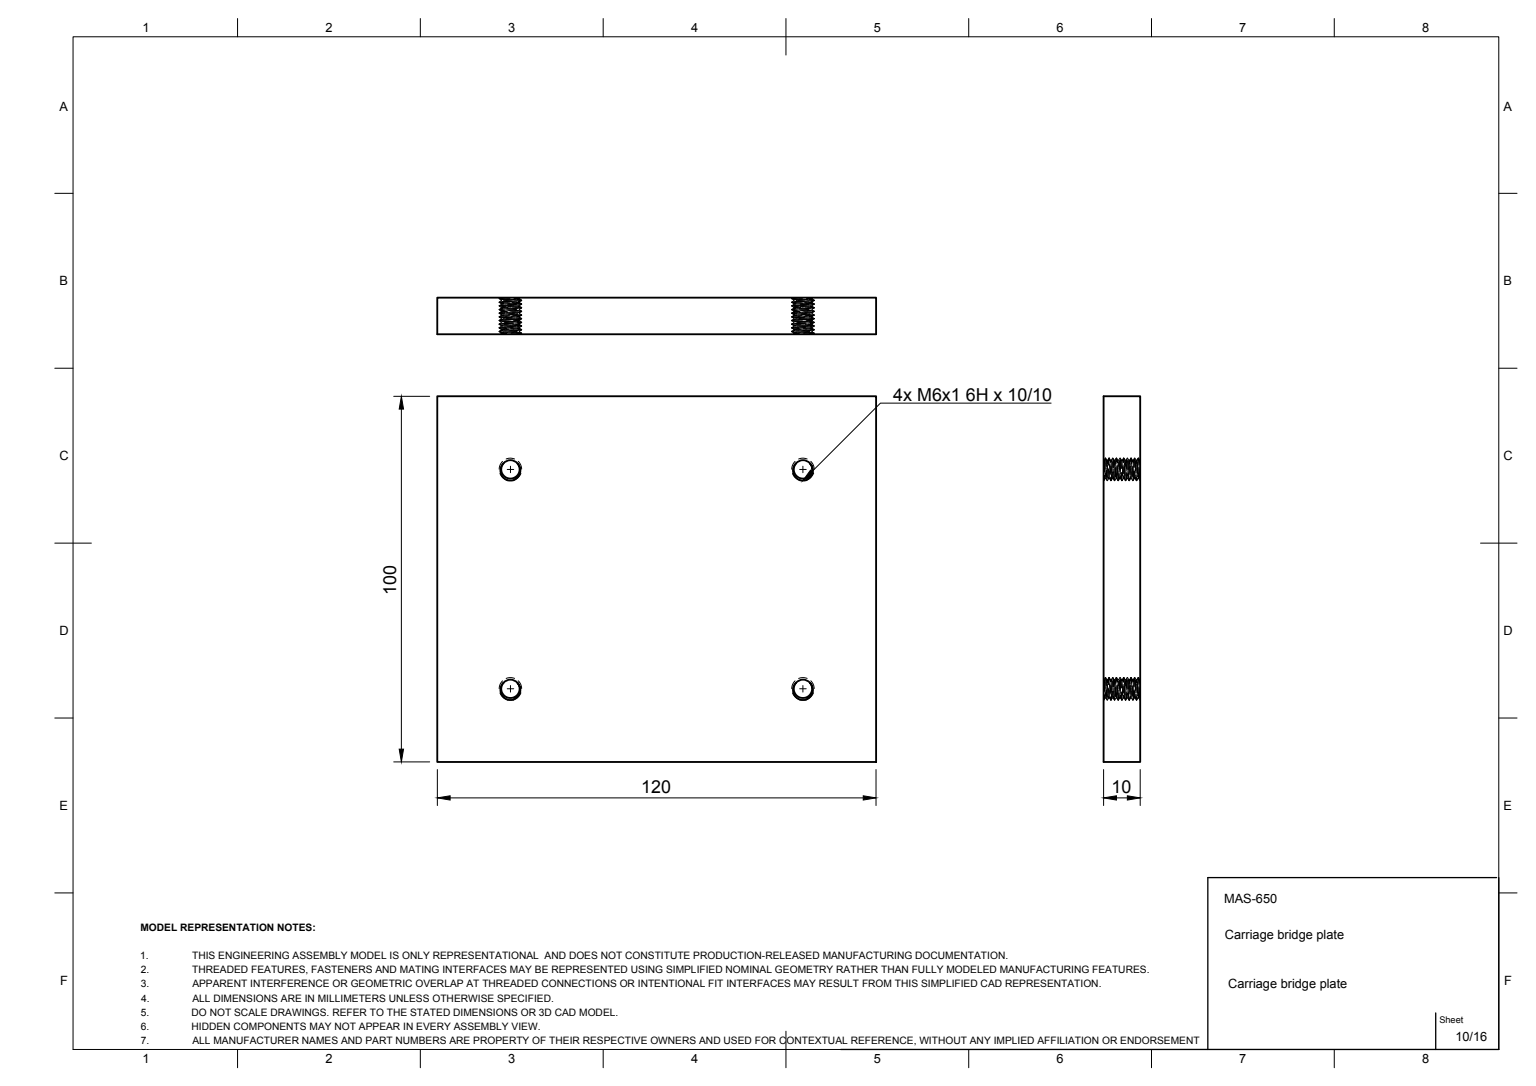
ISO-10303-21;
HEADER;
/* Generated by software containing ST-Developer
 * from STEP Tools, Inc. (www.steptools.com) 
 */

FILE_DESCRIPTION(
/* description */ ('Independent manual traversing gantry with native reusable aluminum pr
ofiles,180mm captured carriage travel, four bronze-bushed rollers, lin
ked ideal rolling motion, bonded acetal lateral guides, positive welde
d end stops and fully retained axle stacks. Editable native profile cu
t lengths220/400mm. Tool attachments viaM6 bridge-plate taps; mounted 
tool outside assembly. Welds, anchors, adhesives, fits, traction, load
/speed/structural/life ratings unassigned.'),
/* implementation_level */ '2;1');

FILE_NAME(
/* name */ 'Carriage bridge plate.step',
/* time_stamp */ '2026-11-09T20:04:38-08:00',
/* author */ (''),
/* organization */ (''),
/* preprocessor_version */ 'ST-DEVELOPER v20.2',
/* originating_system */ 'Autodesk Translation Framework v15.17.0.0',
/* authorisation */ '');

FILE_SCHEMA (('AUTOMOTIVE_DESIGN { 1 0 10303 214 3 1 1 }'));
ENDSEC;

DATA;
#10=MECHANICAL_DESIGN_GEOMETRIC_PRESENTATION_REPRESENTATION('',(#478),#13231);
#239=B_SPLINE_SURFACE_WITH_KNOTS('',3,3,((#8992,#8993,#8994,#8995,#8996,
#8997,#8998,#8999,#9000,#9001,#9002,#9003,#9004,#9005,#9006,#9007,#9008,
#9009,#9010,#9011,#9012,#9013,#9014,#9015,#9016,#9017,#9018,#9019,#9020,
#9021,#9022,#9023,#9024,#9025,#9026,#9027,#9028,#9029,#9030,#9031,#9032,
#9033,#9034,#9035,#9036,#9037,#9038,#9039,#9040,#9041,#9042,#9043,#9044,
#9045,#9046,#9047,#9048,#9049,#9050,#9051,#9052,#9053,#9054,#9055,#9056,
#9057,#9058,#9059),(#9060,#9061,#9062,#9063,#9064,#9065,#9066,#9067,#9068,
#9069,#9070,#9071,#9072,#9073,#9074,#9075,#9076,#9077,#9078,#9079,#9080,
#9081,#9082,#9083,#9084,#9085,#9086,#9087,#9088,#9089,#9090,#9091,#9092,
#9093,#9094,#9095,#9096,#9097,#9098,#9099,#9100,#9101,#9102,#9103,#9104,
#9105,#9106,#9107,#9108,#9109,#9110,#9111,#9112,#9113,#9114,#9115,#9116,
#9117,#9118,#9119,#9120,#9121,#9122,#9123,#9124,#9125,#9126,#9127),(#9128,
#9129,#9130,#9131,#9132,#9133,#9134,#9135,#9136,#9137,#9138,#9139,#9140,
#9141,#9142,#9143,#9144,#9145,#9146,#9147,#9148,#9149,#9150,#9151,#9152,
#9153,#9154,#9155,#9156,#9157,#9158,#9159,#9160,#9161,#9162,#9163,#9164,
#9165,#9166,#9167,#9168,#9169,#9170,#9171,#9172,#9173,#9174,#9175,#9176,
#9177,#9178,#9179,#9180,#9181,#9182,#9183,#9184,#9185,#9186,#9187,#9188,
#9189,#9190,#9191,#9192,#9193,#9194,#9195),(#9196,#9197,#9198,#9199,#9200,
#9201,#9202,#9203,#9204,#9205,#9206,#9207,#9208,#9209,#9210,#9211,#9212,
#9213,#9214,#9215,#9216,#9217,#9218,#9219,#9220,#9221,#9222,#9223,#9224,
#9225,#9226,#9227,#9228,#9229,#9230,#9231,#9232,#9233,#9234,#9235,#9236,
#9237,#9238,#9239,#9240,#9241,#9242,#9243,#9244,#9245,#9246,#9247,#9248,
#9249,#9250,#9251,#9252,#9253,#9254,#9255,#9256,#9257,#9258,#9259,#9260,
#9261,#9262,#9263)),.UNSPECIFIED.,.F.,.F.,.F.,(4,4),(4,1,1,1,1,1,1,1,1,
1,1,1,1,1,1,1,1,1,1,1,1,1,1,1,1,1,1,1,1,1,1,1,1,1,1,1,1,1,1,1,1,1,1,1,1,
1,1,1,1,1,1,1,1,1,1,1,1,1,1,1,1,1,1,1,1,4),(0.,0.0642013499338865),(11.8589888623078,
12.8566626771512,13.8543364919947,14.8520103068381,15.8496841216816,16.8473579365251,
17.8450317513685,18.842705566212,19.8403793810554,20.8380531958989,21.8357270107423,
22.8334008255858,23.8310746404292,24.8287484552727,25.8264222701161,26.8240960849596,
27.821769899803,28.8194437146465,29.8171175294899,30.8147913443334,31.8124651591768,
32.8101389740203,33.8078127888637,34.8054866037072,35.8031604185506,36.8008342333941,
37.7985080482375,38.796181863081,39.7938556779244,40.7915294927679,41.7892033076113,
42.7868771224548,43.7845509372982,44.7822247521417,45.7798985669851,46.7775723818286,
47.775246196672,48.7729200115155,49.7705938263589,50.7682676412024,51.7659414560458,
52.7636152708893,53.7612890857327,54.7589629005762,55.7566367154196,56.7543105302631,
57.7519843451065,58.74965815995,59.7473319747934,60.7450057896369,61.7426796044803,
62.7403534193238,63.7380272341672,64.7357010490107,65.7333748638542,66.7310486786976,
67.728722493541,68.7263963083845,69.7240701232279,70.7217439380714,71.7194177529149,
72.7170915677583,73.7147653826018,74.7124391974452,75.7101130122887,76.7077868271321),
 .UNSPECIFIED.);
#240=B_SPLINE_SURFACE_WITH_KNOTS('',3,3,((#9480,#9481,#9482,#9483,#9484,
#9485,#9486,#9487,#9488,#9489,#9490,#9491,#9492,#9493,#9494,#9495,#9496,
#9497,#9498,#9499,#9500,#9501,#9502,#9503,#9504,#9505,#9506,#9507,#9508,
#9509,#9510,#9511,#9512,#9513,#9514,#9515,#9516,#9517,#9518,#9519,#9520,
#9521,#9522,#9523,#9524,#9525,#9526,#9527,#9528,#9529,#9530,#9531,#9532,
#9533,#9534,#9535,#9536,#9537,#9538,#9539,#9540,#9541,#9542,#9543,#9544,
#9545,#9546,#9547),(#9548,#9549,#9550,#9551,#9552,#9553,#9554,#9555,#9556,
#9557,#9558,#9559,#9560,#9561,#9562,#9563,#9564,#9565,#9566,#9567,#9568,
#9569,#9570,#9571,#9572,#9573,#9574,#9575,#9576,#9577,#9578,#9579,#9580,
#9581,#9582,#9583,#9584,#9585,#9586,#9587,#9588,#9589,#9590,#9591,#9592,
#9593,#9594,#9595,#9596,#9597,#9598,#9599,#9600,#9601,#9602,#9603,#9604,
#9605,#9606,#9607,#9608,#9609,#9610,#9611,#9612,#9613,#9614,#9615),(#9616,
#9617,#9618,#9619,#9620,#9621,#9622,#9623,#9624,#9625,#9626,#9627,#9628,
#9629,#9630,#9631,#9632,#9633,#9634,#9635,#9636,#9637,#9638,#9639,#9640,
#9641,#9642,#9643,#9644,#9645,#9646,#9647,#9648,#9649,#9650,#9651,#9652,
#9653,#9654,#9655,#9656,#9657,#9658,#9659,#9660,#9661,#9662,#9663,#9664,
#9665,#9666,#9667,#9668,#9669,#9670,#9671,#9672,#9673,#9674,#9675,#9676,
#9677,#9678,#9679,#9680,#9681,#9682,#9683),(#9684,#9685,#9686,#9687,#9688,
#9689,#9690,#9691,#9692,#9693,#9694,#9695,#9696,#9697,#9698,#9699,#9700,
#9701,#9702,#9703,#9704,#9705,#9706,#9707,#9708,#9709,#9710,#9711,#9712,
#9713,#9714,#9715,#9716,#9717,#9718,#9719,#9720,#9721,#9722,#9723,#9724,
#9725,#9726,#9727,#9728,#9729,#9730,#9731,#9732,#9733,#9734,#9735,#9736,
#9737,#9738,#9739,#9740,#9741,#9742,#9743,#9744,#9745,#9746,#9747,#9748,
#9749,#9750,#9751)),.UNSPECIFIED.,.F.,.F.,.F.,(4,4),(4,1,1,1,1,1,1,1,1,
1,1,1,1,1,1,1,1,1,1,1,1,1,1,1,1,1,1,1,1,1,1,1,1,1,1,1,1,1,1,1,1,1,1,1,1,
1,1,1,1,1,1,1,1,1,1,1,1,1,1,1,1,1,1,1,1,4),(0.,0.0642013499338865),(14.3984001269718,
15.3960739418153,16.3937477566587,17.3914215715022,18.3890953863456,19.3867692011891,
20.3844430160325,21.382116830876,22.3797906457194,23.3774644605629,24.3751382754063,
25.3728120902498,26.3704859050932,27.3681597199367,28.3658335347801,29.3635073496236,
30.361181164467,31.3588549793105,32.3565287941539,33.3542026089974,34.3518764238408,
35.3495502386843,36.3472240535278,37.3448978683712,38.3425716832147,39.3402454980581,
40.3379193129016,41.335593127745,42.3332669425885,43.3309407574319,44.3286145722754,
45.3262883871188,46.3239622019623,47.3216360168057,48.3193098316492,49.3169836464926,
50.3146574613361,51.3123312761795,52.310005091023,53.3076789058664,54.3053527207099,
55.3030265355533,56.3007003503968,57.2983741652402,58.2960479800837,59.2937217949271,
60.2913956097706,61.289069424614,62.2867432394575,63.2844170543009,64.2820908691444,
65.2797646839878,66.2774384988313,67.2751123136747,68.2727861285182,69.2704599433616,
70.2681337582051,71.2658075730485,72.263481387892,73.2611552027354,74.2588290175789,
75.2565028324223,76.2541766472658,77.2518504621092,78.2495242769527,79.2471980917962),
 .UNSPECIFIED.);
#241=B_SPLINE_SURFACE_WITH_KNOTS('',3,3,((#10569,#10570,#10571,#10572,#10573,
#10574,#10575,#10576,#10577,#10578,#10579,#10580,#10581,#10582,#10583,#10584,
#10585,#10586,#10587,#10588,#10589,#10590,#10591,#10592,#10593,#10594,#10595,
#10596,#10597,#10598,#10599,#10600,#10601,#10602,#10603,#10604,#10605,#10606,
#10607,#10608,#10609,#10610,#10611,#10612,#10613,#10614,#10615,#10616,#10617,
#10618,#10619,#10620,#10621,#10622,#10623,#10624,#10625,#10626,#10627,#10628,
#10629,#10630,#10631,#10632,#10633,#10634,#10635,#10636),(#10637,#10638,
#10639,#10640,#10641,#10642,#10643,#10644,#10645,#10646,#10647,#10648,#10649,
#10650,#10651,#10652,#10653,#10654,#10655,#10656,#10657,#10658,#10659,#10660,
#10661,#10662,#10663,#10664,#10665,#10666,#10667,#10668,#10669,#10670,#10671,
#10672,#10673,#10674,#10675,#10676,#10677,#10678,#10679,#10680,#10681,#10682,
#10683,#10684,#10685,#10686,#10687,#10688,#10689,#10690,#10691,#10692,#10693,
#10694,#10695,#10696,#10697,#10698,#10699,#10700,#10701,#10702,#10703,#10704),
(#10705,#10706,#10707,#10708,#10709,#10710,#10711,#10712,#10713,#10714,
#10715,#10716,#10717,#10718,#10719,#10720,#10721,#10722,#10723,#10724,#10725,
#10726,#10727,#10728,#10729,#10730,#10731,#10732,#10733,#10734,#10735,#10736,
#10737,#10738,#10739,#10740,#10741,#10742,#10743,#10744,#10745,#10746,#10747,
#10748,#10749,#10750,#10751,#10752,#10753,#10754,#10755,#10756,#10757,#10758,
#10759,#10760,#10761,#10762,#10763,#10764,#10765,#10766,#10767,#10768,#10769,
#10770,#10771,#10772),(#10773,#10774,#10775,#10776,#10777,#10778,#10779,
#10780,#10781,#10782,#10783,#10784,#10785,#10786,#10787,#10788,#10789,#10790,
#10791,#10792,#10793,#10794,#10795,#10796,#10797,#10798,#10799,#10800,#10801,
#10802,#10803,#10804,#10805,#10806,#10807,#10808,#10809,#10810,#10811,#10812,
#10813,#10814,#10815,#10816,#10817,#10818,#10819,#10820,#10821,#10822,#10823,
#10824,#10825,#10826,#10827,#10828,#10829,#10830,#10831,#10832,#10833,#10834,
#10835,#10836,#10837,#10838,#10839,#10840)),.UNSPECIFIED.,.F.,.F.,.F.,(4,
4),(4,1,1,1,1,1,1,1,1,1,1,1,1,1,1,1,1,1,1,1,1,1,1,1,1,1,1,1,1,1,1,1,1,1,
1,1,1,1,1,1,1,1,1,1,1,1,1,1,1,1,1,1,1,1,1,1,1,1,1,1,1,1,1,1,1,4),(0.,0.0642013499338865),
(11.8589888623078,12.8566626771512,13.8543364919947,14.8520103068381,15.8496841216816,
16.847357936525,17.8450317513685,18.8427055662119,19.8403793810554,20.8380531958989,
21.8357270107423,22.8334008255858,23.8310746404292,24.8287484552727,25.8264222701161,
26.8240960849596,27.821769899803,28.8194437146465,29.8171175294899,30.8147913443334,
31.8124651591768,32.8101389740203,33.8078127888637,34.8054866037072,35.8031604185506,
36.8008342333941,37.7985080482375,38.796181863081,39.7938556779244,40.7915294927679,
41.7892033076113,42.7868771224548,43.7845509372982,44.7822247521417,45.7798985669851,
46.7775723818286,47.775246196672,48.7729200115155,49.7705938263589,50.7682676412024,
51.7659414560458,52.7636152708893,53.7612890857327,54.7589629005762,55.7566367154196,
56.7543105302631,57.7519843451065,58.74965815995,59.7473319747934,60.7450057896369,
61.7426796044803,62.7403534193238,63.7380272341672,64.7357010490107,65.7333748638542,
66.7310486786976,67.728722493541,68.7263963083845,69.7240701232279,70.7217439380714,
71.7194177529149,72.7170915677583,73.7147653826018,74.7124391974452,75.7101130122887,
76.7077868271321),.UNSPECIFIED.);
#242=B_SPLINE_SURFACE_WITH_KNOTS('',3,3,((#10960,#10961,#10962,#10963,#10964,
#10965,#10966,#10967,#10968,#10969,#10970,#10971,#10972,#10973,#10974,#10975,
#10976,#10977,#10978,#10979,#10980,#10981,#10982,#10983,#10984,#10985,#10986,
#10987,#10988,#10989,#10990,#10991,#10992,#10993,#10994,#10995,#10996,#10997,
#10998,#10999,#11000,#11001,#11002,#11003,#11004,#11005,#11006,#11007,#11008,
#11009,#11010,#11011,#11012,#11013,#11014,#11015,#11016,#11017,#11018,#11019,
#11020,#11021,#11022,#11023,#11024,#11025,#11026,#11027),(#11028,#11029,
#11030,#11031,#11032,#11033,#11034,#11035,#11036,#11037,#11038,#11039,#11040,
#11041,#11042,#11043,#11044,#11045,#11046,#11047,#11048,#11049,#11050,#11051,
#11052,#11053,#11054,#11055,#11056,#11057,#11058,#11059,#11060,#11061,#11062,
#11063,#11064,#11065,#11066,#11067,#11068,#11069,#11070,#11071,#11072,#11073,
#11074,#11075,#11076,#11077,#11078,#11079,#11080,#11081,#11082,#11083,#11084,
#11085,#11086,#11087,#11088,#11089,#11090,#11091,#11092,#11093,#11094,#11095),
(#11096,#11097,#11098,#11099,#11100,#11101,#11102,#11103,#11104,#11105,
#11106,#11107,#11108,#11109,#11110,#11111,#11112,#11113,#11114,#11115,#11116,
#11117,#11118,#11119,#11120,#11121,#11122,#11123,#11124,#11125,#11126,#11127,
#11128,#11129,#11130,#11131,#11132,#11133,#11134,#11135,#11136,#11137,#11138,
#11139,#11140,#11141,#11142,#11143,#11144,#11145,#11146,#11147,#11148,#11149,
#11150,#11151,#11152,#11153,#11154,#11155,#11156,#11157,#11158,#11159,#11160,
#11161,#11162,#11163),(#11164,#11165,#11166,#11167,#11168,#11169,#11170,
#11171,#11172,#11173,#11174,#11175,#11176,#11177,#11178,#11179,#11180,#11181,
#11182,#11183,#11184,#11185,#11186,#11187,#11188,#11189,#11190,#11191,#11192,
#11193,#11194,#11195,#11196,#11197,#11198,#11199,#11200,#11201,#11202,#11203,
#11204,#11205,#11206,#11207,#11208,#11209,#11210,#11211,#11212,#11213,#11214,
#11215,#11216,#11217,#11218,#11219,#11220,#11221,#11222,#11223,#11224,#11225,
#11226,#11227,#11228,#11229,#11230,#11231)),.UNSPECIFIED.,.F.,.F.,.F.,(4,
4),(4,1,1,1,1,1,1,1,1,1,1,1,1,1,1,1,1,1,1,1,1,1,1,1,1,1,1,1,1,1,1,1,1,1,
1,1,1,1,1,1,1,1,1,1,1,1,1,1,1,1,1,1,1,1,1,1,1,1,1,1,1,1,1,1,1,4),(0.,0.0642013499338865),
(14.3984001269718,15.3960739418153,16.3937477566587,17.3914215715022,18.3890953863456,
19.3867692011891,20.3844430160325,21.382116830876,22.3797906457194,23.3774644605629,
24.3751382754063,25.3728120902498,26.3704859050932,27.3681597199367,28.3658335347801,
29.3635073496236,30.361181164467,31.3588549793105,32.3565287941539,33.3542026089974,
34.3518764238408,35.3495502386843,36.3472240535278,37.3448978683712,38.3425716832147,
39.3402454980581,40.3379193129016,41.335593127745,42.3332669425885,43.3309407574319,
44.3286145722754,45.3262883871188,46.3239622019623,47.3216360168057,48.3193098316492,
49.3169836464926,50.3146574613361,51.3123312761795,52.310005091023,53.3076789058664,
54.3053527207099,55.3030265355533,56.3007003503968,57.2983741652402,58.2960479800837,
59.2937217949271,60.2913956097706,61.289069424614,62.2867432394575,63.2844170543009,
64.2820908691444,65.2797646839878,66.2774384988313,67.2751123136747,68.2727861285182,
69.2704599433616,70.2681337582051,71.2658075730485,72.263481387892,73.2611552027354,
74.2588290175789,75.2565028324223,76.2541766472658,77.2518504621092,78.2495242769527,
79.2471980917962),.UNSPECIFIED.);
#243=B_SPLINE_SURFACE_WITH_KNOTS('',3,3,((#11373,#11374,#11375,#11376,#11377,
#11378,#11379,#11380,#11381,#11382,#11383,#11384,#11385,#11386,#11387,#11388,
#11389,#11390,#11391,#11392,#11393,#11394,#11395,#11396,#11397,#11398,#11399,
#11400,#11401,#11402,#11403,#11404,#11405,#11406,#11407,#11408,#11409,#11410,
#11411,#11412,#11413,#11414,#11415,#11416,#11417,#11418,#11419,#11420,#11421,
#11422,#11423,#11424,#11425,#11426,#11427,#11428,#11429,#11430,#11431,#11432,
#11433,#11434,#11435,#11436,#11437,#11438,#11439,#11440),(#11441,#11442,
#11443,#11444,#11445,#11446,#11447,#11448,#11449,#11450,#11451,#11452,#11453,
#11454,#11455,#11456,#11457,#11458,#11459,#11460,#11461,#11462,#11463,#11464,
#11465,#11466,#11467,#11468,#11469,#11470,#11471,#11472,#11473,#11474,#11475,
#11476,#11477,#11478,#11479,#11480,#11481,#11482,#11483,#11484,#11485,#11486,
#11487,#11488,#11489,#11490,#11491,#11492,#11493,#11494,#11495,#11496,#11497,
#11498,#11499,#11500,#11501,#11502,#11503,#11504,#11505,#11506,#11507,#11508),
(#11509,#11510,#11511,#11512,#11513,#11514,#11515,#11516,#11517,#11518,
#11519,#11520,#11521,#11522,#11523,#11524,#11525,#11526,#11527,#11528,#11529,
#11530,#11531,#11532,#11533,#11534,#11535,#11536,#11537,#11538,#11539,#11540,
#11541,#11542,#11543,#11544,#11545,#11546,#11547,#11548,#11549,#11550,#11551,
#11552,#11553,#11554,#11555,#11556,#11557,#11558,#11559,#11560,#11561,#11562,
#11563,#11564,#11565,#11566,#11567,#11568,#11569,#11570,#11571,#11572,#11573,
#11574,#11575,#11576),(#11577,#11578,#11579,#11580,#11581,#11582,#11583,
#11584,#11585,#11586,#11587,#11588,#11589,#11590,#11591,#11592,#11593,#11594,
#11595,#11596,#11597,#11598,#11599,#11600,#11601,#11602,#11603,#11604,#11605,
#11606,#11607,#11608,#11609,#11610,#11611,#11612,#11613,#11614,#11615,#11616,
#11617,#11618,#11619,#11620,#11621,#11622,#11623,#11624,#11625,#11626,#11627,
#11628,#11629,#11630,#11631,#11632,#11633,#11634,#11635,#11636,#11637,#11638,
#11639,#11640,#11641,#11642,#11643,#11644)),.UNSPECIFIED.,.F.,.F.,.F.,(4,
4),(4,1,1,1,1,1,1,1,1,1,1,1,1,1,1,1,1,1,1,1,1,1,1,1,1,1,1,1,1,1,1,1,1,1,
1,1,1,1,1,1,1,1,1,1,1,1,1,1,1,1,1,1,1,1,1,1,1,1,1,1,1,1,1,1,1,4),(0.,0.0642013499338865),
(11.8589888623078,12.8566626771512,13.8543364919947,14.8520103068381,15.8496841216816,
16.847357936525,17.8450317513685,18.8427055662119,19.8403793810554,20.8380531958988,
21.8357270107423,22.8334008255857,23.8310746404292,24.8287484552726,25.8264222701161,
26.8240960849595,27.821769899803,28.8194437146464,29.8171175294899,30.8147913443333,
31.8124651591768,32.8101389740202,33.8078127888637,34.8054866037072,35.8031604185506,
36.8008342333941,37.7985080482375,38.796181863081,39.7938556779244,40.7915294927679,
41.7892033076113,42.7868771224548,43.7845509372982,44.7822247521417,45.7798985669851,
46.7775723818286,47.775246196672,48.7729200115155,49.7705938263589,50.7682676412024,
51.7659414560458,52.7636152708893,53.7612890857327,54.7589629005762,55.7566367154196,
56.7543105302631,57.7519843451065,58.74965815995,59.7473319747934,60.7450057896369,
61.7426796044803,62.7403534193238,63.7380272341672,64.7357010490107,65.7333748638541,
66.7310486786976,67.728722493541,68.7263963083845,69.7240701232279,70.7217439380714,
71.7194177529148,72.7170915677583,73.7147653826017,74.7124391974452,75.7101130122886,
76.7077868271321),.UNSPECIFIED.);
#244=B_SPLINE_SURFACE_WITH_KNOTS('',3,3,((#11764,#11765,#11766,#11767,#11768,
#11769,#11770,#11771,#11772,#11773,#11774,#11775,#11776,#11777,#11778,#11779,
#11780,#11781,#11782,#11783,#11784,#11785,#11786,#11787,#11788,#11789,#11790,
#11791,#11792,#11793,#11794,#11795,#11796,#11797,#11798,#11799,#11800,#11801,
#11802,#11803,#11804,#11805,#11806,#11807,#11808,#11809,#11810,#11811,#11812,
#11813,#11814,#11815,#11816,#11817,#11818,#11819,#11820,#11821,#11822,#11823,
#11824,#11825,#11826,#11827,#11828,#11829,#11830,#11831),(#11832,#11833,
#11834,#11835,#11836,#11837,#11838,#11839,#11840,#11841,#11842,#11843,#11844,
#11845,#11846,#11847,#11848,#11849,#11850,#11851,#11852,#11853,#11854,#11855,
#11856,#11857,#11858,#11859,#11860,#11861,#11862,#11863,#11864,#11865,#11866,
#11867,#11868,#11869,#11870,#11871,#11872,#11873,#11874,#11875,#11876,#11877,
#11878,#11879,#11880,#11881,#11882,#11883,#11884,#11885,#11886,#11887,#11888,
#11889,#11890,#11891,#11892,#11893,#11894,#11895,#11896,#11897,#11898,#11899),
(#11900,#11901,#11902,#11903,#11904,#11905,#11906,#11907,#11908,#11909,
#11910,#11911,#11912,#11913,#11914,#11915,#11916,#11917,#11918,#11919,#11920,
#11921,#11922,#11923,#11924,#11925,#11926,#11927,#11928,#11929,#11930,#11931,
#11932,#11933,#11934,#11935,#11936,#11937,#11938,#11939,#11940,#11941,#11942,
#11943,#11944,#11945,#11946,#11947,#11948,#11949,#11950,#11951,#11952,#11953,
#11954,#11955,#11956,#11957,#11958,#11959,#11960,#11961,#11962,#11963,#11964,
#11965,#11966,#11967),(#11968,#11969,#11970,#11971,#11972,#11973,#11974,
#11975,#11976,#11977,#11978,#11979,#11980,#11981,#11982,#11983,#11984,#11985,
#11986,#11987,#11988,#11989,#11990,#11991,#11992,#11993,#11994,#11995,#11996,
#11997,#11998,#11999,#12000,#12001,#12002,#12003,#12004,#12005,#12006,#12007,
#12008,#12009,#12010,#12011,#12012,#12013,#12014,#12015,#12016,#12017,#12018,
#12019,#12020,#12021,#12022,#12023,#12024,#12025,#12026,#12027,#12028,#12029,
#12030,#12031,#12032,#12033,#12034,#12035)),.UNSPECIFIED.,.F.,.F.,.F.,(4,
4),(4,1,1,1,1,1,1,1,1,1,1,1,1,1,1,1,1,1,1,1,1,1,1,1,1,1,1,1,1,1,1,1,1,1,
1,1,1,1,1,1,1,1,1,1,1,1,1,1,1,1,1,1,1,1,1,1,1,1,1,1,1,1,1,1,1,4),(0.,0.0642013499338865),
(14.3984001269718,15.3960739418153,16.3937477566587,17.3914215715022,18.3890953863456,
19.3867692011891,20.3844430160325,21.382116830876,22.3797906457194,23.3774644605629,
24.3751382754063,25.3728120902498,26.3704859050932,27.3681597199367,28.3658335347801,
29.3635073496236,30.361181164467,31.3588549793105,32.3565287941539,33.3542026089974,
34.3518764238408,35.3495502386843,36.3472240535277,37.3448978683712,38.3425716832146,
39.3402454980581,40.3379193129015,41.335593127745,42.3332669425884,43.3309407574319,
44.3286145722753,45.3262883871188,46.3239622019622,47.3216360168057,48.3193098316492,
49.3169836464926,50.3146574613361,51.3123312761795,52.310005091023,53.3076789058664,
54.3053527207099,55.3030265355533,56.3007003503968,57.2983741652402,58.2960479800837,
59.2937217949271,60.2913956097706,61.289069424614,62.2867432394575,63.2844170543009,
64.2820908691444,65.2797646839878,66.2774384988313,67.2751123136747,68.2727861285182,
69.2704599433616,70.2681337582051,71.2658075730485,72.263481387892,73.2611552027354,
74.2588290175789,75.2565028324223,76.2541766472658,77.2518504621092,78.2495242769527,
79.2471980917961),.UNSPECIFIED.);
#245=B_SPLINE_SURFACE_WITH_KNOTS('',3,3,((#12177,#12178,#12179,#12180,#12181,
#12182,#12183,#12184,#12185,#12186,#12187,#12188,#12189,#12190,#12191,#12192,
#12193,#12194,#12195,#12196,#12197,#12198,#12199,#12200,#12201,#12202,#12203,
#12204,#12205,#12206,#12207,#12208,#12209,#12210,#12211,#12212,#12213,#12214,
#12215,#12216,#12217,#12218,#12219,#12220,#12221,#12222,#12223,#12224,#12225,
#12226,#12227,#12228,#12229,#12230,#12231,#12232,#12233,#12234,#12235,#12236,
#12237,#12238,#12239,#12240,#12241,#12242,#12243,#12244),(#12245,#12246,
#12247,#12248,#12249,#12250,#12251,#12252,#12253,#12254,#12255,#12256,#12257,
#12258,#12259,#12260,#12261,#12262,#12263,#12264,#12265,#12266,#12267,#12268,
#12269,#12270,#12271,#12272,#12273,#12274,#12275,#12276,#12277,#12278,#12279,
#12280,#12281,#12282,#12283,#12284,#12285,#12286,#12287,#12288,#12289,#12290,
#12291,#12292,#12293,#12294,#12295,#12296,#12297,#12298,#12299,#12300,#12301,
#12302,#12303,#12304,#12305,#12306,#12307,#12308,#12309,#12310,#12311,#12312),
(#12313,#12314,#12315,#12316,#12317,#12318,#12319,#12320,#12321,#12322,
#12323,#12324,#12325,#12326,#12327,#12328,#12329,#12330,#12331,#12332,#12333,
#12334,#12335,#12336,#12337,#12338,#12339,#12340,#12341,#12342,#12343,#12344,
#12345,#12346,#12347,#12348,#12349,#12350,#12351,#12352,#12353,#12354,#12355,
#12356,#12357,#12358,#12359,#12360,#12361,#12362,#12363,#12364,#12365,#12366,
#12367,#12368,#12369,#12370,#12371,#12372,#12373,#12374,#12375,#12376,#12377,
#12378,#12379,#12380),(#12381,#12382,#12383,#12384,#12385,#12386,#12387,
#12388,#12389,#12390,#12391,#12392,#12393,#12394,#12395,#12396,#12397,#12398,
#12399,#12400,#12401,#12402,#12403,#12404,#12405,#12406,#12407,#12408,#12409,
#12410,#12411,#12412,#12413,#12414,#12415,#12416,#12417,#12418,#12419,#12420,
#12421,#12422,#12423,#12424,#12425,#12426,#12427,#12428,#12429,#12430,#12431,
#12432,#12433,#12434,#12435,#12436,#12437,#12438,#12439,#12440,#12441,#12442,
#12443,#12444,#12445,#12446,#12447,#12448)),.UNSPECIFIED.,.F.,.F.,.F.,(4,
4),(4,1,1,1,1,1,1,1,1,1,1,1,1,1,1,1,1,1,1,1,1,1,1,1,1,1,1,1,1,1,1,1,1,1,
1,1,1,1,1,1,1,1,1,1,1,1,1,1,1,1,1,1,1,1,1,1,1,1,1,1,1,1,1,1,1,4),(0.,0.0642013499338865),
(11.8589888623078,12.8566626771512,13.8543364919947,14.8520103068381,15.8496841216816,
16.8473579365251,17.8450317513685,18.842705566212,19.8403793810554,20.8380531958989,
21.8357270107423,22.8334008255858,23.8310746404292,24.8287484552727,25.8264222701161,
26.8240960849596,27.821769899803,28.8194437146465,29.8171175294899,30.8147913443334,
31.8124651591768,32.8101389740203,33.8078127888637,34.8054866037072,35.8031604185506,
36.8008342333941,37.7985080482375,38.796181863081,39.7938556779244,40.7915294927679,
41.7892033076113,42.7868771224548,43.7845509372982,44.7822247521417,45.7798985669851,
46.7775723818286,47.775246196672,48.7729200115155,49.7705938263589,50.7682676412024,
51.7659414560458,52.7636152708893,53.7612890857327,54.7589629005762,55.7566367154196,
56.7543105302631,57.7519843451065,58.74965815995,59.7473319747934,60.7450057896369,
61.7426796044803,62.7403534193238,63.7380272341672,64.7357010490107,65.7333748638542,
66.7310486786976,67.728722493541,68.7263963083845,69.7240701232279,70.7217439380714,
71.7194177529149,72.7170915677583,73.7147653826018,74.7124391974452,75.7101130122887,
76.7077868271321),.UNSPECIFIED.);
#246=B_SPLINE_SURFACE_WITH_KNOTS('',3,3,((#12568,#12569,#12570,#12571,#12572,
#12573,#12574,#12575,#12576,#12577,#12578,#12579,#12580,#12581,#12582,#12583,
#12584,#12585,#12586,#12587,#12588,#12589,#12590,#12591,#12592,#12593,#12594,
#12595,#12596,#12597,#12598,#12599,#12600,#12601,#12602,#12603,#12604,#12605,
#12606,#12607,#12608,#12609,#12610,#12611,#12612,#12613,#12614,#12615,#12616,
#12617,#12618,#12619,#12620,#12621,#12622,#12623,#12624,#12625,#12626,#12627,
#12628,#12629,#12630,#12631,#12632,#12633,#12634,#12635),(#12636,#12637,
#12638,#12639,#12640,#12641,#12642,#12643,#12644,#12645,#12646,#12647,#12648,
#12649,#12650,#12651,#12652,#12653,#12654,#12655,#12656,#12657,#12658,#12659,
#12660,#12661,#12662,#12663,#12664,#12665,#12666,#12667,#12668,#12669,#12670,
#12671,#12672,#12673,#12674,#12675,#12676,#12677,#12678,#12679,#12680,#12681,
#12682,#12683,#12684,#12685,#12686,#12687,#12688,#12689,#12690,#12691,#12692,
#12693,#12694,#12695,#12696,#12697,#12698,#12699,#12700,#12701,#12702,#12703),
(#12704,#12705,#12706,#12707,#12708,#12709,#12710,#12711,#12712,#12713,
#12714,#12715,#12716,#12717,#12718,#12719,#12720,#12721,#12722,#12723,#12724,
#12725,#12726,#12727,#12728,#12729,#12730,#12731,#12732,#12733,#12734,#12735,
#12736,#12737,#12738,#12739,#12740,#12741,#12742,#12743,#12744,#12745,#12746,
#12747,#12748,#12749,#12750,#12751,#12752,#12753,#12754,#12755,#12756,#12757,
#12758,#12759,#12760,#12761,#12762,#12763,#12764,#12765,#12766,#12767,#12768,
#12769,#12770,#12771),(#12772,#12773,#12774,#12775,#12776,#12777,#12778,
#12779,#12780,#12781,#12782,#12783,#12784,#12785,#12786,#12787,#12788,#12789,
#12790,#12791,#12792,#12793,#12794,#12795,#12796,#12797,#12798,#12799,#12800,
#12801,#12802,#12803,#12804,#12805,#12806,#12807,#12808,#12809,#12810,#12811,
#12812,#12813,#12814,#12815,#12816,#12817,#12818,#12819,#12820,#12821,#12822,
#12823,#12824,#12825,#12826,#12827,#12828,#12829,#12830,#12831,#12832,#12833,
#12834,#12835,#12836,#12837,#12838,#12839)),.UNSPECIFIED.,.F.,.F.,.F.,(4,
4),(4,1,1,1,1,1,1,1,1,1,1,1,1,1,1,1,1,1,1,1,1,1,1,1,1,1,1,1,1,1,1,1,1,1,
1,1,1,1,1,1,1,1,1,1,1,1,1,1,1,1,1,1,1,1,1,1,1,1,1,1,1,1,1,1,1,4),(0.,0.0642013499338865),
(14.3984001269718,15.3960739418153,16.3937477566587,17.3914215715022,18.3890953863456,
19.3867692011891,20.3844430160325,21.382116830876,22.3797906457194,23.3774644605629,
24.3751382754063,25.3728120902498,26.3704859050932,27.3681597199367,28.3658335347801,
29.3635073496236,30.361181164467,31.3588549793105,32.3565287941539,33.3542026089974,
34.3518764238408,35.3495502386843,36.3472240535278,37.3448978683712,38.3425716832147,
39.3402454980581,40.3379193129016,41.335593127745,42.3332669425885,43.3309407574319,
44.3286145722754,45.3262883871188,46.3239622019623,47.3216360168057,48.3193098316492,
49.3169836464926,50.3146574613361,51.3123312761795,52.310005091023,53.3076789058664,
54.3053527207099,55.3030265355533,56.3007003503968,57.2983741652402,58.2960479800837,
59.2937217949271,60.2913956097706,61.289069424614,62.2867432394575,63.2844170543009,
64.2820908691444,65.2797646839878,66.2774384988313,67.2751123136747,68.2727861285182,
69.2704599433616,70.2681337582051,71.2658075730485,72.263481387892,73.2611552027354,
74.2588290175789,75.2565028324223,76.2541766472658,77.2518504621092,78.2495242769527,
79.2471980917962),.UNSPECIFIED.);
#247=B_SPLINE_CURVE_WITH_KNOTS('',3,(#6191,#6192,#6193,#6194),
 .UNSPECIFIED.,.F.,.F.,(4,4),(64.141416212773,64.8487979648243),
 .UNSPECIFIED.);
#248=B_SPLINE_CURVE_WITH_KNOTS('',3,(#6197,#6198,#6199,#6200,#6201,#6202,
#6203,#6204,#6205,#6206),.UNSPECIFIED.,.F.,.F.,(4,3,3,4),(-62.8318530717959,
-61.855776520294,-60.8581027054505,-60.3976421702574),.UNSPECIFIED.);
#249=B_SPLINE_CURVE_WITH_KNOTS('',3,(#6211,#6212,#6213,#6214,#6215,#6216,
#6217,#6218,#6219,#6220,#6221,#6222,#6223,#6224,#6225,#6226,#6227,#6228,
#6229,#6230,#6231,#6232,#6233,#6234,#6235),.UNSPECIFIED.,.F.,.F.,(4,3,3,
3,3,3,3,3,4),(57.8582309055934,57.8650812609202,58.8627550757636,59.8604288906071,
60.8581027054505,61.855776520294,62.8534503351374,63.8511241499809,64.141416212773),
 .UNSPECIFIED.);
#250=B_SPLINE_CURVE_WITH_KNOTS('',3,(#6236,#6237,#6238,#6239,#6240,#6241,
#6242,#6243,#6244,#6245,#6246,#6247,#6248,#6249,#6250,#6251,#6252,#6253,
#6254,#6255,#6256,#6257),.UNSPECIFIED.,.F.,.F.,(4,3,3,3,3,3,3,4),(-60.3976421702574,
-59.8604288906071,-58.8627550757636,-57.8650812609202,-56.8674074460767,
-55.8697336312333,-54.8720598163898,-54.1144568630778),.UNSPECIFIED.);
#251=B_SPLINE_CURVE_WITH_KNOTS('',3,(#6262,#6263,#6264,#6265,#6266,#6267,
#6268,#6269,#6270,#6271,#6272,#6273,#6274,#6275,#6276,#6277,#6278,#6279,
#6280,#6281,#6282,#6283),.UNSPECIFIED.,.F.,.F.,(4,3,3,3,3,3,3,4),(51.5750455984138,
51.8790383718595,52.8767121867029,53.8743860015464,54.8720598163898,55.8697336312333,
56.8674074460767,57.8582309055934),.UNSPECIFIED.);
#252=B_SPLINE_CURVE_WITH_KNOTS('',3,(#6284,#6285,#6286,#6287,#6288,#6289,
#6290,#6291,#6292,#6293,#6294,#6295,#6296,#6297,#6298,#6299,#6300,#6301,
#6302,#6303,#6304,#6305,#6306,#6307,#6308),.UNSPECIFIED.,.F.,.F.,(4,3,3,
3,3,3,3,3,4),(-54.1144568630778,-53.8743860015464,-52.8767121867029,-51.8790383718595,
-50.881364557016,-49.8836907421726,-48.8860169273291,-47.8883431124856,
-47.8312715558982),.UNSPECIFIED.);
#253=B_SPLINE_CURVE_WITH_KNOTS('',3,(#6313,#6314,#6315,#6316,#6317,#6318,
#6319,#6320,#6321,#6322,#6323,#6324,#6325,#6326,#6327,#6328,#6329,#6330,
#6331,#6332,#6333,#6334),.UNSPECIFIED.,.F.,.F.,(4,3,3,3,3,3,3,4),(45.2918602912342,
45.8929954827987,46.8906692976422,47.8883431124856,48.8860169273291,49.8836907421726,
50.881364557016,51.5750455984138),.UNSPECIFIED.);
#254=B_SPLINE_CURVE_WITH_KNOTS('',3,(#6335,#6336,#6337,#6338,#6339,#6340,
#6341,#6342,#6343,#6344,#6345,#6346,#6347,#6348,#6349,#6350,#6351,#6352,
#6353,#6354,#6355,#6356),.UNSPECIFIED.,.F.,.F.,(4,3,3,3,3,3,3,4),(-47.8312715558982,
-46.8906692976422,-45.8929954827987,-44.8953216679553,-43.8976478531118,
-42.8999740382684,-41.9023002234249,-41.5480862487187),.UNSPECIFIED.);
#255=B_SPLINE_CURVE_WITH_KNOTS('',3,(#6361,#6362,#6363,#6364,#6365,#6366,
#6367,#6368,#6369,#6370,#6371,#6372,#6373,#6374,#6375,#6376,#6377,#6378,
#6379,#6380,#6381,#6382),.UNSPECIFIED.,.F.,.F.,(4,3,3,3,3,3,3,4),(39.0086749840546,
39.906952593738,40.9046264085815,41.9023002234249,42.8999740382684,43.8976478531118,
44.8953216679553,45.2918602912342),.UNSPECIFIED.);
#256=B_SPLINE_CURVE_WITH_KNOTS('',3,(#6383,#6384,#6385,#6386,#6387,#6388,
#6389,#6390,#6391,#6392,#6393,#6394,#6395,#6396,#6397,#6398,#6399,#6400,
#6401,#6402,#6403,#6404),.UNSPECIFIED.,.F.,.F.,(4,3,3,3,3,3,3,4),(-41.5480862487187,
-40.9046264085815,-39.906952593738,-38.9092787788946,-37.9116049640511,
-36.9139311492077,-35.9162573343642,-35.2649009415391),.UNSPECIFIED.);
#257=B_SPLINE_CURVE_WITH_KNOTS('',3,(#6409,#6410,#6411,#6412,#6413,#6414,
#6415,#6416,#6417,#6418,#6419,#6420,#6421,#6422,#6423,#6424,#6425,#6426,
#6427,#6428,#6429,#6430,#6431,#6432,#6433),.UNSPECIFIED.,.F.,.F.,(4,3,3,
3,3,3,3,3,4),(32.725489676875,32.9232358898339,33.9209097046773,34.9185835195208,
35.9162573343642,36.9139311492077,37.9116049640511,38.9092787788946,39.0086749840546),
 .UNSPECIFIED.);
#258=B_SPLINE_CURVE_WITH_KNOTS('',3,(#6434,#6435,#6436,#6437,#6438,#6439,
#6440,#6441,#6442,#6443,#6444,#6445,#6446,#6447,#6448,#6449,#6450,#6451,
#6452,#6453,#6454,#6455),.UNSPECIFIED.,.F.,.F.,(4,3,3,3,3,3,3,4),(-35.2649009415391,
-34.9185835195208,-33.9209097046773,-32.9232358898339,-31.9255620749904,
-30.927888260147,-29.9302144453035,-28.9817156343595),.UNSPECIFIED.);
#259=B_SPLINE_CURVE_WITH_KNOTS('',3,(#6460,#6461,#6462,#6463,#6464,#6465,
#6466,#6467,#6468,#6469,#6470,#6471,#6472,#6473,#6474,#6475,#6476,#6477,
#6478,#6479,#6480,#6481),.UNSPECIFIED.,.F.,.F.,(4,3,3,3,3,3,3,4),(26.4423043696954,
26.9371930007732,27.9348668156166,28.9325406304601,29.9302144453035,30.927888260147,
31.9255620749904,32.725489676875),.UNSPECIFIED.);
#260=B_SPLINE_CURVE_WITH_KNOTS('',3,(#6482,#6483,#6484,#6485,#6486,#6487,
#6488,#6489,#6490,#6491,#6492,#6493,#6494,#6495,#6496,#6497,#6498,#6499,
#6500,#6501,#6502,#6503,#6504,#6505,#6506),.UNSPECIFIED.,.F.,.F.,(4,3,3,
3,3,3,3,3,4),(-28.9817156343595,-28.9325406304601,-27.9348668156166,-26.9371930007732,
-25.9395191859297,-24.9418453710863,-23.9441715562428,-22.9464977413994,
-22.6985303271799),.UNSPECIFIED.);
#261=B_SPLINE_CURVE_WITH_KNOTS('',3,(#6511,#6512,#6513,#6514,#6515,#6516,
#6517,#6518,#6519,#6520,#6521,#6522,#6523,#6524,#6525,#6526,#6527,#6528,
#6529,#6530,#6531,#6532),.UNSPECIFIED.,.F.,.F.,(4,3,3,3,3,3,3,4),(20.1591190625158,
20.9511501117125,21.9488239265559,22.9464977413994,23.9441715562428,24.9418453710863,
25.9395191859297,26.4423043696954),.UNSPECIFIED.);
#262=B_SPLINE_CURVE_WITH_KNOTS('',3,(#6533,#6534,#6535,#6536,#6537,#6538,
#6539,#6540,#6541,#6542,#6543,#6544,#6545,#6546,#6547,#6548,#6549,#6550,
#6551,#6552,#6553,#6554),.UNSPECIFIED.,.F.,.F.,(4,3,3,3,3,3,3,4),(-22.6985303271799,
-21.9488239265559,-20.9511501117125,-19.953476296869,-18.9558024820256,
-17.9581286671821,-16.9604548523387,-16.4153450200003),.UNSPECIFIED.);
#263=B_SPLINE_CURVE_WITH_KNOTS('',3,(#6559,#6560,#6561,#6562,#6563,#6564,
#6565,#6566,#6567,#6568,#6569,#6570,#6571,#6572,#6573,#6574,#6575,#6576,
#6577,#6578,#6579,#6580,#6581,#6582,#6583),.UNSPECIFIED.,.F.,.F.,(4,3,3,
3,3,3,3,3,4),(13.8759337553362,13.9674334078083,14.9651072226518,15.9627810374952,
16.9604548523387,17.9581286671821,18.9558024820256,19.953476296869,20.1591190625158),
 .UNSPECIFIED.);
#264=B_SPLINE_CURVE_WITH_KNOTS('',3,(#6584,#6585,#6586,#6587,#6588,#6589,
#6590,#6591,#6592,#6593,#6594,#6595,#6596,#6597,#6598,#6599,#6600,#6601,
#6602,#6603,#6604,#6605),.UNSPECIFIED.,.F.,.F.,(4,3,3,3,3,3,3,4),(-16.4153450200003,
-15.9627810374952,-14.9651072226518,-13.9674334078083,-12.9697595929649,
-11.9720857781214,-10.974411963278,-10.1321597128207),.UNSPECIFIED.);
#265=B_SPLINE_CURVE_WITH_KNOTS('',3,(#6611,#6612,#6613,#6614,#6615,#6616,
#6617,#6618,#6619,#6620,#6621,#6622,#6623),.UNSPECIFIED.,.F.,.F.,(4,3,3,
3,4),(-3.84897440564113,-2.99302144453035,-1.99534762968691,-0.997673814843449,
0.),.UNSPECIFIED.);
#266=B_SPLINE_CURVE_WITH_KNOTS('',3,(#6626,#6627,#6628,#6629,#6630,#6631,
#6632,#6633,#6634,#6635,#6636,#6637,#6638,#6639,#6640,#6641,#6642,#6643,
#6644),.UNSPECIFIED.,.F.,.F.,(4,3,3,3,3,3,4),(2.01694489302844,2.99302144453035,
3.9906952593738,4.98836907421725,5.9860428890607,6.98371670390416,7.59274844815664),
 .UNSPECIFIED.);
#267=B_SPLINE_CURVE_WITH_KNOTS('',3,(#6650,#6651,#6652,#6653),
 .UNSPECIFIED.,.F.,.F.,(4,4),(64.141416212773,64.8487979648243),
 .UNSPECIFIED.);
#268=B_SPLINE_CURVE_WITH_KNOTS('',3,(#6656,#6657,#6658,#6659,#6660,#6661,
#6662,#6663,#6664,#6665),.UNSPECIFIED.,.F.,.F.,(4,3,3,4),(-62.8318530717958,
-61.855776520294,-60.8581027054505,-60.3976421702575),.UNSPECIFIED.);
#269=B_SPLINE_CURVE_WITH_KNOTS('',3,(#6670,#6671,#6672,#6673,#6674,#6675,
#6676,#6677,#6678,#6679,#6680,#6681,#6682,#6683,#6684,#6685,#6686,#6687,
#6688,#6689,#6690,#6691,#6692,#6693,#6694),.UNSPECIFIED.,.F.,.F.,(4,3,3,
3,3,3,3,3,4),(57.8582309055934,57.8650812609202,58.8627550757636,59.8604288906071,
60.8581027054505,61.855776520294,62.8534503351374,63.8511241499808,64.141416212773),
 .UNSPECIFIED.);
#270=B_SPLINE_CURVE_WITH_KNOTS('',3,(#6695,#6696,#6697,#6698,#6699,#6700,
#6701,#6702,#6703,#6704,#6705,#6706,#6707,#6708,#6709,#6710,#6711,#6712,
#6713,#6714,#6715,#6716),.UNSPECIFIED.,.F.,.F.,(4,3,3,3,3,3,3,4),(-60.3976421702575,
-59.8604288906071,-58.8627550757636,-57.8650812609201,-56.8674074460767,
-55.8697336312333,-54.8720598163898,-54.1144568630779),.UNSPECIFIED.);
#271=B_SPLINE_CURVE_WITH_KNOTS('',3,(#6721,#6722,#6723,#6724,#6725,#6726,
#6727,#6728,#6729,#6730,#6731,#6732,#6733,#6734,#6735,#6736,#6737,#6738,
#6739,#6740,#6741,#6742),.UNSPECIFIED.,.F.,.F.,(4,3,3,3,3,3,3,4),(51.5750455984138,
51.8790383718595,52.8767121867029,53.8743860015464,54.8720598163898,55.8697336312333,
56.8674074460767,57.8582309055934),.UNSPECIFIED.);
#272=B_SPLINE_CURVE_WITH_KNOTS('',3,(#6743,#6744,#6745,#6746,#6747,#6748,
#6749,#6750,#6751,#6752,#6753,#6754,#6755,#6756,#6757,#6758,#6759,#6760,
#6761,#6762,#6763,#6764,#6765,#6766,#6767),.UNSPECIFIED.,.F.,.F.,(4,3,3,
3,3,3,3,3,4),(-54.1144568630779,-53.8743860015464,-52.8767121867029,-51.8790383718595,
-50.881364557016,-49.8836907421726,-48.8860169273291,-47.8883431124857,
-47.8312715558983),.UNSPECIFIED.);
#273=B_SPLINE_CURVE_WITH_KNOTS('',3,(#6772,#6773,#6774,#6775,#6776,#6777,
#6778,#6779,#6780,#6781,#6782,#6783,#6784,#6785,#6786,#6787,#6788,#6789,
#6790,#6791,#6792,#6793),.UNSPECIFIED.,.F.,.F.,(4,3,3,3,3,3,3,4),(45.2918602912342,
45.8929954827987,46.8906692976422,47.8883431124857,48.8860169273291,49.8836907421725,
50.881364557016,51.5750455984138),.UNSPECIFIED.);
#274=B_SPLINE_CURVE_WITH_KNOTS('',3,(#6794,#6795,#6796,#6797,#6798,#6799,
#6800,#6801,#6802,#6803,#6804,#6805,#6806,#6807,#6808,#6809,#6810,#6811,
#6812,#6813,#6814,#6815),.UNSPECIFIED.,.F.,.F.,(4,3,3,3,3,3,3,4),(-47.8312715558983,
-46.8906692976422,-45.8929954827987,-44.8953216679553,-43.8976478531118,
-42.8999740382684,-41.9023002234249,-41.5480862487187),.UNSPECIFIED.);
#275=B_SPLINE_CURVE_WITH_KNOTS('',3,(#6820,#6821,#6822,#6823,#6824,#6825,
#6826,#6827,#6828,#6829,#6830,#6831,#6832,#6833,#6834,#6835,#6836,#6837,
#6838,#6839,#6840,#6841),.UNSPECIFIED.,.F.,.F.,(4,3,3,3,3,3,3,4),(39.0086749840546,
39.906952593738,40.9046264085815,41.9023002234249,42.8999740382684,43.8976478531118,
44.8953216679553,45.2918602912342),.UNSPECIFIED.);
#276=B_SPLINE_CURVE_WITH_KNOTS('',3,(#6842,#6843,#6844,#6845,#6846,#6847,
#6848,#6849,#6850,#6851,#6852,#6853,#6854,#6855,#6856,#6857,#6858,#6859,
#6860,#6861,#6862,#6863),.UNSPECIFIED.,.F.,.F.,(4,3,3,3,3,3,3,4),(-41.5480862487187,
-40.9046264085815,-39.906952593738,-38.9092787788946,-37.9116049640511,
-36.9139311492077,-35.9162573343642,-35.2649009415391),.UNSPECIFIED.);
#277=B_SPLINE_CURVE_WITH_KNOTS('',3,(#6868,#6869,#6870,#6871,#6872,#6873,
#6874,#6875,#6876,#6877,#6878,#6879,#6880,#6881,#6882,#6883,#6884,#6885,
#6886,#6887,#6888,#6889,#6890,#6891,#6892),.UNSPECIFIED.,.F.,.F.,(4,3,3,
3,3,3,3,3,4),(32.725489676875,32.9232358898339,33.9209097046773,34.9185835195208,
35.9162573343642,36.9139311492077,37.9116049640511,38.9092787788946,39.0086749840546),
 .UNSPECIFIED.);
#278=B_SPLINE_CURVE_WITH_KNOTS('',3,(#6893,#6894,#6895,#6896,#6897,#6898,
#6899,#6900,#6901,#6902,#6903,#6904,#6905,#6906,#6907,#6908,#6909,#6910,
#6911,#6912,#6913,#6914),.UNSPECIFIED.,.F.,.F.,(4,3,3,3,3,3,3,4),(-35.2649009415391,
-34.9185835195208,-33.9209097046773,-32.9232358898339,-31.9255620749904,
-30.927888260147,-29.9302144453035,-28.9817156343595),.UNSPECIFIED.);
#279=B_SPLINE_CURVE_WITH_KNOTS('',3,(#6919,#6920,#6921,#6922,#6923,#6924,
#6925,#6926,#6927,#6928,#6929,#6930,#6931,#6932,#6933,#6934,#6935,#6936,
#6937,#6938,#6939,#6940),.UNSPECIFIED.,.F.,.F.,(4,3,3,3,3,3,3,4),(26.4423043696954,
26.9371930007732,27.9348668156166,28.9325406304601,29.9302144453035,30.927888260147,
31.9255620749904,32.725489676875),.UNSPECIFIED.);
#280=B_SPLINE_CURVE_WITH_KNOTS('',3,(#6941,#6942,#6943,#6944,#6945,#6946,
#6947,#6948,#6949,#6950,#6951,#6952,#6953,#6954,#6955,#6956,#6957,#6958,
#6959,#6960,#6961,#6962,#6963,#6964,#6965),.UNSPECIFIED.,.F.,.F.,(4,3,3,
3,3,3,3,3,4),(-28.9817156343595,-28.9325406304601,-27.9348668156166,-26.9371930007732,
-25.9395191859297,-24.9418453710863,-23.9441715562428,-22.9464977413994,
-22.6985303271799),.UNSPECIFIED.);
#281=B_SPLINE_CURVE_WITH_KNOTS('',3,(#6970,#6971,#6972,#6973,#6974,#6975,
#6976,#6977,#6978,#6979,#6980,#6981,#6982,#6983,#6984,#6985,#6986,#6987,
#6988,#6989,#6990,#6991),.UNSPECIFIED.,.F.,.F.,(4,3,3,3,3,3,3,4),(20.1591190625158,
20.9511501117125,21.9488239265559,22.9464977413994,23.9441715562428,24.9418453710863,
25.9395191859297,26.4423043696954),.UNSPECIFIED.);
#282=B_SPLINE_CURVE_WITH_KNOTS('',3,(#6992,#6993,#6994,#6995,#6996,#6997,
#6998,#6999,#7000,#7001,#7002,#7003,#7004,#7005,#7006,#7007,#7008,#7009,
#7010,#7011,#7012,#7013),.UNSPECIFIED.,.F.,.F.,(4,3,3,3,3,3,3,4),(-22.6985303271799,
-21.9488239265559,-20.9511501117125,-19.953476296869,-18.9558024820256,
-17.9581286671821,-16.9604548523387,-16.4153450200003),.UNSPECIFIED.);
#283=B_SPLINE_CURVE_WITH_KNOTS('',3,(#7018,#7019,#7020,#7021,#7022,#7023,
#7024,#7025,#7026,#7027,#7028,#7029,#7030,#7031,#7032,#7033,#7034,#7035,
#7036,#7037,#7038,#7039,#7040,#7041,#7042),.UNSPECIFIED.,.F.,.F.,(4,3,3,
3,3,3,3,3,4),(13.8759337553362,13.9674334078083,14.9651072226518,15.9627810374952,
16.9604548523387,17.9581286671821,18.9558024820256,19.953476296869,20.1591190625158),
 .UNSPECIFIED.);
#284=B_SPLINE_CURVE_WITH_KNOTS('',3,(#7043,#7044,#7045,#7046,#7047,#7048,
#7049,#7050,#7051,#7052,#7053,#7054,#7055,#7056,#7057,#7058,#7059,#7060,
#7061,#7062,#7063,#7064),.UNSPECIFIED.,.F.,.F.,(4,3,3,3,3,3,3,4),(-16.4153450200003,
-15.9627810374952,-14.9651072226518,-13.9674334078083,-12.9697595929649,
-11.9720857781214,-10.974411963278,-10.1321597128207),.UNSPECIFIED.);
#285=B_SPLINE_CURVE_WITH_KNOTS('',3,(#7070,#7071,#7072,#7073,#7074,#7075,
#7076,#7077,#7078,#7079,#7080,#7081,#7082),.UNSPECIFIED.,.F.,.F.,(4,3,3,
3,4),(-3.84897440564115,-2.99302144453035,-1.9953476296869,-0.997673814843451,
0.),.UNSPECIFIED.);
#286=B_SPLINE_CURVE_WITH_KNOTS('',3,(#7085,#7086,#7087,#7088,#7089,#7090,
#7091,#7092,#7093,#7094,#7095,#7096,#7097,#7098,#7099,#7100,#7101,#7102,
#7103),.UNSPECIFIED.,.F.,.F.,(4,3,3,3,3,3,4),(2.0169448930285,2.99302144453035,
3.99069525937381,4.98836907421726,5.98604288906071,6.98371670390416,7.59274844815666),
 .UNSPECIFIED.);
#287=B_SPLINE_CURVE_WITH_KNOTS('',3,(#7109,#7110,#7111,#7112),
 .UNSPECIFIED.,.F.,.F.,(4,4),(64.141416212773,64.8487979648243),
 .UNSPECIFIED.);
#288=B_SPLINE_CURVE_WITH_KNOTS('',3,(#7115,#7116,#7117,#7118,#7119,#7120,
#7121,#7122,#7123,#7124),.UNSPECIFIED.,.F.,.F.,(4,3,3,4),(-62.8318530717958,
-61.855776520294,-60.8581027054505,-60.3976421702574),.UNSPECIFIED.);
#289=B_SPLINE_CURVE_WITH_KNOTS('',3,(#7129,#7130,#7131,#7132,#7133,#7134,
#7135,#7136,#7137,#7138,#7139,#7140,#7141,#7142,#7143,#7144,#7145,#7146,
#7147,#7148,#7149,#7150,#7151,#7152,#7153),.UNSPECIFIED.,.F.,.F.,(4,3,3,
3,3,3,3,3,4),(57.8582309055934,57.8650812609202,58.8627550757636,59.8604288906071,
60.8581027054505,61.855776520294,62.8534503351374,63.8511241499808,64.141416212773),
 .UNSPECIFIED.);
#290=B_SPLINE_CURVE_WITH_KNOTS('',3,(#7154,#7155,#7156,#7157,#7158,#7159,
#7160,#7161,#7162,#7163,#7164,#7165,#7166,#7167,#7168,#7169,#7170,#7171,
#7172,#7173,#7174,#7175),.UNSPECIFIED.,.F.,.F.,(4,3,3,3,3,3,3,4),(-60.3976421702574,
-59.8604288906071,-58.8627550757636,-57.8650812609202,-56.8674074460767,
-55.8697336312333,-54.8720598163898,-54.1144568630778),.UNSPECIFIED.);
#291=B_SPLINE_CURVE_WITH_KNOTS('',3,(#7180,#7181,#7182,#7183,#7184,#7185,
#7186,#7187,#7188,#7189,#7190,#7191,#7192,#7193,#7194,#7195,#7196,#7197,
#7198,#7199,#7200,#7201),.UNSPECIFIED.,.F.,.F.,(4,3,3,3,3,3,3,4),(51.5750455984138,
51.8790383718595,52.8767121867029,53.8743860015464,54.8720598163898,55.8697336312333,
56.8674074460767,57.8582309055934),.UNSPECIFIED.);
#292=B_SPLINE_CURVE_WITH_KNOTS('',3,(#7202,#7203,#7204,#7205,#7206,#7207,
#7208,#7209,#7210,#7211,#7212,#7213,#7214,#7215,#7216,#7217,#7218,#7219,
#7220,#7221,#7222,#7223,#7224,#7225,#7226),.UNSPECIFIED.,.F.,.F.,(4,3,3,
3,3,3,3,3,4),(-54.1144568630778,-53.8743860015464,-52.8767121867029,-51.8790383718595,
-50.881364557016,-49.8836907421726,-48.8860169273291,-47.8883431124856,
-47.8312715558982),.UNSPECIFIED.);
#293=B_SPLINE_CURVE_WITH_KNOTS('',3,(#7231,#7232,#7233,#7234,#7235,#7236,
#7237,#7238,#7239,#7240,#7241,#7242,#7243,#7244,#7245,#7246,#7247,#7248,
#7249,#7250,#7251,#7252),.UNSPECIFIED.,.F.,.F.,(4,3,3,3,3,3,3,4),(45.2918602912342,
45.8929954827987,46.8906692976422,47.8883431124856,48.8860169273291,49.8836907421725,
50.881364557016,51.5750455984138),.UNSPECIFIED.);
#294=B_SPLINE_CURVE_WITH_KNOTS('',3,(#7253,#7254,#7255,#7256,#7257,#7258,
#7259,#7260,#7261,#7262,#7263,#7264,#7265,#7266,#7267,#7268,#7269,#7270,
#7271,#7272,#7273,#7274),.UNSPECIFIED.,.F.,.F.,(4,3,3,3,3,3,3,4),(-47.8312715558982,
-46.8906692976422,-45.8929954827987,-44.8953216679553,-43.8976478531118,
-42.8999740382684,-41.9023002234249,-41.5480862487187),.UNSPECIFIED.);
#295=B_SPLINE_CURVE_WITH_KNOTS('',3,(#7279,#7280,#7281,#7282,#7283,#7284,
#7285,#7286,#7287,#7288,#7289,#7290,#7291,#7292,#7293,#7294,#7295,#7296,
#7297,#7298,#7299,#7300),.UNSPECIFIED.,.F.,.F.,(4,3,3,3,3,3,3,4),(39.0086749840546,
39.906952593738,40.9046264085815,41.9023002234249,42.8999740382684,43.8976478531118,
44.8953216679553,45.2918602912342),.UNSPECIFIED.);
#296=B_SPLINE_CURVE_WITH_KNOTS('',3,(#7301,#7302,#7303,#7304,#7305,#7306,
#7307,#7308,#7309,#7310,#7311,#7312,#7313,#7314,#7315,#7316,#7317,#7318,
#7319,#7320,#7321,#7322),.UNSPECIFIED.,.F.,.F.,(4,3,3,3,3,3,3,4),(-41.5480862487187,
-40.9046264085815,-39.906952593738,-38.9092787788946,-37.9116049640511,
-36.9139311492077,-35.9162573343642,-35.2649009415391),.UNSPECIFIED.);
#297=B_SPLINE_CURVE_WITH_KNOTS('',3,(#7327,#7328,#7329,#7330,#7331,#7332,
#7333,#7334,#7335,#7336,#7337,#7338,#7339,#7340,#7341,#7342,#7343,#7344,
#7345,#7346,#7347,#7348,#7349,#7350,#7351),.UNSPECIFIED.,.F.,.F.,(4,3,3,
3,3,3,3,3,4),(32.725489676875,32.9232358898339,33.9209097046773,34.9185835195208,
35.9162573343642,36.9139311492077,37.9116049640511,38.9092787788946,39.0086749840546),
 .UNSPECIFIED.);
#298=B_SPLINE_CURVE_WITH_KNOTS('',3,(#7352,#7353,#7354,#7355,#7356,#7357,
#7358,#7359,#7360,#7361,#7362,#7363,#7364,#7365,#7366,#7367,#7368,#7369,
#7370,#7371,#7372,#7373),.UNSPECIFIED.,.F.,.F.,(4,3,3,3,3,3,3,4),(-35.2649009415391,
-34.9185835195208,-33.9209097046773,-32.9232358898339,-31.9255620749904,
-30.927888260147,-29.9302144453035,-28.9817156343595),.UNSPECIFIED.);
#299=B_SPLINE_CURVE_WITH_KNOTS('',3,(#7378,#7379,#7380,#7381,#7382,#7383,
#7384,#7385,#7386,#7387,#7388,#7389,#7390,#7391,#7392,#7393,#7394,#7395,
#7396,#7397,#7398,#7399),.UNSPECIFIED.,.F.,.F.,(4,3,3,3,3,3,3,4),(26.4423043696954,
26.9371930007732,27.9348668156166,28.9325406304601,29.9302144453035,30.927888260147,
31.9255620749904,32.725489676875),.UNSPECIFIED.);
#300=B_SPLINE_CURVE_WITH_KNOTS('',3,(#7400,#7401,#7402,#7403,#7404,#7405,
#7406,#7407,#7408,#7409,#7410,#7411,#7412,#7413,#7414,#7415,#7416,#7417,
#7418,#7419,#7420,#7421,#7422,#7423,#7424),.UNSPECIFIED.,.F.,.F.,(4,3,3,
3,3,3,3,3,4),(-28.9817156343595,-28.9325406304601,-27.9348668156166,-26.9371930007732,
-25.9395191859297,-24.9418453710863,-23.9441715562428,-22.9464977413994,
-22.6985303271799),.UNSPECIFIED.);
#301=B_SPLINE_CURVE_WITH_KNOTS('',3,(#7429,#7430,#7431,#7432,#7433,#7434,
#7435,#7436,#7437,#7438,#7439,#7440,#7441,#7442,#7443,#7444,#7445,#7446,
#7447,#7448,#7449,#7450),.UNSPECIFIED.,.F.,.F.,(4,3,3,3,3,3,3,4),(20.1591190625158,
20.9511501117125,21.9488239265559,22.9464977413994,23.9441715562428,24.9418453710863,
25.9395191859297,26.4423043696954),.UNSPECIFIED.);
#302=B_SPLINE_CURVE_WITH_KNOTS('',3,(#7451,#7452,#7453,#7454,#7455,#7456,
#7457,#7458,#7459,#7460,#7461,#7462,#7463,#7464,#7465,#7466,#7467,#7468,
#7469,#7470,#7471,#7472),.UNSPECIFIED.,.F.,.F.,(4,3,3,3,3,3,3,4),(-22.6985303271799,
-21.9488239265559,-20.9511501117125,-19.953476296869,-18.9558024820256,
-17.9581286671821,-16.9604548523387,-16.4153450200003),.UNSPECIFIED.);
#303=B_SPLINE_CURVE_WITH_KNOTS('',3,(#7477,#7478,#7479,#7480,#7481,#7482,
#7483,#7484,#7485,#7486,#7487,#7488,#7489,#7490,#7491,#7492,#7493,#7494,
#7495,#7496,#7497,#7498,#7499,#7500,#7501),.UNSPECIFIED.,.F.,.F.,(4,3,3,
3,3,3,3,3,4),(13.8759337553362,13.9674334078083,14.9651072226518,15.9627810374952,
16.9604548523387,17.9581286671821,18.9558024820256,19.953476296869,20.1591190625158),
 .UNSPECIFIED.);
#304=B_SPLINE_CURVE_WITH_KNOTS('',3,(#7502,#7503,#7504,#7505,#7506,#7507,
#7508,#7509,#7510,#7511,#7512,#7513,#7514,#7515,#7516,#7517,#7518,#7519,
#7520,#7521,#7522,#7523),.UNSPECIFIED.,.F.,.F.,(4,3,3,3,3,3,3,4),(-16.4153450200003,
-15.9627810374952,-14.9651072226518,-13.9674334078083,-12.9697595929649,
-11.9720857781214,-10.974411963278,-10.1321597128207),.UNSPECIFIED.);
#305=B_SPLINE_CURVE_WITH_KNOTS('',3,(#7529,#7530,#7531,#7532,#7533,#7534,
#7535,#7536,#7537,#7538,#7539,#7540,#7541),.UNSPECIFIED.,.F.,.F.,(4,3,3,
3,4),(-3.84897440564114,-2.99302144453035,-1.9953476296869,-0.997673814843452,
0.),.UNSPECIFIED.);
#306=B_SPLINE_CURVE_WITH_KNOTS('',3,(#7544,#7545,#7546,#7547,#7548,#7549,
#7550,#7551,#7552,#7553,#7554,#7555,#7556,#7557,#7558,#7559,#7560,#7561,
#7562),.UNSPECIFIED.,.F.,.F.,(4,3,3,3,3,3,4),(2.0169448930285,2.99302144453035,
3.9906952593738,4.98836907421725,5.9860428890607,6.98371670390415,7.59274844815666),
 .UNSPECIFIED.);
#307=B_SPLINE_CURVE_WITH_KNOTS('',3,(#7568,#7569,#7570,#7571),
 .UNSPECIFIED.,.F.,.F.,(4,4),(64.141416212773,64.8487979648243),
 .UNSPECIFIED.);
#308=B_SPLINE_CURVE_WITH_KNOTS('',3,(#7574,#7575,#7576,#7577,#7578,#7579,
#7580,#7581,#7582,#7583),.UNSPECIFIED.,.F.,.F.,(4,3,3,4),(-62.8318530717959,
-61.855776520294,-60.8581027054505,-60.3976421702574),.UNSPECIFIED.);
#309=B_SPLINE_CURVE_WITH_KNOTS('',3,(#7588,#7589,#7590,#7591,#7592,#7593,
#7594,#7595,#7596,#7597,#7598,#7599,#7600,#7601,#7602,#7603,#7604,#7605,
#7606,#7607,#7608,#7609,#7610,#7611,#7612),.UNSPECIFIED.,.F.,.F.,(4,3,3,
3,3,3,3,3,4),(57.8582309055934,57.8650812609202,58.8627550757636,59.8604288906071,
60.8581027054505,61.855776520294,62.8534503351374,63.8511241499808,64.141416212773),
 .UNSPECIFIED.);
#310=B_SPLINE_CURVE_WITH_KNOTS('',3,(#7613,#7614,#7615,#7616,#7617,#7618,
#7619,#7620,#7621,#7622,#7623,#7624,#7625,#7626,#7627,#7628,#7629,#7630,
#7631,#7632,#7633,#7634),.UNSPECIFIED.,.F.,.F.,(4,3,3,3,3,3,3,4),(-60.3976421702574,
-59.8604288906071,-58.8627550757636,-57.8650812609202,-56.8674074460767,
-55.8697336312333,-54.8720598163898,-54.1144568630778),.UNSPECIFIED.);
#311=B_SPLINE_CURVE_WITH_KNOTS('',3,(#7639,#7640,#7641,#7642,#7643,#7644,
#7645,#7646,#7647,#7648,#7649,#7650,#7651,#7652,#7653,#7654,#7655,#7656,
#7657,#7658,#7659,#7660),.UNSPECIFIED.,.F.,.F.,(4,3,3,3,3,3,3,4),(51.5750455984138,
51.8790383718595,52.8767121867029,53.8743860015464,54.8720598163898,55.8697336312333,
56.8674074460767,57.8582309055934),.UNSPECIFIED.);
#312=B_SPLINE_CURVE_WITH_KNOTS('',3,(#7661,#7662,#7663,#7664,#7665,#7666,
#7667,#7668,#7669,#7670,#7671,#7672,#7673,#7674,#7675,#7676,#7677,#7678,
#7679,#7680,#7681,#7682,#7683,#7684,#7685),.UNSPECIFIED.,.F.,.F.,(4,3,3,
3,3,3,3,3,4),(-54.1144568630778,-53.8743860015464,-52.8767121867029,-51.8790383718595,
-50.881364557016,-49.8836907421725,-48.8860169273291,-47.8883431124856,
-47.8312715558982),.UNSPECIFIED.);
#313=B_SPLINE_CURVE_WITH_KNOTS('',3,(#7690,#7691,#7692,#7693,#7694,#7695,
#7696,#7697,#7698,#7699,#7700,#7701,#7702,#7703,#7704,#7705,#7706,#7707,
#7708,#7709,#7710,#7711),.UNSPECIFIED.,.F.,.F.,(4,3,3,3,3,3,3,4),(45.2918602912342,
45.8929954827987,46.8906692976422,47.8883431124857,48.8860169273291,49.8836907421726,
50.881364557016,51.5750455984138),.UNSPECIFIED.);
#314=B_SPLINE_CURVE_WITH_KNOTS('',3,(#7712,#7713,#7714,#7715,#7716,#7717,
#7718,#7719,#7720,#7721,#7722,#7723,#7724,#7725,#7726,#7727,#7728,#7729,
#7730,#7731,#7732,#7733),.UNSPECIFIED.,.F.,.F.,(4,3,3,3,3,3,3,4),(-47.8312715558982,
-46.8906692976422,-45.8929954827987,-44.8953216679553,-43.8976478531118,
-42.8999740382684,-41.9023002234249,-41.5480862487187),.UNSPECIFIED.);
#315=B_SPLINE_CURVE_WITH_KNOTS('',3,(#7738,#7739,#7740,#7741,#7742,#7743,
#7744,#7745,#7746,#7747,#7748,#7749,#7750,#7751,#7752,#7753,#7754,#7755,
#7756,#7757,#7758,#7759),.UNSPECIFIED.,.F.,.F.,(4,3,3,3,3,3,3,4),(39.0086749840546,
39.906952593738,40.9046264085815,41.9023002234249,42.8999740382684,43.8976478531118,
44.8953216679553,45.2918602912342),.UNSPECIFIED.);
#316=B_SPLINE_CURVE_WITH_KNOTS('',3,(#7760,#7761,#7762,#7763,#7764,#7765,
#7766,#7767,#7768,#7769,#7770,#7771,#7772,#7773,#7774,#7775,#7776,#7777,
#7778,#7779,#7780,#7781),.UNSPECIFIED.,.F.,.F.,(4,3,3,3,3,3,3,4),(-41.5480862487187,
-40.9046264085815,-39.906952593738,-38.9092787788946,-37.9116049640511,
-36.9139311492077,-35.9162573343642,-35.2649009415391),.UNSPECIFIED.);
#317=B_SPLINE_CURVE_WITH_KNOTS('',3,(#7786,#7787,#7788,#7789,#7790,#7791,
#7792,#7793,#7794,#7795,#7796,#7797,#7798,#7799,#7800,#7801,#7802,#7803,
#7804,#7805,#7806,#7807,#7808,#7809,#7810),.UNSPECIFIED.,.F.,.F.,(4,3,3,
3,3,3,3,3,4),(32.725489676875,32.9232358898339,33.9209097046773,34.9185835195208,
35.9162573343642,36.9139311492077,37.9116049640511,38.9092787788946,39.0086749840546),
 .UNSPECIFIED.);
#318=B_SPLINE_CURVE_WITH_KNOTS('',3,(#7811,#7812,#7813,#7814,#7815,#7816,
#7817,#7818,#7819,#7820,#7821,#7822,#7823,#7824,#7825,#7826,#7827,#7828,
#7829,#7830,#7831,#7832),.UNSPECIFIED.,.F.,.F.,(4,3,3,3,3,3,3,4),(-35.2649009415391,
-34.9185835195208,-33.9209097046773,-32.9232358898339,-31.9255620749904,
-30.927888260147,-29.9302144453035,-28.9817156343595),.UNSPECIFIED.);
#319=B_SPLINE_CURVE_WITH_KNOTS('',3,(#7837,#7838,#7839,#7840,#7841,#7842,
#7843,#7844,#7845,#7846,#7847,#7848,#7849,#7850,#7851,#7852,#7853,#7854,
#7855,#7856,#7857,#7858),.UNSPECIFIED.,.F.,.F.,(4,3,3,3,3,3,3,4),(26.4423043696954,
26.9371930007732,27.9348668156166,28.9325406304601,29.9302144453035,30.927888260147,
31.9255620749904,32.725489676875),.UNSPECIFIED.);
#320=B_SPLINE_CURVE_WITH_KNOTS('',3,(#7859,#7860,#7861,#7862,#7863,#7864,
#7865,#7866,#7867,#7868,#7869,#7870,#7871,#7872,#7873,#7874,#7875,#7876,
#7877,#7878,#7879,#7880,#7881,#7882,#7883),.UNSPECIFIED.,.F.,.F.,(4,3,3,
3,3,3,3,3,4),(-28.9817156343595,-28.9325406304601,-27.9348668156166,-26.9371930007732,
-25.9395191859297,-24.9418453710863,-23.9441715562428,-22.9464977413994,
-22.6985303271799),.UNSPECIFIED.);
#321=B_SPLINE_CURVE_WITH_KNOTS('',3,(#7888,#7889,#7890,#7891,#7892,#7893,
#7894,#7895,#7896,#7897,#7898,#7899,#7900,#7901,#7902,#7903,#7904,#7905,
#7906,#7907,#7908,#7909),.UNSPECIFIED.,.F.,.F.,(4,3,3,3,3,3,3,4),(20.1591190625158,
20.9511501117125,21.9488239265559,22.9464977413994,23.9441715562428,24.9418453710863,
25.9395191859297,26.4423043696954),.UNSPECIFIED.);
#322=B_SPLINE_CURVE_WITH_KNOTS('',3,(#7910,#7911,#7912,#7913,#7914,#7915,
#7916,#7917,#7918,#7919,#7920,#7921,#7922,#7923,#7924,#7925,#7926,#7927,
#7928,#7929,#7930,#7931),.UNSPECIFIED.,.F.,.F.,(4,3,3,3,3,3,3,4),(-22.6985303271799,
-21.9488239265559,-20.9511501117125,-19.953476296869,-18.9558024820256,
-17.9581286671821,-16.9604548523387,-16.4153450200003),.UNSPECIFIED.);
#323=B_SPLINE_CURVE_WITH_KNOTS('',3,(#7936,#7937,#7938,#7939,#7940,#7941,
#7942,#7943,#7944,#7945,#7946,#7947,#7948,#7949,#7950,#7951,#7952,#7953,
#7954,#7955,#7956,#7957,#7958,#7959,#7960),.UNSPECIFIED.,.F.,.F.,(4,3,3,
3,3,3,3,3,4),(13.8759337553362,13.9674334078083,14.9651072226518,15.9627810374952,
16.9604548523387,17.9581286671821,18.9558024820256,19.953476296869,20.1591190625158),
 .UNSPECIFIED.);
#324=B_SPLINE_CURVE_WITH_KNOTS('',3,(#7961,#7962,#7963,#7964,#7965,#7966,
#7967,#7968,#7969,#7970,#7971,#7972,#7973,#7974,#7975,#7976,#7977,#7978,
#7979,#7980,#7981,#7982),.UNSPECIFIED.,.F.,.F.,(4,3,3,3,3,3,3,4),(-16.4153450200003,
-15.9627810374952,-14.9651072226518,-13.9674334078083,-12.9697595929649,
-11.9720857781214,-10.974411963278,-10.1321597128207),.UNSPECIFIED.);
#325=B_SPLINE_CURVE_WITH_KNOTS('',3,(#7988,#7989,#7990,#7991,#7992,#7993,
#7994,#7995,#7996,#7997,#7998,#7999,#8000),.UNSPECIFIED.,.F.,.F.,(4,3,3,
3,4),(-3.84897440564114,-2.99302144453035,-1.9953476296869,-0.997673814843451,
0.),.UNSPECIFIED.);
#326=B_SPLINE_CURVE_WITH_KNOTS('',3,(#8003,#8004,#8005,#8006,#8007,#8008,
#8009,#8010,#8011,#8012,#8013,#8014,#8015,#8016,#8017,#8018,#8019,#8020,
#8021),.UNSPECIFIED.,.F.,.F.,(4,3,3,3,3,3,4),(2.01694489302845,2.99302144453035,
3.9906952593738,4.98836907421725,5.98604288906071,6.98371670390416,7.59274844815666),
 .UNSPECIFIED.);
#327=B_SPLINE_CURVE_WITH_KNOTS('',3,(#8027,#8028,#8029,#8030,#8031,#8032,
#8033,#8034),.UNSPECIFIED.,.F.,.F.,(4,1,1,1,1,4),(72.2566310325652,72.7170915677583,
73.7147653826018,74.7124391974452,75.7101130122887,76.7077868271321),
 .UNSPECIFIED.);
#328=B_SPLINE_CURVE_WITH_KNOTS('',3,(#8037,#8038,#8039,#8040,#8041,#8042,
#8043,#8044,#8045),.UNSPECIFIED.,.F.,.F.,(4,1,1,1,1,1,4),(72.2566310325652,
72.263481387892,73.2611552027354,74.2588290175789,75.2565028324223,76.2541766472658,
77.2302531987677),.UNSPECIFIED.);
#329=B_SPLINE_CURVE_WITH_KNOTS('',3,(#8050,#8051,#8052,#8053,#8054,#8055,
#8056,#8057,#8058,#8059),.UNSPECIFIED.,.F.,.F.,(4,1,1,1,1,1,1,4),(65.9734457253856,
66.7310486786976,67.728722493541,68.7263963083845,69.7240701232279,70.7217439380714,
71.7194177529149,72.2566310325652),.UNSPECIFIED.);
#330=B_SPLINE_CURVE_WITH_KNOTS('',3,(#8060,#8061,#8062,#8063,#8064,#8065,
#8066,#8067,#8068,#8069),.UNSPECIFIED.,.F.,.F.,(4,1,1,1,1,1,1,4),(65.9734457253856,
66.2774384988313,67.2751123136747,68.2727861285182,69.2704599433616,70.2681337582051,
71.2658075730485,72.2566310325652),.UNSPECIFIED.);
#331=B_SPLINE_CURVE_WITH_KNOTS('',3,(#8074,#8075,#8076,#8077,#8078,#8079,
#8080,#8081,#8082,#8083,#8084),.UNSPECIFIED.,.F.,.F.,(4,1,1,1,1,1,1,1,4),
(59.6902604182061,59.7473319747934,60.7450057896369,61.7426796044803,62.7403534193238,
63.7380272341672,64.7357010490107,65.7333748638542,65.9734457253856),
 .UNSPECIFIED.);
#332=B_SPLINE_CURVE_WITH_KNOTS('',3,(#8085,#8086,#8087,#8088,#8089,#8090,
#8091,#8092,#8093,#8094),.UNSPECIFIED.,.F.,.F.,(4,1,1,1,1,1,1,4),(59.6902604182061,
60.2913956097706,61.289069424614,62.2867432394575,63.2844170543009,64.2820908691444,
65.2797646839878,65.9734457253856),.UNSPECIFIED.);
#333=B_SPLINE_CURVE_WITH_KNOTS('',3,(#8099,#8100,#8101,#8102,#8103,#8104,
#8105,#8106,#8107,#8108),.UNSPECIFIED.,.F.,.F.,(4,1,1,1,1,1,1,4),(53.4070751110265,
53.7612890857327,54.7589629005762,55.7566367154196,56.7543105302631,57.7519843451065,
58.74965815995,59.6902604182061),.UNSPECIFIED.);
#334=B_SPLINE_CURVE_WITH_KNOTS('',3,(#8109,#8110,#8111,#8112,#8113,#8114,
#8115,#8116,#8117,#8118),.UNSPECIFIED.,.F.,.F.,(4,1,1,1,1,1,1,4),(53.4070751110265,
54.3053527207099,55.3030265355533,56.3007003503968,57.2983741652402,58.2960479800837,
59.2937217949271,59.6902604182061),.UNSPECIFIED.);
#335=B_SPLINE_CURVE_WITH_KNOTS('',3,(#8123,#8124,#8125,#8126,#8127,#8128,
#8129,#8130,#8131,#8132),.UNSPECIFIED.,.F.,.F.,(4,1,1,1,1,1,1,4),(47.1238898038469,
47.775246196672,48.7729200115155,49.7705938263589,50.7682676412024,51.7659414560458,
52.7636152708893,53.4070751110265),.UNSPECIFIED.);
#336=B_SPLINE_CURVE_WITH_KNOTS('',3,(#8133,#8134,#8135,#8136,#8137,#8138,
#8139,#8140,#8141,#8142,#8143),.UNSPECIFIED.,.F.,.F.,(4,1,1,1,1,1,1,1,4),
(47.1238898038469,47.3216360168057,48.3193098316492,49.3169836464926,50.3146574613361,
51.3123312761795,52.310005091023,53.3076789058664,53.4070751110265),
 .UNSPECIFIED.);
#337=B_SPLINE_CURVE_WITH_KNOTS('',3,(#8148,#8149,#8150,#8151,#8152,#8153,
#8154,#8155,#8156,#8157),.UNSPECIFIED.,.F.,.F.,(4,1,1,1,1,1,1,4),(40.8407044966673,
41.7892033076113,42.7868771224548,43.7845509372982,44.7822247521417,45.7798985669851,
46.7775723818286,47.1238898038469),.UNSPECIFIED.);
#338=B_SPLINE_CURVE_WITH_KNOTS('',3,(#8158,#8159,#8160,#8161,#8162,#8163,
#8164,#8165,#8166,#8167),.UNSPECIFIED.,.F.,.F.,(4,1,1,1,1,1,1,4),(40.8407044966673,
41.335593127745,42.3332669425885,43.3309407574319,44.3286145722754,45.3262883871188,
46.3239622019623,47.1238898038469),.UNSPECIFIED.);
#339=B_SPLINE_CURVE_WITH_KNOTS('',3,(#8172,#8173,#8174,#8175,#8176,#8177,
#8178,#8179,#8180,#8181,#8182),.UNSPECIFIED.,.F.,.F.,(4,1,1,1,1,1,1,1,4),
(34.5575191894877,34.8054866037072,35.8031604185506,36.8008342333941,37.7985080482375,
38.796181863081,39.7938556779244,40.7915294927679,40.8407044966673),
 .UNSPECIFIED.);
#340=B_SPLINE_CURVE_WITH_KNOTS('',3,(#8183,#8184,#8185,#8186,#8187,#8188,
#8189,#8190,#8191,#8192),.UNSPECIFIED.,.F.,.F.,(4,1,1,1,1,1,1,4),(34.5575191894877,
35.3495502386843,36.3472240535278,37.3448978683712,38.3425716832147,39.3402454980581,
40.3379193129016,40.8407044966673),.UNSPECIFIED.);
#341=B_SPLINE_CURVE_WITH_KNOTS('',3,(#8197,#8198,#8199,#8200,#8201,#8202,
#8203,#8204,#8205,#8206),.UNSPECIFIED.,.F.,.F.,(4,1,1,1,1,1,1,4),(28.2743338823081,
28.8194437146465,29.8171175294899,30.8147913443334,31.8124651591768,32.8101389740203,
33.8078127888637,34.5575191894877),.UNSPECIFIED.);
#342=B_SPLINE_CURVE_WITH_KNOTS('',3,(#8207,#8208,#8209,#8210,#8211,#8212,
#8213,#8214,#8215,#8216,#8217),.UNSPECIFIED.,.F.,.F.,(4,1,1,1,1,1,1,1,4),
(28.2743338823081,28.3658335347801,29.3635073496236,30.361181164467,31.3588549793105,
32.3565287941539,33.3542026089974,34.3518764238408,34.5575191894877),
 .UNSPECIFIED.);
#343=B_SPLINE_CURVE_WITH_KNOTS('',3,(#8222,#8223,#8224,#8225,#8226,#8227,
#8228,#8229,#8230,#8231),.UNSPECIFIED.,.F.,.F.,(4,1,1,1,1,1,1,4),(21.9911485751285,
22.8334008255858,23.8310746404292,24.8287484552727,25.8264222701161,26.8240960849596,
27.821769899803,28.2743338823081),.UNSPECIFIED.);
#344=B_SPLINE_CURVE_WITH_KNOTS('',3,(#8232,#8233,#8234,#8235,#8236,#8237,
#8238,#8239,#8240,#8241),.UNSPECIFIED.,.F.,.F.,(4,1,1,1,1,1,1,4),(21.9911485751285,
22.3797906457194,23.3774644605629,24.3751382754063,25.3728120902498,26.3704859050932,
27.3681597199367,28.2743338823081),.UNSPECIFIED.);
#345=B_SPLINE_CURVE_WITH_KNOTS('',3,(#8247,#8248,#8249,#8250,#8251),
 .UNSPECIFIED.,.F.,.F.,(4,1,4),(14.3984001269718,15.3960739418153,15.7079632679489),
 .UNSPECIFIED.);
#346=B_SPLINE_CURVE_WITH_KNOTS('',3,(#8254,#8255,#8256,#8257,#8258),
 .UNSPECIFIED.,.F.,.F.,(4,1,4),(13.8759337553362,14.8520103068381,15.7079632679489),
 .UNSPECIFIED.);
#347=B_SPLINE_CURVE_WITH_KNOTS('',3,(#8264,#8265,#8266,#8267,#8268,#8269,
#8270,#8271),.UNSPECIFIED.,.F.,.F.,(4,1,1,1,1,4),(72.2566310325652,72.7170915677583,
73.7147653826017,74.7124391974452,75.7101130122886,76.7077868271321),
 .UNSPECIFIED.);
#348=B_SPLINE_CURVE_WITH_KNOTS('',3,(#8274,#8275,#8276,#8277,#8278,#8279,
#8280,#8281,#8282),.UNSPECIFIED.,.F.,.F.,(4,1,1,1,1,1,4),(72.2566310325652,
72.263481387892,73.2611552027354,74.2588290175789,75.2565028324223,76.2541766472658,
77.2302531987677),.UNSPECIFIED.);
#349=B_SPLINE_CURVE_WITH_KNOTS('',3,(#8287,#8288,#8289,#8290,#8291,#8292,
#8293,#8294,#8295,#8296),.UNSPECIFIED.,.F.,.F.,(4,1,1,1,1,1,1,4),(65.9734457253856,
66.7310486786976,67.728722493541,68.7263963083845,69.7240701232279,70.7217439380714,
71.7194177529148,72.2566310325652),.UNSPECIFIED.);
#350=B_SPLINE_CURVE_WITH_KNOTS('',3,(#8297,#8298,#8299,#8300,#8301,#8302,
#8303,#8304,#8305,#8306),.UNSPECIFIED.,.F.,.F.,(4,1,1,1,1,1,1,4),(65.9734457253856,
66.2774384988313,67.2751123136747,68.2727861285182,69.2704599433616,70.2681337582051,
71.2658075730485,72.2566310325652),.UNSPECIFIED.);
#351=B_SPLINE_CURVE_WITH_KNOTS('',3,(#8311,#8312,#8313,#8314,#8315,#8316,
#8317,#8318,#8319,#8320,#8321),.UNSPECIFIED.,.F.,.F.,(4,1,1,1,1,1,1,1,4),
(59.6902604182061,59.7473319747934,60.7450057896369,61.7426796044803,62.7403534193238,
63.7380272341672,64.7357010490107,65.7333748638541,65.9734457253856),
 .UNSPECIFIED.);
#352=B_SPLINE_CURVE_WITH_KNOTS('',3,(#8322,#8323,#8324,#8325,#8326,#8327,
#8328,#8329,#8330,#8331),.UNSPECIFIED.,.F.,.F.,(4,1,1,1,1,1,1,4),(59.6902604182061,
60.2913956097706,61.289069424614,62.2867432394575,63.2844170543009,64.2820908691444,
65.2797646839878,65.9734457253856),.UNSPECIFIED.);
#353=B_SPLINE_CURVE_WITH_KNOTS('',3,(#8336,#8337,#8338,#8339,#8340,#8341,
#8342,#8343,#8344,#8345),.UNSPECIFIED.,.F.,.F.,(4,1,1,1,1,1,1,4),(53.4070751110265,
53.7612890857327,54.7589629005762,55.7566367154196,56.7543105302631,57.7519843451065,
58.74965815995,59.6902604182061),.UNSPECIFIED.);
#354=B_SPLINE_CURVE_WITH_KNOTS('',3,(#8346,#8347,#8348,#8349,#8350,#8351,
#8352,#8353,#8354,#8355),.UNSPECIFIED.,.F.,.F.,(4,1,1,1,1,1,1,4),(53.4070751110265,
54.3053527207099,55.3030265355533,56.3007003503968,57.2983741652402,58.2960479800837,
59.2937217949271,59.6902604182061),.UNSPECIFIED.);
#355=B_SPLINE_CURVE_WITH_KNOTS('',3,(#8360,#8361,#8362,#8363,#8364,#8365,
#8366,#8367,#8368,#8369),.UNSPECIFIED.,.F.,.F.,(4,1,1,1,1,1,1,4),(47.1238898038469,
47.775246196672,48.7729200115155,49.7705938263589,50.7682676412024,51.7659414560458,
52.7636152708893,53.4070751110265),.UNSPECIFIED.);
#356=B_SPLINE_CURVE_WITH_KNOTS('',3,(#8370,#8371,#8372,#8373,#8374,#8375,
#8376,#8377,#8378,#8379,#8380),.UNSPECIFIED.,.F.,.F.,(4,1,1,1,1,1,1,1,4),
(47.1238898038469,47.3216360168057,48.3193098316492,49.3169836464926,50.3146574613361,
51.3123312761795,52.310005091023,53.3076789058664,53.4070751110265),
 .UNSPECIFIED.);
#357=B_SPLINE_CURVE_WITH_KNOTS('',3,(#8385,#8386,#8387,#8388,#8389,#8390,
#8391,#8392,#8393,#8394),.UNSPECIFIED.,.F.,.F.,(4,1,1,1,1,1,1,4),(40.8407044966673,
41.7892033076113,42.7868771224548,43.7845509372982,44.7822247521417,45.7798985669851,
46.7775723818286,47.1238898038469),.UNSPECIFIED.);
#358=B_SPLINE_CURVE_WITH_KNOTS('',3,(#8395,#8396,#8397,#8398,#8399,#8400,
#8401,#8402,#8403,#8404),.UNSPECIFIED.,.F.,.F.,(4,1,1,1,1,1,1,4),(40.8407044966673,
41.335593127745,42.3332669425884,43.3309407574319,44.3286145722753,45.3262883871188,
46.3239622019622,47.1238898038469),.UNSPECIFIED.);
#359=B_SPLINE_CURVE_WITH_KNOTS('',3,(#8409,#8410,#8411,#8412,#8413,#8414,
#8415,#8416,#8417,#8418,#8419),.UNSPECIFIED.,.F.,.F.,(4,1,1,1,1,1,1,1,4),
(34.5575191894877,34.8054866037072,35.8031604185506,36.8008342333941,37.7985080482375,
38.796181863081,39.7938556779244,40.7915294927679,40.8407044966673),
 .UNSPECIFIED.);
#360=B_SPLINE_CURVE_WITH_KNOTS('',3,(#8420,#8421,#8422,#8423,#8424,#8425,
#8426,#8427,#8428,#8429),.UNSPECIFIED.,.F.,.F.,(4,1,1,1,1,1,1,4),(34.5575191894877,
35.3495502386843,36.3472240535277,37.3448978683712,38.3425716832146,39.3402454980581,
40.3379193129015,40.8407044966673),.UNSPECIFIED.);
#361=B_SPLINE_CURVE_WITH_KNOTS('',3,(#8434,#8435,#8436,#8437,#8438,#8439,
#8440,#8441,#8442,#8443),.UNSPECIFIED.,.F.,.F.,(4,1,1,1,1,1,1,4),(28.2743338823081,
28.8194437146464,29.8171175294899,30.8147913443333,31.8124651591768,32.8101389740202,
33.8078127888637,34.5575191894877),.UNSPECIFIED.);
#362=B_SPLINE_CURVE_WITH_KNOTS('',3,(#8444,#8445,#8446,#8447,#8448,#8449,
#8450,#8451,#8452,#8453,#8454),.UNSPECIFIED.,.F.,.F.,(4,1,1,1,1,1,1,1,4),
(28.2743338823081,28.3658335347801,29.3635073496236,30.361181164467,31.3588549793105,
32.3565287941539,33.3542026089974,34.3518764238408,34.5575191894877),
 .UNSPECIFIED.);
#363=B_SPLINE_CURVE_WITH_KNOTS('',3,(#8459,#8460,#8461,#8462,#8463,#8464,
#8465,#8466,#8467,#8468),.UNSPECIFIED.,.F.,.F.,(4,1,1,1,1,1,1,4),(21.9911485751285,
22.8334008255857,23.8310746404292,24.8287484552726,25.8264222701161,26.8240960849595,
27.821769899803,28.2743338823081),.UNSPECIFIED.);
#364=B_SPLINE_CURVE_WITH_KNOTS('',3,(#8469,#8470,#8471,#8472,#8473,#8474,
#8475,#8476,#8477,#8478),.UNSPECIFIED.,.F.,.F.,(4,1,1,1,1,1,1,4),(21.9911485751285,
22.3797906457194,23.3774644605629,24.3751382754063,25.3728120902498,26.3704859050932,
27.3681597199367,28.2743338823081),.UNSPECIFIED.);
#365=B_SPLINE_CURVE_WITH_KNOTS('',3,(#8484,#8485,#8486,#8487,#8488),
 .UNSPECIFIED.,.F.,.F.,(4,1,4),(14.3984001269718,15.3960739418153,15.7079632679489),
 .UNSPECIFIED.);
#366=B_SPLINE_CURVE_WITH_KNOTS('',3,(#8491,#8492,#8493,#8494,#8495),
 .UNSPECIFIED.,.F.,.F.,(4,1,4),(13.8759337553362,14.8520103068381,15.7079632679489),
 .UNSPECIFIED.);
#367=B_SPLINE_CURVE_WITH_KNOTS('',3,(#8501,#8502,#8503,#8504,#8505,#8506,
#8507,#8508),.UNSPECIFIED.,.F.,.F.,(4,1,1,1,1,4),(72.2566310325652,72.7170915677583,
73.7147653826018,74.7124391974452,75.7101130122887,76.7077868271321),
 .UNSPECIFIED.);
#368=B_SPLINE_CURVE_WITH_KNOTS('',3,(#8511,#8512,#8513,#8514,#8515,#8516,
#8517,#8518,#8519),.UNSPECIFIED.,.F.,.F.,(4,1,1,1,1,1,4),(72.2566310325652,
72.263481387892,73.2611552027354,74.2588290175789,75.2565028324223,76.2541766472658,
77.2302531987677),.UNSPECIFIED.);
#369=B_SPLINE_CURVE_WITH_KNOTS('',3,(#8524,#8525,#8526,#8527,#8528,#8529,
#8530,#8531,#8532,#8533),.UNSPECIFIED.,.F.,.F.,(4,1,1,1,1,1,1,4),(65.9734457253856,
66.7310486786976,67.728722493541,68.7263963083845,69.7240701232279,70.7217439380714,
71.7194177529149,72.2566310325652),.UNSPECIFIED.);
#370=B_SPLINE_CURVE_WITH_KNOTS('',3,(#8534,#8535,#8536,#8537,#8538,#8539,
#8540,#8541,#8542,#8543),.UNSPECIFIED.,.F.,.F.,(4,1,1,1,1,1,1,4),(65.9734457253856,
66.2774384988313,67.2751123136747,68.2727861285182,69.2704599433616,70.2681337582051,
71.2658075730485,72.2566310325652),.UNSPECIFIED.);
#371=B_SPLINE_CURVE_WITH_KNOTS('',3,(#8548,#8549,#8550,#8551,#8552,#8553,
#8554,#8555,#8556,#8557,#8558),.UNSPECIFIED.,.F.,.F.,(4,1,1,1,1,1,1,1,4),
(59.6902604182061,59.7473319747934,60.7450057896369,61.7426796044803,62.7403534193238,
63.7380272341672,64.7357010490107,65.7333748638542,65.9734457253856),
 .UNSPECIFIED.);
#372=B_SPLINE_CURVE_WITH_KNOTS('',3,(#8559,#8560,#8561,#8562,#8563,#8564,
#8565,#8566,#8567,#8568),.UNSPECIFIED.,.F.,.F.,(4,1,1,1,1,1,1,4),(59.6902604182061,
60.2913956097706,61.289069424614,62.2867432394575,63.2844170543009,64.2820908691444,
65.2797646839878,65.9734457253856),.UNSPECIFIED.);
#373=B_SPLINE_CURVE_WITH_KNOTS('',3,(#8573,#8574,#8575,#8576,#8577,#8578,
#8579,#8580,#8581,#8582),.UNSPECIFIED.,.F.,.F.,(4,1,1,1,1,1,1,4),(53.4070751110265,
53.7612890857327,54.7589629005762,55.7566367154196,56.7543105302631,57.7519843451065,
58.74965815995,59.6902604182061),.UNSPECIFIED.);
#374=B_SPLINE_CURVE_WITH_KNOTS('',3,(#8583,#8584,#8585,#8586,#8587,#8588,
#8589,#8590,#8591,#8592),.UNSPECIFIED.,.F.,.F.,(4,1,1,1,1,1,1,4),(53.4070751110265,
54.3053527207099,55.3030265355533,56.3007003503968,57.2983741652402,58.2960479800837,
59.2937217949271,59.6902604182061),.UNSPECIFIED.);
#375=B_SPLINE_CURVE_WITH_KNOTS('',3,(#8597,#8598,#8599,#8600,#8601,#8602,
#8603,#8604,#8605,#8606),.UNSPECIFIED.,.F.,.F.,(4,1,1,1,1,1,1,4),(47.1238898038469,
47.775246196672,48.7729200115155,49.7705938263589,50.7682676412024,51.7659414560458,
52.7636152708893,53.4070751110265),.UNSPECIFIED.);
#376=B_SPLINE_CURVE_WITH_KNOTS('',3,(#8607,#8608,#8609,#8610,#8611,#8612,
#8613,#8614,#8615,#8616,#8617),.UNSPECIFIED.,.F.,.F.,(4,1,1,1,1,1,1,1,4),
(47.1238898038469,47.3216360168057,48.3193098316492,49.3169836464926,50.3146574613361,
51.3123312761795,52.310005091023,53.3076789058664,53.4070751110265),
 .UNSPECIFIED.);
#377=B_SPLINE_CURVE_WITH_KNOTS('',3,(#8622,#8623,#8624,#8625,#8626,#8627,
#8628,#8629,#8630,#8631),.UNSPECIFIED.,.F.,.F.,(4,1,1,1,1,1,1,4),(40.8407044966673,
41.7892033076113,42.7868771224548,43.7845509372982,44.7822247521417,45.7798985669851,
46.7775723818286,47.1238898038469),.UNSPECIFIED.);
#378=B_SPLINE_CURVE_WITH_KNOTS('',3,(#8632,#8633,#8634,#8635,#8636,#8637,
#8638,#8639,#8640,#8641),.UNSPECIFIED.,.F.,.F.,(4,1,1,1,1,1,1,4),(40.8407044966673,
41.335593127745,42.3332669425885,43.3309407574319,44.3286145722754,45.3262883871188,
46.3239622019623,47.1238898038469),.UNSPECIFIED.);
#379=B_SPLINE_CURVE_WITH_KNOTS('',3,(#8646,#8647,#8648,#8649,#8650,#8651,
#8652,#8653,#8654,#8655,#8656),.UNSPECIFIED.,.F.,.F.,(4,1,1,1,1,1,1,1,4),
(34.5575191894877,34.8054866037072,35.8031604185506,36.8008342333941,37.7985080482375,
38.796181863081,39.7938556779244,40.7915294927679,40.8407044966673),
 .UNSPECIFIED.);
#380=B_SPLINE_CURVE_WITH_KNOTS('',3,(#8657,#8658,#8659,#8660,#8661,#8662,
#8663,#8664,#8665,#8666),.UNSPECIFIED.,.F.,.F.,(4,1,1,1,1,1,1,4),(34.5575191894877,
35.3495502386843,36.3472240535278,37.3448978683712,38.3425716832147,39.3402454980581,
40.3379193129016,40.8407044966673),.UNSPECIFIED.);
#381=B_SPLINE_CURVE_WITH_KNOTS('',3,(#8671,#8672,#8673,#8674,#8675,#8676,
#8677,#8678,#8679,#8680),.UNSPECIFIED.,.F.,.F.,(4,1,1,1,1,1,1,4),(28.2743338823081,
28.8194437146465,29.8171175294899,30.8147913443334,31.8124651591768,32.8101389740203,
33.8078127888637,34.5575191894877),.UNSPECIFIED.);
#382=B_SPLINE_CURVE_WITH_KNOTS('',3,(#8681,#8682,#8683,#8684,#8685,#8686,
#8687,#8688,#8689,#8690,#8691),.UNSPECIFIED.,.F.,.F.,(4,1,1,1,1,1,1,1,4),
(28.2743338823081,28.3658335347801,29.3635073496236,30.361181164467,31.3588549793105,
32.3565287941539,33.3542026089974,34.3518764238408,34.5575191894877),
 .UNSPECIFIED.);
#383=B_SPLINE_CURVE_WITH_KNOTS('',3,(#8696,#8697,#8698,#8699,#8700,#8701,
#8702,#8703,#8704,#8705),.UNSPECIFIED.,.F.,.F.,(4,1,1,1,1,1,1,4),(21.9911485751285,
22.8334008255858,23.8310746404292,24.8287484552727,25.8264222701161,26.8240960849596,
27.821769899803,28.2743338823081),.UNSPECIFIED.);
#384=B_SPLINE_CURVE_WITH_KNOTS('',3,(#8706,#8707,#8708,#8709,#8710,#8711,
#8712,#8713,#8714,#8715),.UNSPECIFIED.,.F.,.F.,(4,1,1,1,1,1,1,4),(21.9911485751285,
22.3797906457194,23.3774644605629,24.3751382754063,25.3728120902498,26.3704859050932,
27.3681597199367,28.2743338823081),.UNSPECIFIED.);
#385=B_SPLINE_CURVE_WITH_KNOTS('',3,(#8721,#8722,#8723,#8724,#8725),
 .UNSPECIFIED.,.F.,.F.,(4,1,4),(14.3984001269718,15.3960739418153,15.7079632679489),
 .UNSPECIFIED.);
#386=B_SPLINE_CURVE_WITH_KNOTS('',3,(#8728,#8729,#8730,#8731,#8732),
 .UNSPECIFIED.,.F.,.F.,(4,1,4),(13.8759337553362,14.8520103068381,15.7079632679489),
 .UNSPECIFIED.);
#387=B_SPLINE_CURVE_WITH_KNOTS('',3,(#8738,#8739,#8740,#8741,#8742,#8743,
#8744,#8745),.UNSPECIFIED.,.F.,.F.,(4,1,1,1,1,4),(72.2566310325652,72.7170915677583,
73.7147653826018,74.7124391974452,75.7101130122887,76.7077868271321),
 .UNSPECIFIED.);
#388=B_SPLINE_CURVE_WITH_KNOTS('',3,(#8748,#8749,#8750,#8751,#8752,#8753,
#8754,#8755,#8756),.UNSPECIFIED.,.F.,.F.,(4,1,1,1,1,1,4),(72.2566310325652,
72.263481387892,73.2611552027354,74.2588290175789,75.2565028324223,76.2541766472658,
77.2302531987677),.UNSPECIFIED.);
#389=B_SPLINE_CURVE_WITH_KNOTS('',3,(#8761,#8762,#8763,#8764,#8765,#8766,
#8767,#8768,#8769,#8770),.UNSPECIFIED.,.F.,.F.,(4,1,1,1,1,1,1,4),(65.9734457253856,
66.7310486786976,67.728722493541,68.7263963083845,69.7240701232279,70.7217439380714,
71.7194177529149,72.2566310325652),.UNSPECIFIED.);
#390=B_SPLINE_CURVE_WITH_KNOTS('',3,(#8771,#8772,#8773,#8774,#8775,#8776,
#8777,#8778,#8779,#8780),.UNSPECIFIED.,.F.,.F.,(4,1,1,1,1,1,1,4),(65.9734457253856,
66.2774384988313,67.2751123136747,68.2727861285182,69.2704599433616,70.2681337582051,
71.2658075730485,72.2566310325652),.UNSPECIFIED.);
#391=B_SPLINE_CURVE_WITH_KNOTS('',3,(#8785,#8786,#8787,#8788,#8789,#8790,
#8791,#8792,#8793,#8794,#8795),.UNSPECIFIED.,.F.,.F.,(4,1,1,1,1,1,1,1,4),
(59.6902604182061,59.7473319747934,60.7450057896369,61.7426796044803,62.7403534193238,
63.7380272341672,64.7357010490107,65.7333748638542,65.9734457253856),
 .UNSPECIFIED.);
#392=B_SPLINE_CURVE_WITH_KNOTS('',3,(#8796,#8797,#8798,#8799,#8800,#8801,
#8802,#8803,#8804,#8805),.UNSPECIFIED.,.F.,.F.,(4,1,1,1,1,1,1,4),(59.6902604182061,
60.2913956097706,61.289069424614,62.2867432394575,63.2844170543009,64.2820908691444,
65.2797646839878,65.9734457253856),.UNSPECIFIED.);
#393=B_SPLINE_CURVE_WITH_KNOTS('',3,(#8810,#8811,#8812,#8813,#8814,#8815,
#8816,#8817,#8818,#8819),.UNSPECIFIED.,.F.,.F.,(4,1,1,1,1,1,1,4),(53.4070751110265,
53.7612890857327,54.7589629005762,55.7566367154196,56.7543105302631,57.7519843451065,
58.74965815995,59.6902604182061),.UNSPECIFIED.);
#394=B_SPLINE_CURVE_WITH_KNOTS('',3,(#8820,#8821,#8822,#8823,#8824,#8825,
#8826,#8827,#8828,#8829),.UNSPECIFIED.,.F.,.F.,(4,1,1,1,1,1,1,4),(53.4070751110265,
54.3053527207099,55.3030265355533,56.3007003503968,57.2983741652402,58.2960479800837,
59.2937217949271,59.6902604182061),.UNSPECIFIED.);
#395=B_SPLINE_CURVE_WITH_KNOTS('',3,(#8834,#8835,#8836,#8837,#8838,#8839,
#8840,#8841,#8842,#8843),.UNSPECIFIED.,.F.,.F.,(4,1,1,1,1,1,1,4),(47.1238898038469,
47.775246196672,48.7729200115155,49.7705938263589,50.7682676412024,51.7659414560458,
52.7636152708893,53.4070751110265),.UNSPECIFIED.);
#396=B_SPLINE_CURVE_WITH_KNOTS('',3,(#8844,#8845,#8846,#8847,#8848,#8849,
#8850,#8851,#8852,#8853,#8854),.UNSPECIFIED.,.F.,.F.,(4,1,1,1,1,1,1,1,4),
(47.1238898038469,47.3216360168057,48.3193098316492,49.3169836464926,50.3146574613361,
51.3123312761795,52.310005091023,53.3076789058664,53.4070751110265),
 .UNSPECIFIED.);
#397=B_SPLINE_CURVE_WITH_KNOTS('',3,(#8859,#8860,#8861,#8862,#8863,#8864,
#8865,#8866,#8867,#8868),.UNSPECIFIED.,.F.,.F.,(4,1,1,1,1,1,1,4),(40.8407044966673,
41.7892033076113,42.7868771224548,43.7845509372982,44.7822247521417,45.7798985669851,
46.7775723818286,47.1238898038469),.UNSPECIFIED.);
#398=B_SPLINE_CURVE_WITH_KNOTS('',3,(#8869,#8870,#8871,#8872,#8873,#8874,
#8875,#8876,#8877,#8878),.UNSPECIFIED.,.F.,.F.,(4,1,1,1,1,1,1,4),(40.8407044966673,
41.335593127745,42.3332669425885,43.3309407574319,44.3286145722754,45.3262883871188,
46.3239622019623,47.1238898038469),.UNSPECIFIED.);
#399=B_SPLINE_CURVE_WITH_KNOTS('',3,(#8883,#8884,#8885,#8886,#8887,#8888,
#8889,#8890,#8891,#8892,#8893),.UNSPECIFIED.,.F.,.F.,(4,1,1,1,1,1,1,1,4),
(34.5575191894877,34.8054866037072,35.8031604185506,36.8008342333941,37.7985080482375,
38.796181863081,39.7938556779244,40.7915294927679,40.8407044966673),
 .UNSPECIFIED.);
#400=B_SPLINE_CURVE_WITH_KNOTS('',3,(#8894,#8895,#8896,#8897,#8898,#8899,
#8900,#8901,#8902,#8903),.UNSPECIFIED.,.F.,.F.,(4,1,1,1,1,1,1,4),(34.5575191894877,
35.3495502386843,36.3472240535278,37.3448978683712,38.3425716832147,39.3402454980581,
40.3379193129016,40.8407044966673),.UNSPECIFIED.);
#401=B_SPLINE_CURVE_WITH_KNOTS('',3,(#8908,#8909,#8910,#8911,#8912,#8913,
#8914,#8915,#8916,#8917),.UNSPECIFIED.,.F.,.F.,(4,1,1,1,1,1,1,4),(28.2743338823081,
28.8194437146465,29.8171175294899,30.8147913443334,31.8124651591768,32.8101389740203,
33.8078127888637,34.5575191894877),.UNSPECIFIED.);
#402=B_SPLINE_CURVE_WITH_KNOTS('',3,(#8918,#8919,#8920,#8921,#8922,#8923,
#8924,#8925,#8926,#8927,#8928),.UNSPECIFIED.,.F.,.F.,(4,1,1,1,1,1,1,1,4),
(28.2743338823081,28.3658335347801,29.3635073496236,30.361181164467,31.3588549793105,
32.3565287941539,33.3542026089974,34.3518764238408,34.5575191894877),
 .UNSPECIFIED.);
#403=B_SPLINE_CURVE_WITH_KNOTS('',3,(#8933,#8934,#8935,#8936,#8937,#8938,
#8939,#8940,#8941,#8942),.UNSPECIFIED.,.F.,.F.,(4,1,1,1,1,1,1,4),(21.9911485751285,
22.8334008255858,23.8310746404292,24.8287484552727,25.8264222701161,26.8240960849596,
27.821769899803,28.2743338823081),.UNSPECIFIED.);
#404=B_SPLINE_CURVE_WITH_KNOTS('',3,(#8943,#8944,#8945,#8946,#8947,#8948,
#8949,#8950,#8951,#8952),.UNSPECIFIED.,.F.,.F.,(4,1,1,1,1,1,1,4),(21.9911485751285,
22.3797906457194,23.3774644605629,24.3751382754063,25.3728120902498,26.3704859050932,
27.3681597199367,28.2743338823081),.UNSPECIFIED.);
#405=B_SPLINE_CURVE_WITH_KNOTS('',3,(#8958,#8959,#8960,#8961,#8962),
 .UNSPECIFIED.,.F.,.F.,(4,1,4),(14.3984001269718,15.3960739418153,15.7079632679489),
 .UNSPECIFIED.);
#406=B_SPLINE_CURVE_WITH_KNOTS('',3,(#8965,#8966,#8967,#8968,#8969),
 .UNSPECIFIED.,.F.,.F.,(4,1,4),(13.8759337553362,14.8520103068381,15.7079632679489),
 .UNSPECIFIED.);
#407=B_SPLINE_CURVE_WITH_KNOTS('',3,(#8971,#8972,#8973,#8974,#8975,#8976,
#8977,#8978,#8979,#8980,#8981),.UNSPECIFIED.,.F.,.F.,(4,1,1,1,1,1,1,1,4),
(15.7079632679489,15.8496841216816,16.8473579365251,17.8450317513685,18.842705566212,
19.8403793810554,20.8380531958989,21.8357270107423,21.9911485751285),
 .UNSPECIFIED.);
#408=B_SPLINE_CURVE_WITH_KNOTS('',3,(#8982,#8983,#8984,#8985,#8986,#8987,
#8988,#8989,#8990,#8991),.UNSPECIFIED.,.F.,.F.,(4,1,1,1,1,1,1,4),(15.7079632679489,
16.3937477566587,17.3914215715022,18.3890953863456,19.3867692011891,20.3844430160325,
21.382116830876,21.9911485751285),.UNSPECIFIED.);
#409=B_SPLINE_CURVE_WITH_KNOTS('',3,(#9264,#9265,#9266,#9267,#9268,#9269,
#9270,#9271,#9272,#9273,#9274,#9275,#9276,#9277,#9278,#9279,#9280,#9281,
#9282,#9283,#9284,#9285,#9286,#9287,#9288,#9289,#9290,#9291,#9292,#9293,
#9294,#9295,#9296,#9297,#9298,#9299,#9300,#9301,#9302,#9303,#9304,#9305,
#9306,#9307,#9308,#9309,#9310,#9311,#9312,#9313,#9314,#9315,#9316,#9317,
#9318,#9319,#9320,#9321,#9322,#9323,#9324,#9325,#9326,#9327,#9328,#9329,
#9330,#9331,#9332,#9333,#9334,#9335,#9336,#9337,#9338,#9339,#9340,#9341,
#9342,#9343,#9344,#9345,#9346,#9347,#9348,#9349,#9350,#9351,#9352,#9353,
#9354,#9355,#9356,#9357),.UNSPECIFIED.,.F.,.F.,(4,3,3,3,3,3,3,3,3,3,3,3,
3,3,3,3,3,3,3,3,3,3,3,3,3,3,3,3,3,3,3,4),(0.,0.0297253856296242,0.0601108027378182,
0.0895285923314871,0.115269158225947,0.120663203154239,0.150426123645478,
0.180024242366161,0.208881461646413,0.221328534043225,0.230191839641767,
0.234061656880844,0.262605657052961,0.290518670715962,0.295453119487169,
0.324405064850195,0.334115170721295,0.339546989903195,0.343311812224126,
0.371402280037358,0.399548859805574,0.427297746231078,0.438086546423522,
0.4438564739476,0.448937779695101,0.477641116182565,0.499168618548163,0.50804276641633,
0.513343558540668,0.539242379724507,0.563751125644957,0.569248610399426),
 .UNSPECIFIED.);
#410=B_SPLINE_CURVE_WITH_KNOTS('',3,(#9358,#9359,#9360,#9361,#9362,#9363,
#9364,#9365,#9366,#9367,#9368,#9369,#9370,#9371,#9372,#9373,#9374,#9375,
#9376,#9377,#9378,#9379,#9380,#9381,#9382,#9383,#9384,#9385,#9386,#9387,
#9388,#9389,#9390,#9391,#9392,#9393,#9394,#9395,#9396,#9397,#9398,#9399,
#9400,#9401,#9402,#9403,#9404,#9405,#9406,#9407,#9408,#9409,#9410,#9411,
#9412,#9413,#9414,#9415,#9416,#9417,#9418,#9419,#9420,#9421,#9422,#9423,
#9424,#9425,#9426,#9427,#9428,#9429,#9430,#9431,#9432,#9433,#9434,#9435,
#9436,#9437,#9438,#9439,#9440,#9441,#9442,#9443,#9444,#9445,#9446,#9447,
#9448,#9449,#9450,#9451,#9452,#9453,#9454),.UNSPECIFIED.,.F.,.F.,(4,3,3,
3,3,3,3,3,3,3,3,3,3,3,3,3,3,3,3,3,3,3,3,3,3,3,3,3,3,3,3,3,4),(0.,0.0253648787438216,
0.0514012503296148,0.0783340991562622,0.0901172205179204,0.0965533763871403,
0.102698976537763,0.130004344707653,0.157760279045425,0.185036219519768,
0.195822086385967,0.202205933167581,0.206455228577107,0.235058197592291,
0.263563073600605,0.266864040942794,0.294771372010393,0.305811990557415,
0.311201564685129,0.315692000115899,0.343784542768854,0.372917960011625,
0.402371202344126,0.413838480330537,0.423017273727782,0.428134361040601,
0.458199607388461,0.483702640496826,0.492128633871143,0.498168341087558,
0.529190040454739,0.56021173982192,0.566847306048046),.UNSPECIFIED.);
#411=B_SPLINE_CURVE_WITH_KNOTS('',3,(#9455,#9456,#9457,#9458,#9459,#9460,
#9461,#9462,#9463,#9464,#9465,#9466,#9467,#9468,#9469,#9470,#9471,#9472,
#9473,#9474,#9475,#9476,#9477,#9478,#9479),.UNSPECIFIED.,.F.,.F.,(4,3,3,
3,3,3,3,3,4),(-10.1321597128207,-9.9767381484345,-8.97906433359106,-7.9813905187476,
-6.98371670390416,-5.9860428890607,-4.98836907421726,-3.9906952593738,-3.84897440564114),
 .UNSPECIFIED.);
#412=B_SPLINE_CURVE_WITH_KNOTS('',3,(#9752,#9753,#9754,#9755,#9756,#9757,
#9758,#9759,#9760,#9761,#9762,#9763,#9764,#9765,#9766,#9767,#9768,#9769,
#9770,#9771,#9772,#9773,#9774,#9775,#9776,#9777,#9778,#9779,#9780,#9781,
#9782,#9783,#9784,#9785,#9786,#9787,#9788,#9789,#9790,#9791,#9792,#9793,
#9794,#9795,#9796,#9797,#9798,#9799,#9800,#9801,#9802,#9803,#9804,#9805,
#9806,#9807,#9808,#9809,#9810,#9811,#9812,#9813,#9814,#9815,#9816,#9817,
#9818,#9819,#9820,#9821,#9822,#9823,#9824,#9825,#9826,#9827,#9828,#9829,
#9830,#9831,#9832,#9833,#9834,#9835,#9836,#9837,#9838,#9839,#9840,#9841,
#9842,#9843,#9844,#9845,#9846,#9847,#9848),.UNSPECIFIED.,.F.,.F.,(4,3,3,
3,3,3,3,3,3,3,3,3,3,3,3,3,3,3,3,3,3,3,3,3,3,3,3,3,3,3,3,3,4),(0.,0.0253648724852029,
0.0514012384230764,0.0783340887380444,0.0901172107508429,0.0965533720660576,
0.102698977879582,0.130004341727049,0.157760273968556,0.185036215712122,
0.195822085350035,0.202205931968829,0.206455227843058,0.235058195828899,
0.263563073798338,0.26686404094282,0.294771375027874,0.305811996926419,
0.311201630318074,0.31569201086916,0.343784558171023,0.372917977567861,
0.402371220433395,0.413838515963309,0.423017671022353,0.428134408783598,
0.458199656551482,0.483702677369108,0.492128800036471,0.498168345990172,
0.529190042906079,0.560211739821985,0.56684730604811),.UNSPECIFIED.);
#413=B_SPLINE_CURVE_WITH_KNOTS('',3,(#9849,#9850,#9851,#9852,#9853,#9854,
#9855,#9856,#9857,#9858,#9859,#9860,#9861,#9862,#9863,#9864,#9865,#9866,
#9867,#9868,#9869,#9870),.UNSPECIFIED.,.F.,.F.,(4,3,3,3,3,3,3,4),(7.59274844815666,
7.9813905187476,8.97906433359105,9.97673814843451,10.974411963278,11.9720857781214,
12.9697595929649,13.8759337553362),.UNSPECIFIED.);
#414=B_SPLINE_CURVE_WITH_KNOTS('',3,(#9871,#9872,#9873,#9874,#9875,#9876,
#9877,#9878,#9879,#9880,#9881,#9882,#9883,#9884,#9885,#9886,#9887,#9888,
#9889,#9890,#9891,#9892,#9893,#9894,#9895,#9896,#9897,#9898,#9899,#9900,
#9901,#9902,#9903,#9904,#9905,#9906,#9907,#9908,#9909,#9910,#9911,#9912,
#9913,#9914,#9915,#9916,#9917,#9918,#9919,#9920,#9921,#9922,#9923,#9924,
#9925,#9926,#9927,#9928,#9929,#9930,#9931,#9932,#9933,#9934,#9935,#9936,
#9937,#9938,#9939,#9940,#9941,#9942,#9943,#9944,#9945,#9946,#9947,#9948,
#9949,#9950,#9951,#9952,#9953,#9954,#9955,#9956,#9957,#9958,#9959,#9960,
#9961,#9962,#9963,#9964),.UNSPECIFIED.,.F.,.F.,(4,3,3,3,3,3,3,3,3,3,3,3,
3,3,3,3,3,3,3,3,3,3,3,3,3,3,3,3,3,3,3,4),(0.,0.0297253803932464,0.0601107949195137,
0.0895285854904694,0.115269152240056,0.120663201907019,0.150426122369489,
0.180024242551286,0.208881461785255,0.221328534890279,0.230191850972631,
0.234061673089794,0.262605674713976,0.290518689511932,0.295453119487159,
0.324405064607358,0.334115171284016,0.339546990350236,0.343311812881693,
0.371402280552886,0.399548860319871,0.427297747957366,0.43808655063386,
0.443856478069222,0.448937779896069,0.477641116333293,0.499168618661212,
0.508042768434368,0.513343559316224,0.53924238350147,0.563751125644968,
0.569248610399442),.UNSPECIFIED.);
#415=B_SPLINE_CURVE_WITH_KNOTS('',3,(#9974,#9975,#9976,#9977,#9978,#9979,
#9980,#9981,#9982,#9983,#9984,#9985,#9986,#9987,#9988,#9989,#9990,#9991,
#9992,#9993,#9994,#9995,#9996,#9997,#9998,#9999,#10000,#10001,#10002,#10003,
#10004,#10005,#10006,#10007,#10008,#10009,#10010,#10011,#10012,#10013,#10014,
#10015,#10016,#10017,#10018,#10019,#10020,#10021,#10022,#10023,#10024,#10025,
#10026,#10027,#10028,#10029,#10030,#10031,#10032,#10033,#10034,#10035,#10036,
#10037,#10038,#10039,#10040,#10041,#10042,#10043,#10044,#10045,#10046,#10047,
#10048,#10049,#10050,#10051,#10052,#10053,#10054,#10055,#10056,#10057,#10058,
#10059,#10060,#10061,#10062,#10063,#10064,#10065,#10066,#10067,#10068,#10069,
#10070),.UNSPECIFIED.,.F.,.F.,(4,3,3,3,3,3,3,3,3,3,3,3,3,3,3,3,3,3,3,3,
3,3,3,3,3,3,3,3,3,3,3,3,4),(0.,0.0253648605053273,0.0514012156305792,0.0783340687946069,
0.0901171920538689,0.0965533637916206,0.102698980421147,0.130004335995597,
0.157760264221757,0.185036208402018,0.195822083362881,0.202205929681762,
0.206455226436585,0.235058192455082,0.263563074173201,0.2668640409428,0.294771380802971,
0.305812009113333,0.311201755151532,0.315692031327867,0.343784587536137,
0.372918011054392,0.402371254938888,0.413838583941099,0.4230184291352,0.428134500012189,
0.458199750478009,0.483702747813993,0.492129117528397,0.498168355355325,
0.529190047588635,0.560211739821945,0.566847306048074),.UNSPECIFIED.);
#416=B_SPLINE_CURVE_WITH_KNOTS('',3,(#10071,#10072,#10073,#10074,#10075,
#10076,#10077,#10078,#10079,#10080,#10081,#10082,#10083,#10084,#10085,#10086,
#10087,#10088,#10089,#10090,#10091,#10092,#10093,#10094,#10095,#10096,#10097,
#10098,#10099,#10100,#10101,#10102,#10103,#10104,#10105,#10106,#10107,#10108,
#10109,#10110,#10111,#10112,#10113,#10114,#10115,#10116,#10117,#10118,#10119,
#10120,#10121,#10122,#10123,#10124,#10125,#10126,#10127,#10128,#10129,#10130,
#10131,#10132,#10133,#10134,#10135,#10136,#10137,#10138,#10139,#10140,#10141,
#10142,#10143,#10144,#10145,#10146,#10147,#10148,#10149,#10150,#10151,#10152,
#10153,#10154,#10155,#10156,#10157,#10158,#10159,#10160,#10161,#10162,#10163,
#10164),.UNSPECIFIED.,.F.,.F.,(4,3,3,3,3,3,3,3,3,3,3,3,3,3,3,3,3,3,3,3,
3,3,3,3,3,3,3,3,3,3,3,4),(0.,0.0297254323827744,0.0601108725400646,0.0895286534084515,
0.11526921166829,0.12066321428879,0.150426135046203,0.180024240717284,0.208881460409753,
0.221328526477776,0.230191738437716,0.234061511334529,0.262605498546548,
0.290518502067642,0.29545311948716,0.324405067020953,0.334115165693271,
0.339546985526679,0.343311805029728,0.371402274101902,0.399548853885078,
0.42729772947452,0.438086506007797,0.443856434974185,0.44893777735014,0.477641114423841,
0.499168617229116,0.508042746133096,0.513343551251566,0.539242345608596,
0.563751125644942,0.569248610399418),.UNSPECIFIED.);
#417=B_SPLINE_CURVE_WITH_KNOTS('',3,(#10165,#10166,#10167,#10168,#10169,
#10170,#10171,#10172,#10173,#10174,#10175,#10176,#10177,#10178,#10179,#10180,
#10181,#10182,#10183,#10184,#10185,#10186,#10187,#10188,#10189,#10190,#10191,
#10192,#10193,#10194,#10195,#10196,#10197,#10198,#10199,#10200,#10201,#10202,
#10203,#10204,#10205,#10206,#10207,#10208,#10209,#10210,#10211,#10212,#10213,
#10214,#10215,#10216,#10217,#10218,#10219,#10220,#10221,#10222,#10223,#10224,
#10225,#10226,#10227,#10228,#10229,#10230,#10231,#10232,#10233,#10234,#10235,
#10236,#10237,#10238,#10239,#10240,#10241,#10242,#10243,#10244,#10245,#10246,
#10247,#10248,#10249,#10250,#10251,#10252,#10253,#10254,#10255,#10256,#10257,
#10258,#10259,#10260,#10261),.UNSPECIFIED.,.F.,.F.,(4,3,3,3,3,3,3,3,3,3,
3,3,3,3,3,3,3,3,3,3,3,3,3,3,3,3,3,3,3,3,3,3,4),(0.,0.0253648987606154,0.0514012884108024,
0.0783341324773016,0.0901172517563951,0.0965533902110582,0.102698972275023,
0.130004354267608,0.157760295311984,0.185036231719687,0.195822089703329,
0.202205936992556,0.206455230916444,0.235058203214103,0.263563072953794,
0.266864040942797,0.294771362359164,0.305811970189412,0.311201355676537,
0.315691965877597,0.343784493654311,0.372917904009451,0.402371144638991,
0.413838366652747,0.423016006622453,0.42813420907177,0.458199450904524,
0.483702523133876,0.492128105008987,0.498168325925378,0.529190032873656,
0.560211739821933,0.566847306048061),.UNSPECIFIED.);
#418=B_SPLINE_CURVE_WITH_KNOTS('',3,(#10262,#10263,#10264,#10265,#10266,
#10267,#10268,#10269,#10270,#10271,#10272,#10273,#10274,#10275,#10276,#10277,
#10278,#10279,#10280,#10281,#10282,#10283,#10284,#10285,#10286,#10287,#10288,
#10289,#10290,#10291,#10292,#10293,#10294,#10295,#10296,#10297,#10298,#10299,
#10300,#10301,#10302,#10303,#10304,#10305,#10306,#10307,#10308,#10309,#10310,
#10311,#10312,#10313,#10314,#10315,#10316,#10317,#10318,#10319,#10320,#10321,
#10322,#10323,#10324,#10325,#10326,#10327,#10328,#10329,#10330,#10331,#10332,
#10333,#10334,#10335,#10336,#10337,#10338,#10339,#10340,#10341,#10342,#10343,
#10344,#10345,#10346,#10347,#10348,#10349,#10350,#10351,#10352,#10353,#10354,
#10355),.UNSPECIFIED.,.F.,.F.,(4,3,3,3,3,3,3,3,3,3,3,3,3,3,3,3,3,3,3,3,
3,3,3,3,3,3,3,3,3,3,3,4),(0.,0.0297253962397254,0.0601108185791267,0.0895286061926336,
0.115269170354452,0.12066320568266,0.150426126236148,0.180024241996468,
0.208881461369146,0.221328532330586,0.230191816729447,0.23406162386096,
0.262605621092836,0.290518632453638,0.295453119487182,0.324405065342412,
0.334115169579262,0.339546988882028,0.343311810500951,0.371402278599766,
0.399548858373274,0.427297742341304,0.438086537068835,0.443856464964634,
0.448937779125463,0.477641115755344,0.499168618227755,0.508042761654416,
0.513343556861467,0.539242371960185,0.563751125644987,0.569248610399463),
 .UNSPECIFIED.);
#419=B_SPLINE_CURVE_WITH_KNOTS('',3,(#10356,#10357,#10358,#10359,#10360,
#10361,#10362,#10363,#10364,#10365,#10366,#10367,#10368,#10369,#10370,#10371,
#10372,#10373,#10374,#10375,#10376,#10377,#10378,#10379,#10380,#10381,#10382,
#10383,#10384,#10385,#10386,#10387,#10388,#10389,#10390,#10391,#10392,#10393,
#10394,#10395,#10396,#10397,#10398,#10399,#10400,#10401,#10402,#10403,#10404,
#10405,#10406,#10407,#10408,#10409,#10410,#10411,#10412,#10413,#10414,#10415,
#10416,#10417,#10418,#10419,#10420,#10421,#10422,#10423,#10424,#10425,#10426,
#10427,#10428,#10429,#10430,#10431,#10432,#10433,#10434,#10435,#10436,#10437,
#10438,#10439,#10440,#10441,#10442,#10443,#10444,#10445,#10446,#10447,#10448,
#10449,#10450,#10451,#10452),.UNSPECIFIED.,.F.,.F.,(4,3,3,3,3,3,3,3,3,3,
3,3,3,3,3,3,3,3,3,3,3,3,3,3,3,3,3,3,3,3,3,3,4),(0.,0.025364844042126,0.0514011843088595,
0.0783340413881027,0.0901171663602716,0.0965533524230185,0.102698983918303,
0.130004328122858,0.157760250831759,0.185036198359521,0.195822080632133,
0.20220592653402,0.206455224516067,0.235058187831454,0.263563074702486,
0.266864040942805,0.294771388738814,0.30581202586054,0.311201927094549,
0.315692059513443,0.343784627954795,0.372918057137183,0.402371302422366,
0.413838677482968,0.423019472683294,0.428134625857437,0.458199880044474,
0.483702844988851,0.492129555524298,0.498168368529568,0.529190054175775,
0.560211739821982,0.566847306048111),.UNSPECIFIED.);
#420=B_SPLINE_CURVE_WITH_KNOTS('',3,(#10453,#10454,#10455,#10456,#10457,
#10458,#10459,#10460,#10461,#10462,#10463,#10464,#10465,#10466,#10467,#10468,
#10469,#10470,#10471,#10472,#10473,#10474,#10475,#10476,#10477,#10478,#10479,
#10480,#10481,#10482,#10483,#10484,#10485,#10486,#10487,#10488,#10489,#10490,
#10491,#10492,#10493,#10494,#10495,#10496,#10497,#10498,#10499,#10500,#10501,
#10502,#10503,#10504,#10505,#10506,#10507,#10508,#10509,#10510,#10511,#10512,
#10513,#10514,#10515,#10516,#10517,#10518,#10519,#10520,#10521,#10522,#10523,
#10524,#10525,#10526,#10527,#10528,#10529,#10530,#10531,#10532,#10533,#10534,
#10535,#10536,#10537,#10538,#10539,#10540,#10541,#10542,#10543,#10544,#10545,
#10546),.UNSPECIFIED.,.F.,.F.,(4,3,3,3,3,3,3,3,3,3,3,3,3,3,3,3,3,3,3,3,
3,3,3,3,3,3,3,3,3,3,3,4),(0.,0.0297254135725658,0.0601108444573347,0.0895286288360644,
0.115269190167453,0.120663209818937,0.15042613047052,0.180024241393071,
0.208881460916596,0.221328529533058,0.230191779298948,0.234061570055621,
0.262605562480418,0.290518570080715,0.295453119487172,0.324405066148158,
0.334115167717825,0.339546987280336,0.343311807892538,0.371402276458584,
0.399548856237476,0.42729773618933,0.438086522212006,0.443856450609684,
0.448937778272206,0.477641115115396,0.499168617747789,0.508042754204043,
0.513343554169974,0.539242359324933,0.563751125644967,0.569248610399445),
 .UNSPECIFIED.);
#421=B_SPLINE_CURVE_WITH_KNOTS('',3,(#10548,#10549,#10550,#10551,#10552,
#10553,#10554,#10555,#10556,#10557,#10558),.UNSPECIFIED.,.F.,.F.,(4,1,1,
1,1,1,1,1,4),(15.7079632679489,15.8496841216816,16.847357936525,17.8450317513685,
18.8427055662119,19.8403793810554,20.8380531958989,21.8357270107423,21.9911485751285),
 .UNSPECIFIED.);
#422=B_SPLINE_CURVE_WITH_KNOTS('',3,(#10559,#10560,#10561,#10562,#10563,
#10564,#10565,#10566,#10567,#10568),.UNSPECIFIED.,.F.,.F.,(4,1,1,1,1,1,
1,4),(15.7079632679489,16.3937477566587,17.3914215715022,18.3890953863456,
19.3867692011891,20.3844430160325,21.382116830876,21.9911485751285),
 .UNSPECIFIED.);
#423=B_SPLINE_CURVE_WITH_KNOTS('',3,(#10841,#10842,#10843,#10844,#10845,
#10846,#10847,#10848,#10849,#10850,#10851,#10852,#10853,#10854,#10855,#10856,
#10857,#10858,#10859,#10860,#10861,#10862,#10863,#10864,#10865,#10866,#10867,
#10868,#10869,#10870,#10871,#10872,#10873,#10874,#10875,#10876,#10877,#10878,
#10879,#10880,#10881,#10882,#10883,#10884,#10885,#10886,#10887,#10888,#10889,
#10890,#10891,#10892,#10893,#10894,#10895,#10896,#10897,#10898,#10899,#10900,
#10901,#10902,#10903,#10904,#10905,#10906,#10907,#10908,#10909,#10910,#10911,
#10912,#10913,#10914,#10915,#10916,#10917,#10918,#10919,#10920,#10921,#10922,
#10923,#10924,#10925,#10926,#10927,#10928,#10929,#10930,#10931,#10932,#10933,
#10934),.UNSPECIFIED.,.F.,.F.,(4,3,3,3,3,3,3,3,3,3,3,3,3,3,3,3,3,3,3,3,
3,3,3,3,3,3,3,3,3,3,3,4),(0.,0.0297253703679347,0.0601107799498536,0.0895285723920194,
0.115269140778915,0.120663199497391,0.150426119902105,0.180024242882666,
0.208881462033794,0.221328536492063,0.230191872423422,0.234061703914739,
0.262605708325631,0.290518725301924,0.29545311948718,0.32440506413479,0.334115172344466,
0.339546991246465,0.343311814329514,0.37140228172866,0.399548861491339,
0.427297751445956,0.438086559078568,0.443856486243239,0.448937780382051,
0.477641116697784,0.499168618934584,0.508042772723187,0.513343560868865,
0.539242390799467,0.563751125644983,0.569248610399456),.UNSPECIFIED.);
#424=B_SPLINE_CURVE_WITH_KNOTS('',3,(#10935,#10936,#10937,#10938,#10939,
#10940,#10941,#10942,#10943,#10944,#10945,#10946,#10947,#10948,#10949,#10950,
#10951,#10952,#10953,#10954,#10955,#10956,#10957,#10958,#10959),
 .UNSPECIFIED.,.F.,.F.,(4,3,3,3,3,3,3,3,4),(-10.1321597128207,-9.97673814843451,
-8.97906433359106,-7.98139051874761,-6.98371670390416,-5.98604288906071,
-4.98836907421726,-3.9906952593738,-3.84897440564114),.UNSPECIFIED.);
#425=B_SPLINE_CURVE_WITH_KNOTS('',3,(#11232,#11233,#11234,#11235,#11236,
#11237,#11238,#11239,#11240,#11241,#11242,#11243,#11244,#11245,#11246,#11247,
#11248,#11249,#11250,#11251,#11252,#11253,#11254,#11255,#11256,#11257,#11258,
#11259,#11260,#11261,#11262,#11263,#11264,#11265,#11266,#11267,#11268,#11269,
#11270,#11271,#11272,#11273,#11274,#11275,#11276,#11277,#11278,#11279,#11280,
#11281,#11282,#11283,#11284,#11285,#11286,#11287,#11288,#11289,#11290,#11291,
#11292,#11293,#11294,#11295,#11296,#11297,#11298,#11299,#11300,#11301,#11302,
#11303,#11304,#11305,#11306,#11307,#11308,#11309,#11310,#11311,#11312,#11313,
#11314,#11315,#11316,#11317,#11318,#11319,#11320,#11321,#11322,#11323,#11324,
#11325,#11326,#11327,#11328),.UNSPECIFIED.,.F.,.F.,(4,3,3,3,3,3,3,3,3,3,
3,3,3,3,3,3,3,3,3,3,3,3,3,3,3,3,3,3,3,3,3,3,4),(0.,0.0253649346248504,0.0514013566484054,
0.0783341921852065,0.090117307732557,0.0965534149831339,0.102698964686601,
0.130004371440625,0.157760324498296,0.185036253609426,0.195822095654156,
0.202205943841528,0.2064552351094,0.235058213296301,0.263563071795369,0.266864040942814,
0.294771345060892,0.305811933683324,0.311200980890666,0.315691904514554,
0.343784405626614,0.372917803637586,0.402371041212361,0.413838162909138,
0.423013737084902,0.428133938024777,0.458199171791025,0.483702313798766,
0.492127161867958,0.498168299793874,0.529190019807931,0.560211739821988,
0.566847306048107),.UNSPECIFIED.);
#426=B_SPLINE_CURVE_WITH_KNOTS('',3,(#11329,#11330,#11331,#11332,#11333,
#11334,#11335,#11336,#11337,#11338,#11339,#11340,#11341,#11342,#11343,#11344,
#11345,#11346,#11347,#11348,#11349,#11350),.UNSPECIFIED.,.F.,.F.,(4,3,3,
3,3,3,3,4),(7.59274844815666,7.98139051874761,8.97906433359106,9.97673814843451,
10.974411963278,11.9720857781214,12.9697595929649,13.8759337553362),
 .UNSPECIFIED.);
#427=B_SPLINE_CURVE_WITH_KNOTS('',3,(#11352,#11353,#11354,#11355,#11356,
#11357,#11358,#11359,#11360,#11361,#11362),.UNSPECIFIED.,.F.,.F.,(4,1,1,
1,1,1,1,1,4),(15.7079632679489,15.8496841216816,16.847357936525,17.8450317513685,
18.8427055662119,19.8403793810554,20.8380531958988,21.8357270107423,21.9911485751285),
 .UNSPECIFIED.);
#428=B_SPLINE_CURVE_WITH_KNOTS('',3,(#11363,#11364,#11365,#11366,#11367,
#11368,#11369,#11370,#11371,#11372),.UNSPECIFIED.,.F.,.F.,(4,1,1,1,1,1,
1,4),(15.7079632679489,16.3937477566587,17.3914215715022,18.3890953863456,
19.3867692011891,20.3844430160325,21.382116830876,21.9911485751285),
 .UNSPECIFIED.);
#429=B_SPLINE_CURVE_WITH_KNOTS('',3,(#11645,#11646,#11647,#11648,#11649,
#11650,#11651,#11652,#11653,#11654,#11655,#11656,#11657,#11658,#11659,#11660,
#11661,#11662,#11663,#11664,#11665,#11666,#11667,#11668,#11669,#11670,#11671,
#11672,#11673,#11674,#11675,#11676,#11677,#11678,#11679,#11680,#11681,#11682,
#11683,#11684,#11685,#11686,#11687,#11688,#11689,#11690,#11691,#11692,#11693,
#11694,#11695,#11696,#11697,#11698,#11699,#11700,#11701,#11702,#11703,#11704,
#11705,#11706,#11707,#11708,#11709,#11710,#11711,#11712,#11713,#11714,#11715,
#11716,#11717,#11718,#11719,#11720,#11721,#11722,#11723,#11724,#11725,#11726,
#11727,#11728,#11729,#11730,#11731,#11732,#11733,#11734,#11735,#11736,#11737,
#11738),.UNSPECIFIED.,.F.,.F.,(4,3,3,3,3,3,3,3,3,3,3,3,3,3,3,3,3,3,3,3,
3,3,3,3,3,3,3,3,3,3,3,4),(0.,0.0297254023740782,0.0601108277330677,0.0895286142023326,
0.115269177362939,0.120663207133914,0.15042612772287,0.180024241772488,
0.208881461201163,0.221328531331202,0.230191803363959,0.234061604650791,
0.262605600181984,0.290518610215652,0.295453119487186,0.324405065627094,
0.334115168920554,0.339546988327522,0.343311809571304,0.371402277835618,
0.399548857610104,0.427297740159933,0.438086531802328,0.443856459882809,
0.448937778846684,0.477641115546252,0.499168618070928,0.508042759111529,
0.513343555924621,0.539242367504077,0.563751125644955,0.569248610399431),
 .UNSPECIFIED.);
#430=B_SPLINE_CURVE_WITH_KNOTS('',3,(#11739,#11740,#11741,#11742,#11743,
#11744,#11745,#11746,#11747,#11748,#11749,#11750,#11751,#11752,#11753,#11754,
#11755,#11756,#11757,#11758,#11759,#11760,#11761,#11762,#11763),
 .UNSPECIFIED.,.F.,.F.,(4,3,3,3,3,3,3,3,4),(-10.1321597128207,-9.97673814843451,
-8.97906433359106,-7.9813905187476,-6.98371670390416,-5.98604288906071,
-4.98836907421726,-3.99069525937381,-3.84897440564115),.UNSPECIFIED.);
#431=B_SPLINE_CURVE_WITH_KNOTS('',3,(#12036,#12037,#12038,#12039,#12040,
#12041,#12042,#12043,#12044,#12045,#12046,#12047,#12048,#12049,#12050,#12051,
#12052,#12053,#12054,#12055,#12056,#12057,#12058,#12059,#12060,#12061,#12062,
#12063,#12064,#12065,#12066,#12067,#12068,#12069,#12070,#12071,#12072,#12073,
#12074,#12075,#12076,#12077,#12078,#12079,#12080,#12081,#12082,#12083,#12084,
#12085,#12086,#12087,#12088,#12089,#12090,#12091,#12092,#12093,#12094,#12095,
#12096,#12097,#12098,#12099,#12100,#12101,#12102,#12103,#12104,#12105,#12106,
#12107,#12108,#12109,#12110,#12111,#12112,#12113,#12114,#12115,#12116,#12117,
#12118,#12119,#12120,#12121,#12122,#12123,#12124,#12125,#12126,#12127,#12128,
#12129,#12130,#12131,#12132),.UNSPECIFIED.,.F.,.F.,(4,3,3,3,3,3,3,3,3,3,
3,3,3,3,3,3,3,3,3,3,3,3,3,3,3,3,3,3,3,3,3,3,4),(0.,0.0253648914275516,0.0514012744616646,
0.078334120271809,0.0901172403137471,0.0965533851472873,0.102698973861186,
0.130004350789599,0.157760289377991,0.185036227269198,0.195822088492465,
0.202205935589398,0.206455229962407,0.235058201053358,0.263563073088682,
0.26686404094282,0.294771365897737,0.305811977656062,0.311201432434786,
0.315691978449507,0.343784511677691,0.37291792455713,0.402371165813427,
0.413838408362615,0.423016471455126,0.42813426476668,0.458199508244744,
0.483702566139053,0.492128298799099,0.49816833135269,0.529190035587335,
0.560211739821979,0.566847306048113),.UNSPECIFIED.);
#432=B_SPLINE_CURVE_WITH_KNOTS('',3,(#12133,#12134,#12135,#12136,#12137,
#12138,#12139,#12140,#12141,#12142,#12143,#12144,#12145,#12146,#12147,#12148,
#12149,#12150,#12151,#12152,#12153,#12154),.UNSPECIFIED.,.F.,.F.,(4,3,3,
3,3,3,3,4),(7.59274844815666,7.98139051874761,8.97906433359107,9.97673814843452,
10.974411963278,11.9720857781214,12.9697595929649,13.8759337553362),
 .UNSPECIFIED.);
#433=B_SPLINE_CURVE_WITH_KNOTS('',3,(#12156,#12157,#12158,#12159,#12160,
#12161,#12162,#12163,#12164,#12165,#12166),.UNSPECIFIED.,.F.,.F.,(4,1,1,
1,1,1,1,1,4),(15.7079632679489,15.8496841216816,16.8473579365251,17.8450317513685,
18.842705566212,19.8403793810554,20.8380531958989,21.8357270107423,21.9911485751285),
 .UNSPECIFIED.);
#434=B_SPLINE_CURVE_WITH_KNOTS('',3,(#12167,#12168,#12169,#12170,#12171,
#12172,#12173,#12174,#12175,#12176),.UNSPECIFIED.,.F.,.F.,(4,1,1,1,1,1,
1,4),(15.7079632679489,16.3937477566587,17.3914215715022,18.3890953863456,
19.3867692011891,20.3844430160325,21.382116830876,21.9911485751285),
 .UNSPECIFIED.);
#435=B_SPLINE_CURVE_WITH_KNOTS('',3,(#12449,#12450,#12451,#12452,#12453,
#12454,#12455,#12456,#12457,#12458,#12459,#12460,#12461,#12462,#12463,#12464,
#12465,#12466,#12467,#12468,#12469,#12470,#12471,#12472,#12473,#12474,#12475,
#12476,#12477,#12478,#12479,#12480,#12481,#12482,#12483,#12484,#12485,#12486,
#12487,#12488,#12489,#12490,#12491,#12492,#12493,#12494,#12495,#12496,#12497,
#12498,#12499,#12500,#12501,#12502,#12503,#12504,#12505,#12506,#12507,#12508,
#12509,#12510,#12511,#12512,#12513,#12514,#12515,#12516,#12517,#12518,#12519,
#12520,#12521,#12522,#12523,#12524,#12525,#12526,#12527,#12528,#12529,#12530,
#12531,#12532,#12533,#12534,#12535,#12536,#12537,#12538,#12539,#12540,#12541,
#12542),.UNSPECIFIED.,.F.,.F.,(4,3,3,3,3,3,3,3,3,3,3,3,3,3,3,3,3,3,3,3,
3,3,3,3,3,3,3,3,3,3,3,4),(0.,0.029725356595138,0.0601107593868406,0.0895285543993829,
0.115269125035357,0.12066319618678,0.150426116509258,0.180024243330567,
0.20888146236972,0.221328538686106,0.230191901801689,0.234061746102067,
0.262605754332067,0.290518774304223,0.295453119487179,0.324405063500147,
0.334115173835696,0.339546992466191,0.343311816416088,0.37140228344413,
0.399548863199563,0.427297756337497,0.438086570890066,0.443856497633085,
0.448937781098459,0.477641117235086,0.499168619337557,0.508042778795357,
0.513343563033152,0.539242400853845,0.563751125644967,0.569248610399444),
 .UNSPECIFIED.);
#436=B_SPLINE_CURVE_WITH_KNOTS('',3,(#12543,#12544,#12545,#12546,#12547,
#12548,#12549,#12550,#12551,#12552,#12553,#12554,#12555,#12556,#12557,#12558,
#12559,#12560,#12561,#12562,#12563,#12564,#12565,#12566,#12567),
 .UNSPECIFIED.,.F.,.F.,(4,3,3,3,3,3,3,3,4),(-10.1321597128207,-9.97673814843451,
-8.97906433359106,-7.98139051874761,-6.98371670390416,-5.98604288906071,
-4.98836907421726,-3.99069525937381,-3.84897440564113),.UNSPECIFIED.);
#437=B_SPLINE_CURVE_WITH_KNOTS('',3,(#12840,#12841,#12842,#12843,#12844,
#12845,#12846,#12847,#12848,#12849,#12850,#12851,#12852,#12853,#12854,#12855,
#12856,#12857,#12858,#12859,#12860,#12861,#12862,#12863,#12864,#12865,#12866,
#12867,#12868,#12869,#12870,#12871,#12872,#12873,#12874,#12875,#12876,#12877,
#12878,#12879,#12880,#12881,#12882,#12883,#12884,#12885,#12886,#12887,#12888,
#12889,#12890,#12891,#12892,#12893,#12894,#12895,#12896,#12897,#12898,#12899,
#12900,#12901,#12902,#12903,#12904,#12905,#12906,#12907,#12908,#12909,#12910,
#12911,#12912,#12913,#12914,#12915,#12916,#12917,#12918,#12919,#12920,#12921,
#12922,#12923,#12924,#12925,#12926,#12927,#12928,#12929,#12930,#12931,#12932,
#12933,#12934,#12935,#12936),.UNSPECIFIED.,.F.,.F.,(4,3,3,3,3,3,3,3,3,3,
3,3,3,3,3,3,3,3,3,3,3,3,3,3,3,3,3,3,3,3,3,3,4),(0.,0.0253649121453671,0.0514013138739685,
0.0783341547575759,0.0901172726441542,0.0965533994556431,0.102698969500997,
0.130004360735148,0.157760306262492,0.185036239932576,0.195822091936498,
0.202205939549384,0.206455232492389,0.235058206978254,0.263563072530515,
0.266864040942828,0.294771355900332,0.305811956558916,0.311201215703461,
0.315691942956057,0.343784460775633,0.372917866524038,0.40237110601464,
0.413838290565183,0.423015158860743,0.42813410765337,0.458199346461555,
0.48370244480167,0.492127752073996,0.498168316004108,0.529190027913061,
0.560211739822014,0.566847306048133),.UNSPECIFIED.);
#438=B_SPLINE_CURVE_WITH_KNOTS('',3,(#12937,#12938,#12939,#12940,#12941,
#12942,#12943,#12944,#12945,#12946,#12947,#12948,#12949,#12950,#12951,#12952,
#12953,#12954,#12955,#12956,#12957,#12958),.UNSPECIFIED.,.F.,.F.,(4,3,3,
3,3,3,3,4),(7.59274844815664,7.98139051874761,8.97906433359106,9.97673814843451,
10.974411963278,11.9720857781214,12.9697595929649,13.8759337553362),
 .UNSPECIFIED.);
#446=SHAPE_REPRESENTATION_RELATIONSHIP('SRR','None',#13335,#462);
#462=ADVANCED_BREP_SHAPE_REPRESENTATION('',(#494),#13222);
#478=STYLED_ITEM('',(#13417),#494);
#494=MANIFOLD_SOLID_BREP('Body1',#4158);
#531=FACE_BOUND('',#1044,.T.);
#532=FACE_BOUND('',#1045,.T.);
#533=FACE_BOUND('',#1046,.T.);
#534=FACE_BOUND('',#1047,.T.);
#535=FACE_BOUND('',#1066,.T.);
#536=FACE_BOUND('',#1067,.T.);
#537=FACE_BOUND('',#1068,.T.);
#538=FACE_BOUND('',#1069,.T.);
#602=PLANE('',#4584);
#603=PLANE('',#4592);
#604=PLANE('',#4593);
#605=PLANE('',#4594);
#606=PLANE('',#4595);
#607=PLANE('',#4596);
#711=FACE_OUTER_BOUND('',#960,.T.);
#712=FACE_OUTER_BOUND('',#961,.T.);
#713=FACE_OUTER_BOUND('',#962,.T.);
#714=FACE_OUTER_BOUND('',#963,.T.);
#715=FACE_OUTER_BOUND('',#964,.T.);
#716=FACE_OUTER_BOUND('',#965,.T.);
#717=FACE_OUTER_BOUND('',#966,.T.);
#718=FACE_OUTER_BOUND('',#967,.T.);
#719=FACE_OUTER_BOUND('',#968,.T.);
#720=FACE_OUTER_BOUND('',#969,.T.);
#721=FACE_OUTER_BOUND('',#970,.T.);
#722=FACE_OUTER_BOUND('',#971,.T.);
#723=FACE_OUTER_BOUND('',#972,.T.);
#724=FACE_OUTER_BOUND('',#973,.T.);
#725=FACE_OUTER_BOUND('',#974,.T.);
#726=FACE_OUTER_BOUND('',#975,.T.);
#727=FACE_OUTER_BOUND('',#976,.T.);
#728=FACE_OUTER_BOUND('',#977,.T.);
#729=FACE_OUTER_BOUND('',#978,.T.);
#730=FACE_OUTER_BOUND('',#979,.T.);
#731=FACE_OUTER_BOUND('',#980,.T.);
#732=FACE_OUTER_BOUND('',#981,.T.);
#733=FACE_OUTER_BOUND('',#982,.T.);
#734=FACE_OUTER_BOUND('',#983,.T.);
#735=FACE_OUTER_BOUND('',#984,.T.);
#736=FACE_OUTER_BOUND('',#985,.T.);
#737=FACE_OUTER_BOUND('',#986,.T.);
#738=FACE_OUTER_BOUND('',#987,.T.);
#739=FACE_OUTER_BOUND('',#988,.T.);
#740=FACE_OUTER_BOUND('',#989,.T.);
#741=FACE_OUTER_BOUND('',#990,.T.);
#742=FACE_OUTER_BOUND('',#991,.T.);
#743=FACE_OUTER_BOUND('',#992,.T.);
#744=FACE_OUTER_BOUND('',#993,.T.);
#745=FACE_OUTER_BOUND('',#994,.T.);
#746=FACE_OUTER_BOUND('',#995,.T.);
#747=FACE_OUTER_BOUND('',#996,.T.);
#748=FACE_OUTER_BOUND('',#997,.T.);
#749=FACE_OUTER_BOUND('',#998,.T.);
#750=FACE_OUTER_BOUND('',#999,.T.);
#751=FACE_OUTER_BOUND('',#1000,.T.);
#752=FACE_OUTER_BOUND('',#1001,.T.);
#753=FACE_OUTER_BOUND('',#1002,.T.);
#754=FACE_OUTER_BOUND('',#1003,.T.);
#755=FACE_OUTER_BOUND('',#1004,.T.);
#756=FACE_OUTER_BOUND('',#1005,.T.);
#757=FACE_OUTER_BOUND('',#1006,.T.);
#758=FACE_OUTER_BOUND('',#1007,.T.);
#759=FACE_OUTER_BOUND('',#1008,.T.);
#760=FACE_OUTER_BOUND('',#1009,.T.);
#761=FACE_OUTER_BOUND('',#1010,.T.);
#762=FACE_OUTER_BOUND('',#1011,.T.);
#763=FACE_OUTER_BOUND('',#1012,.T.);
#764=FACE_OUTER_BOUND('',#1013,.T.);
#765=FACE_OUTER_BOUND('',#1014,.T.);
#766=FACE_OUTER_BOUND('',#1015,.T.);
#767=FACE_OUTER_BOUND('',#1016,.T.);
#768=FACE_OUTER_BOUND('',#1017,.T.);
#769=FACE_OUTER_BOUND('',#1018,.T.);
#770=FACE_OUTER_BOUND('',#1019,.T.);
#771=FACE_OUTER_BOUND('',#1020,.T.);
#772=FACE_OUTER_BOUND('',#1021,.T.);
#773=FACE_OUTER_BOUND('',#1022,.T.);
#774=FACE_OUTER_BOUND('',#1023,.T.);
#775=FACE_OUTER_BOUND('',#1024,.T.);
#776=FACE_OUTER_BOUND('',#1025,.T.);
#777=FACE_OUTER_BOUND('',#1026,.T.);
#778=FACE_OUTER_BOUND('',#1027,.T.);
#779=FACE_OUTER_BOUND('',#1028,.T.);
#780=FACE_OUTER_BOUND('',#1029,.T.);
#781=FACE_OUTER_BOUND('',#1030,.T.);
#782=FACE_OUTER_BOUND('',#1031,.T.);
#783=FACE_OUTER_BOUND('',#1032,.T.);
#784=FACE_OUTER_BOUND('',#1033,.T.);
#785=FACE_OUTER_BOUND('',#1034,.T.);
#786=FACE_OUTER_BOUND('',#1035,.T.);
#787=FACE_OUTER_BOUND('',#1036,.T.);
#788=FACE_OUTER_BOUND('',#1037,.T.);
#789=FACE_OUTER_BOUND('',#1038,.T.);
#790=FACE_OUTER_BOUND('',#1039,.T.);
#791=FACE_OUTER_BOUND('',#1040,.T.);
#792=FACE_OUTER_BOUND('',#1041,.T.);
#793=FACE_OUTER_BOUND('',#1042,.T.);
#794=FACE_OUTER_BOUND('',#1043,.T.);
#795=FACE_OUTER_BOUND('',#1048,.T.);
#796=FACE_OUTER_BOUND('',#1049,.T.);
#797=FACE_OUTER_BOUND('',#1050,.T.);
#798=FACE_OUTER_BOUND('',#1051,.T.);
#799=FACE_OUTER_BOUND('',#1052,.T.);
#800=FACE_OUTER_BOUND('',#1053,.T.);
#801=FACE_OUTER_BOUND('',#1054,.T.);
#802=FACE_OUTER_BOUND('',#1055,.T.);
#803=FACE_OUTER_BOUND('',#1056,.T.);
#804=FACE_OUTER_BOUND('',#1057,.T.);
#805=FACE_OUTER_BOUND('',#1058,.T.);
#806=FACE_OUTER_BOUND('',#1059,.T.);
#807=FACE_OUTER_BOUND('',#1060,.T.);
#808=FACE_OUTER_BOUND('',#1061,.T.);
#809=FACE_OUTER_BOUND('',#1062,.T.);
#810=FACE_OUTER_BOUND('',#1063,.T.);
#811=FACE_OUTER_BOUND('',#1064,.T.);
#812=FACE_OUTER_BOUND('',#1065,.T.);
#960=EDGE_LOOP('',(#3066,#3067,#3068,#3069));
#961=EDGE_LOOP('',(#3070,#3071,#3072,#3073));
#962=EDGE_LOOP('',(#3074,#3075,#3076,#3077));
#963=EDGE_LOOP('',(#3078,#3079,#3080,#3081));
#964=EDGE_LOOP('',(#3082,#3083,#3084,#3085));
#965=EDGE_LOOP('',(#3086,#3087,#3088,#3089));
#966=EDGE_LOOP('',(#3090,#3091,#3092,#3093));
#967=EDGE_LOOP('',(#3094,#3095,#3096,#3097));
#968=EDGE_LOOP('',(#3098,#3099,#3100,#3101));
#969=EDGE_LOOP('',(#3102,#3103,#3104,#3105));
#970=EDGE_LOOP('',(#3106,#3107,#3108,#3109));
#971=EDGE_LOOP('',(#3110,#3111,#3112,#3113));
#972=EDGE_LOOP('',(#3114,#3115,#3116,#3117));
#973=EDGE_LOOP('',(#3118,#3119,#3120,#3121));
#974=EDGE_LOOP('',(#3122,#3123,#3124,#3125));
#975=EDGE_LOOP('',(#3126,#3127,#3128,#3129));
#976=EDGE_LOOP('',(#3130,#3131,#3132,#3133));
#977=EDGE_LOOP('',(#3134,#3135,#3136,#3137));
#978=EDGE_LOOP('',(#3138,#3139,#3140,#3141));
#979=EDGE_LOOP('',(#3142,#3143,#3144,#3145));
#980=EDGE_LOOP('',(#3146,#3147,#3148,#3149));
#981=EDGE_LOOP('',(#3150,#3151,#3152,#3153));
#982=EDGE_LOOP('',(#3154,#3155,#3156,#3157));
#983=EDGE_LOOP('',(#3158,#3159,#3160,#3161));
#984=EDGE_LOOP('',(#3162,#3163,#3164,#3165));
#985=EDGE_LOOP('',(#3166,#3167,#3168,#3169));
#986=EDGE_LOOP('',(#3170,#3171,#3172,#3173));
#987=EDGE_LOOP('',(#3174,#3175,#3176,#3177));
#988=EDGE_LOOP('',(#3178,#3179,#3180,#3181));
#989=EDGE_LOOP('',(#3182,#3183,#3184,#3185));
#990=EDGE_LOOP('',(#3186,#3187,#3188,#3189));
#991=EDGE_LOOP('',(#3190,#3191,#3192,#3193));
#992=EDGE_LOOP('',(#3194,#3195,#3196,#3197));
#993=EDGE_LOOP('',(#3198,#3199,#3200,#3201));
#994=EDGE_LOOP('',(#3202,#3203,#3204,#3205));
#995=EDGE_LOOP('',(#3206,#3207,#3208,#3209));
#996=EDGE_LOOP('',(#3210,#3211,#3212,#3213));
#997=EDGE_LOOP('',(#3214,#3215,#3216,#3217));
#998=EDGE_LOOP('',(#3218,#3219,#3220,#3221));
#999=EDGE_LOOP('',(#3222,#3223,#3224,#3225));
#1000=EDGE_LOOP('',(#3226,#3227,#3228,#3229));
#1001=EDGE_LOOP('',(#3230,#3231,#3232,#3233));
#1002=EDGE_LOOP('',(#3234,#3235,#3236,#3237));
#1003=EDGE_LOOP('',(#3238,#3239,#3240,#3241));
#1004=EDGE_LOOP('',(#3242,#3243,#3244,#3245));
#1005=EDGE_LOOP('',(#3246,#3247,#3248,#3249));
#1006=EDGE_LOOP('',(#3250,#3251,#3252,#3253));
#1007=EDGE_LOOP('',(#3254,#3255,#3256,#3257));
#1008=EDGE_LOOP('',(#3258,#3259,#3260,#3261));
#1009=EDGE_LOOP('',(#3262,#3263,#3264,#3265));
#1010=EDGE_LOOP('',(#3266,#3267,#3268,#3269));
#1011=EDGE_LOOP('',(#3270,#3271,#3272,#3273));
#1012=EDGE_LOOP('',(#3274,#3275,#3276,#3277));
#1013=EDGE_LOOP('',(#3278,#3279,#3280,#3281));
#1014=EDGE_LOOP('',(#3282,#3283,#3284,#3285));
#1015=EDGE_LOOP('',(#3286,#3287,#3288,#3289));
#1016=EDGE_LOOP('',(#3290,#3291,#3292,#3293));
#1017=EDGE_LOOP('',(#3294,#3295,#3296,#3297));
#1018=EDGE_LOOP('',(#3298,#3299,#3300,#3301));
#1019=EDGE_LOOP('',(#3302,#3303,#3304,#3305));
#1020=EDGE_LOOP('',(#3306,#3307,#3308,#3309));
#1021=EDGE_LOOP('',(#3310,#3311,#3312,#3313));
#1022=EDGE_LOOP('',(#3314,#3315,#3316,#3317));
#1023=EDGE_LOOP('',(#3318,#3319,#3320,#3321));
#1024=EDGE_LOOP('',(#3322,#3323,#3324,#3325));
#1025=EDGE_LOOP('',(#3326,#3327,#3328,#3329));
#1026=EDGE_LOOP('',(#3330,#3331,#3332,#3333));
#1027=EDGE_LOOP('',(#3334,#3335,#3336,#3337));
#1028=EDGE_LOOP('',(#3338,#3339,#3340,#3341));
#1029=EDGE_LOOP('',(#3342,#3343,#3344,#3345));
#1030=EDGE_LOOP('',(#3346,#3347,#3348,#3349));
#1031=EDGE_LOOP('',(#3350,#3351,#3352,#3353));
#1032=EDGE_LOOP('',(#3354,#3355,#3356,#3357));
#1033=EDGE_LOOP('',(#3358,#3359,#3360,#3361));
#1034=EDGE_LOOP('',(#3362,#3363,#3364,#3365));
#1035=EDGE_LOOP('',(#3366,#3367,#3368,#3369));
#1036=EDGE_LOOP('',(#3370,#3371,#3372,#3373));
#1037=EDGE_LOOP('',(#3374,#3375,#3376,#3377));
#1038=EDGE_LOOP('',(#3378,#3379,#3380,#3381));
#1039=EDGE_LOOP('',(#3382,#3383,#3384,#3385));
#1040=EDGE_LOOP('',(#3386,#3387,#3388,#3389));
#1041=EDGE_LOOP('',(#3390,#3391,#3392,#3393,#3394,#3395,#3396,#3397,#3398,
#3399,#3400,#3401,#3402,#3403,#3404,#3405,#3406,#3407,#3408,#3409,#3410,
#3411,#3412,#3413));
#1042=EDGE_LOOP('',(#3414,#3415,#3416,#3417,#3418,#3419,#3420,#3421,#3422,
#3423,#3424,#3425,#3426,#3427,#3428,#3429,#3430,#3431,#3432,#3433,#3434,
#3435,#3436,#3437));
#1043=EDGE_LOOP('',(#3438,#3439,#3440,#3441));
#1044=EDGE_LOOP('',(#3442,#3443,#3444,#3445));
#1045=EDGE_LOOP('',(#3446,#3447,#3448,#3449));
#1046=EDGE_LOOP('',(#3450,#3451,#3452,#3453));
#1047=EDGE_LOOP('',(#3454,#3455,#3456,#3457));
#1048=EDGE_LOOP('',(#3458,#3459,#3460,#3461));
#1049=EDGE_LOOP('',(#3462,#3463,#3464,#3465,#3466,#3467,#3468,#3469,#3470,
#3471,#3472,#3473,#3474,#3475,#3476,#3477,#3478,#3479,#3480,#3481,#3482,
#3483,#3484,#3485));
#1050=EDGE_LOOP('',(#3486,#3487,#3488,#3489,#3490,#3491,#3492,#3493,#3494,
#3495,#3496,#3497,#3498,#3499,#3500,#3501,#3502,#3503,#3504,#3505,#3506,
#3507,#3508,#3509));
#1051=EDGE_LOOP('',(#3510,#3511,#3512,#3513));
#1052=EDGE_LOOP('',(#3514,#3515,#3516,#3517,#3518,#3519,#3520,#3521,#3522,
#3523,#3524,#3525,#3526,#3527,#3528,#3529,#3530,#3531,#3532,#3533,#3534,
#3535,#3536,#3537));
#1053=EDGE_LOOP('',(#3538,#3539,#3540,#3541,#3542,#3543,#3544,#3545,#3546,
#3547,#3548,#3549,#3550,#3551,#3552,#3553,#3554,#3555,#3556,#3557,#3558,
#3559,#3560,#3561));
#1054=EDGE_LOOP('',(#3562,#3563,#3564,#3565));
#1055=EDGE_LOOP('',(#3566,#3567,#3568,#3569,#3570,#3571,#3572,#3573,#3574,
#3575,#3576,#3577,#3578,#3579,#3580,#3581,#3582,#3583,#3584,#3585,#3586,
#3587,#3588,#3589));
#1056=EDGE_LOOP('',(#3590,#3591,#3592,#3593,#3594,#3595,#3596,#3597,#3598,
#3599,#3600,#3601,#3602,#3603,#3604,#3605,#3606,#3607,#3608,#3609,#3610,
#3611,#3612,#3613));
#1057=EDGE_LOOP('',(#3614,#3615,#3616,#3617));
#1058=EDGE_LOOP('',(#3618,#3619,#3620,#3621));
#1059=EDGE_LOOP('',(#3622,#3623,#3624,#3625));
#1060=EDGE_LOOP('',(#3626,#3627,#3628,#3629));
#1061=EDGE_LOOP('',(#3630,#3631,#3632,#3633));
#1062=EDGE_LOOP('',(#3634,#3635,#3636,#3637));
#1063=EDGE_LOOP('',(#3638,#3639,#3640,#3641));
#1064=EDGE_LOOP('',(#3642,#3643,#3644,#3645));
#1065=EDGE_LOOP('',(#3646,#3647,#3648,#3649));
#1066=EDGE_LOOP('',(#3650,#3651,#3652,#3653));
#1067=EDGE_LOOP('',(#3654,#3655,#3656,#3657));
#1068=EDGE_LOOP('',(#3658,#3659,#3660,#3661));
#1069=EDGE_LOOP('',(#3662,#3663,#3664,#3665));
#1260=LINE('',#6189,#1522);
#1261=LINE('',#6210,#1523);
#1262=LINE('',#6261,#1524);
#1263=LINE('',#6312,#1525);
#1264=LINE('',#6360,#1526);
#1265=LINE('',#6408,#1527);
#1266=LINE('',#6459,#1528);
#1267=LINE('',#6510,#1529);
#1268=LINE('',#6558,#1530);
#1269=LINE('',#6609,#1531);
#1270=LINE('',#6648,#1532);
#1271=LINE('',#6669,#1533);
#1272=LINE('',#6720,#1534);
#1273=LINE('',#6771,#1535);
#1274=LINE('',#6819,#1536);
#1275=LINE('',#6867,#1537);
#1276=LINE('',#6918,#1538);
#1277=LINE('',#6969,#1539);
#1278=LINE('',#7017,#1540);
#1279=LINE('',#7068,#1541);
#1280=LINE('',#7107,#1542);
#1281=LINE('',#7128,#1543);
#1282=LINE('',#7179,#1544);
#1283=LINE('',#7230,#1545);
#1284=LINE('',#7278,#1546);
#1285=LINE('',#7326,#1547);
#1286=LINE('',#7377,#1548);
#1287=LINE('',#7428,#1549);
#1288=LINE('',#7476,#1550);
#1289=LINE('',#7527,#1551);
#1290=LINE('',#7566,#1552);
#1291=LINE('',#7587,#1553);
#1292=LINE('',#7638,#1554);
#1293=LINE('',#7689,#1555);
#1294=LINE('',#7737,#1556);
#1295=LINE('',#7785,#1557);
#1296=LINE('',#7836,#1558);
#1297=LINE('',#7887,#1559);
#1298=LINE('',#7935,#1560);
#1299=LINE('',#7986,#1561);
#1300=LINE('',#8025,#1562);
#1301=LINE('',#8049,#1563);
#1302=LINE('',#8073,#1564);
#1303=LINE('',#8098,#1565);
#1304=LINE('',#8122,#1566);
#1305=LINE('',#8147,#1567);
#1306=LINE('',#8171,#1568);
#1307=LINE('',#8196,#1569);
#1308=LINE('',#8221,#1570);
#1309=LINE('',#8245,#1571);
#1310=LINE('',#8262,#1572);
#1311=LINE('',#8286,#1573);
#1312=LINE('',#8310,#1574);
#1313=LINE('',#8335,#1575);
#1314=LINE('',#8359,#1576);
#1315=LINE('',#8384,#1577);
#1316=LINE('',#8408,#1578);
#1317=LINE('',#8433,#1579);
#1318=LINE('',#8458,#1580);
#1319=LINE('',#8482,#1581);
#1320=LINE('',#8499,#1582);
#1321=LINE('',#8523,#1583);
#1322=LINE('',#8547,#1584);
#1323=LINE('',#8572,#1585);
#1324=LINE('',#8596,#1586);
#1325=LINE('',#8621,#1587);
#1326=LINE('',#8645,#1588);
#1327=LINE('',#8670,#1589);
#1328=LINE('',#8695,#1590);
#1329=LINE('',#8719,#1591);
#1330=LINE('',#8736,#1592);
#1331=LINE('',#8760,#1593);
#1332=LINE('',#8784,#1594);
#1333=LINE('',#8809,#1595);
#1334=LINE('',#8833,#1596);
#1335=LINE('',#8858,#1597);
#1336=LINE('',#8882,#1598);
#1337=LINE('',#8907,#1599);
#1338=LINE('',#8932,#1600);
#1339=LINE('',#8956,#1601);
#1340=LINE('',#9968,#1602);
#1341=LINE('',#9970,#1603);
#1342=LINE('',#9972,#1604);
#1343=LINE('',#9973,#1605);
#1344=LINE('',#12966,#1606);
#1345=LINE('',#12967,#1607);
#1346=LINE('',#12968,#1608);
#1347=LINE('',#12971,#1609);
#1348=LINE('',#12972,#1610);
#1349=LINE('',#12975,#1611);
#1350=LINE('',#12976,#1612);
#1351=LINE('',#12978,#1613);
#1522=VECTOR('',#5159,3.);
#1523=VECTOR('',#5164,3.);
#1524=VECTOR('',#5167,3.);
#1525=VECTOR('',#5170,3.);
#1526=VECTOR('',#5173,3.);
#1527=VECTOR('',#5176,3.);
#1528=VECTOR('',#5179,3.);
#1529=VECTOR('',#5182,3.);
#1530=VECTOR('',#5185,3.);
#1531=VECTOR('',#5188,3.);
#1532=VECTOR('',#5193,3.);
#1533=VECTOR('',#5198,3.);
#1534=VECTOR('',#5201,3.);
#1535=VECTOR('',#5204,3.);
#1536=VECTOR('',#5207,3.);
#1537=VECTOR('',#5210,3.);
#1538=VECTOR('',#5213,3.);
#1539=VECTOR('',#5216,3.);
#1540=VECTOR('',#5219,3.);
#1541=VECTOR('',#5222,3.);
#1542=VECTOR('',#5227,3.);
#1543=VECTOR('',#5232,3.);
#1544=VECTOR('',#5235,3.);
#1545=VECTOR('',#5238,3.);
#1546=VECTOR('',#5241,3.);
#1547=VECTOR('',#5244,3.);
#1548=VECTOR('',#5247,3.);
#1549=VECTOR('',#5250,3.);
#1550=VECTOR('',#5253,3.);
#1551=VECTOR('',#5256,3.);
#1552=VECTOR('',#5261,3.);
#1553=VECTOR('',#5266,3.);
#1554=VECTOR('',#5269,3.);
#1555=VECTOR('',#5272,3.);
#1556=VECTOR('',#5275,3.);
#1557=VECTOR('',#5278,3.);
#1558=VECTOR('',#5281,3.);
#1559=VECTOR('',#5284,3.);
#1560=VECTOR('',#5287,3.);
#1561=VECTOR('',#5290,3.);
#1562=VECTOR('',#5295,3.0735);
#1563=VECTOR('',#5300,3.0735);
#1564=VECTOR('',#5303,3.0735);
#1565=VECTOR('',#5306,3.0735);
#1566=VECTOR('',#5309,3.0735);
#1567=VECTOR('',#5312,3.0735);
#1568=VECTOR('',#5315,3.0735);
#1569=VECTOR('',#5318,3.0735);
#1570=VECTOR('',#5321,3.0735);
#1571=VECTOR('',#5324,3.0735);
#1572=VECTOR('',#5329,3.07350000000001);
#1573=VECTOR('',#5334,3.07350000000001);
#1574=VECTOR('',#5337,3.07350000000001);
#1575=VECTOR('',#5340,3.07350000000001);
#1576=VECTOR('',#5343,3.07350000000001);
#1577=VECTOR('',#5346,3.07350000000001);
#1578=VECTOR('',#5349,3.07350000000001);
#1579=VECTOR('',#5352,3.07350000000001);
#1580=VECTOR('',#5355,3.07350000000001);
#1581=VECTOR('',#5358,3.07350000000001);
#1582=VECTOR('',#5363,3.07350000000001);
#1583=VECTOR('',#5368,3.0735);
#1584=VECTOR('',#5371,3.0735);
#1585=VECTOR('',#5374,3.0735);
#1586=VECTOR('',#5377,3.07350000000001);
#1587=VECTOR('',#5380,3.07350000000001);
#1588=VECTOR('',#5383,3.0735);
#1589=VECTOR('',#5386,3.0735);
#1590=VECTOR('',#5389,3.0735);
#1591=VECTOR('',#5392,3.0735);
#1592=VECTOR('',#5397,3.07350000000001);
#1593=VECTOR('',#5402,3.07350000000001);
#1594=VECTOR('',#5405,3.07350000000001);
#1595=VECTOR('',#5408,3.07350000000001);
#1596=VECTOR('',#5411,3.07350000000001);
#1597=VECTOR('',#5414,3.07350000000001);
#1598=VECTOR('',#5417,3.07350000000001);
#1599=VECTOR('',#5420,3.07350000000001);
#1600=VECTOR('',#5423,3.07350000000001);
#1601=VECTOR('',#5426,3.07350000000001);
#1602=VECTOR('',#5433,10.);
#1603=VECTOR('',#5434,10.);
#1604=VECTOR('',#5435,10.);
#1605=VECTOR('',#5436,10.);
#1606=VECTOR('',#5453,10.);
#1607=VECTOR('',#5454,10.);
#1608=VECTOR('',#5455,10.);
#1609=VECTOR('',#5458,10.);
#1610=VECTOR('',#5459,10.);
#1611=VECTOR('',#5462,10.);
#1612=VECTOR('',#5463,10.);
#1613=VECTOR('',#5466,10.);
#1704=CIRCLE('',#4488,2.5175);
#1705=CIRCLE('',#4498,2.5175);
#1706=CIRCLE('',#4500,2.5175);
#1707=CIRCLE('',#4510,2.5175);
#1708=CIRCLE('',#4512,2.5175);
#1709=CIRCLE('',#4522,2.5175);
#1710=CIRCLE('',#4524,2.5175);
#1711=CIRCLE('',#4534,2.5175);
#1712=CIRCLE('',#4536,3.07349999999999);
#1713=CIRCLE('',#4546,3.0735);
#1714=CIRCLE('',#4548,3.07350000000001);
#1715=CIRCLE('',#4558,3.07350000000001);
#1716=CIRCLE('',#4560,3.0735);
#1717=CIRCLE('',#4570,3.0735);
#1718=CIRCLE('',#4572,3.07350000000001);
#1719=CIRCLE('',#4582,3.07350000000001);
#1880=VERTEX_POINT('',#6187);
#1881=VERTEX_POINT('',#6188);
#1882=VERTEX_POINT('',#6190);
#1883=VERTEX_POINT('',#6195);
#1884=VERTEX_POINT('',#6208);
#1885=VERTEX_POINT('',#6209);
#1886=VERTEX_POINT('',#6259);
#1887=VERTEX_POINT('',#6260);
#1888=VERTEX_POINT('',#6310);
#1889=VERTEX_POINT('',#6311);
#1890=VERTEX_POINT('',#6358);
#1891=VERTEX_POINT('',#6359);
#1892=VERTEX_POINT('',#6406);
#1893=VERTEX_POINT('',#6407);
#1894=VERTEX_POINT('',#6457);
#1895=VERTEX_POINT('',#6458);
#1896=VERTEX_POINT('',#6508);
#1897=VERTEX_POINT('',#6509);
#1898=VERTEX_POINT('',#6556);
#1899=VERTEX_POINT('',#6557);
#1900=VERTEX_POINT('',#6607);
#1901=VERTEX_POINT('',#6608);
#1902=VERTEX_POINT('',#6610);
#1903=VERTEX_POINT('',#6624);
#1904=VERTEX_POINT('',#6646);
#1905=VERTEX_POINT('',#6647);
#1906=VERTEX_POINT('',#6649);
#1907=VERTEX_POINT('',#6654);
#1908=VERTEX_POINT('',#6667);
#1909=VERTEX_POINT('',#6668);
#1910=VERTEX_POINT('',#6718);
#1911=VERTEX_POINT('',#6719);
#1912=VERTEX_POINT('',#6769);
#1913=VERTEX_POINT('',#6770);
#1914=VERTEX_POINT('',#6817);
#1915=VERTEX_POINT('',#6818);
#1916=VERTEX_POINT('',#6865);
#1917=VERTEX_POINT('',#6866);
#1918=VERTEX_POINT('',#6916);
#1919=VERTEX_POINT('',#6917);
#1920=VERTEX_POINT('',#6967);
#1921=VERTEX_POINT('',#6968);
#1922=VERTEX_POINT('',#7015);
#1923=VERTEX_POINT('',#7016);
#1924=VERTEX_POINT('',#7066);
#1925=VERTEX_POINT('',#7067);
#1926=VERTEX_POINT('',#7069);
#1927=VERTEX_POINT('',#7083);
#1928=VERTEX_POINT('',#7105);
#1929=VERTEX_POINT('',#7106);
#1930=VERTEX_POINT('',#7108);
#1931=VERTEX_POINT('',#7113);
#1932=VERTEX_POINT('',#7126);
#1933=VERTEX_POINT('',#7127);
#1934=VERTEX_POINT('',#7177);
#1935=VERTEX_POINT('',#7178);
#1936=VERTEX_POINT('',#7228);
#1937=VERTEX_POINT('',#7229);
#1938=VERTEX_POINT('',#7276);
#1939=VERTEX_POINT('',#7277);
#1940=VERTEX_POINT('',#7324);
#1941=VERTEX_POINT('',#7325);
#1942=VERTEX_POINT('',#7375);
#1943=VERTEX_POINT('',#7376);
#1944=VERTEX_POINT('',#7426);
#1945=VERTEX_POINT('',#7427);
#1946=VERTEX_POINT('',#7474);
#1947=VERTEX_POINT('',#7475);
#1948=VERTEX_POINT('',#7525);
#1949=VERTEX_POINT('',#7526);
#1950=VERTEX_POINT('',#7528);
#1951=VERTEX_POINT('',#7542);
#1952=VERTEX_POINT('',#7564);
#1953=VERTEX_POINT('',#7565);
#1954=VERTEX_POINT('',#7567);
#1955=VERTEX_POINT('',#7572);
#1956=VERTEX_POINT('',#7585);
#1957=VERTEX_POINT('',#7586);
#1958=VERTEX_POINT('',#7636);
#1959=VERTEX_POINT('',#7637);
#1960=VERTEX_POINT('',#7687);
#1961=VERTEX_POINT('',#7688);
#1962=VERTEX_POINT('',#7735);
#1963=VERTEX_POINT('',#7736);
#1964=VERTEX_POINT('',#7783);
#1965=VERTEX_POINT('',#7784);
#1966=VERTEX_POINT('',#7834);
#1967=VERTEX_POINT('',#7835);
#1968=VERTEX_POINT('',#7885);
#1969=VERTEX_POINT('',#7886);
#1970=VERTEX_POINT('',#7933);
#1971=VERTEX_POINT('',#7934);
#1972=VERTEX_POINT('',#7984);
#1973=VERTEX_POINT('',#7985);
#1974=VERTEX_POINT('',#7987);
#1975=VERTEX_POINT('',#8001);
#1976=VERTEX_POINT('',#8023);
#1977=VERTEX_POINT('',#8024);
#1978=VERTEX_POINT('',#8026);
#1979=VERTEX_POINT('',#8035);
#1980=VERTEX_POINT('',#8047);
#1981=VERTEX_POINT('',#8048);
#1982=VERTEX_POINT('',#8071);
#1983=VERTEX_POINT('',#8072);
#1984=VERTEX_POINT('',#8096);
#1985=VERTEX_POINT('',#8097);
#1986=VERTEX_POINT('',#8120);
#1987=VERTEX_POINT('',#8121);
#1988=VERTEX_POINT('',#8145);
#1989=VERTEX_POINT('',#8146);
#1990=VERTEX_POINT('',#8169);
#1991=VERTEX_POINT('',#8170);
#1992=VERTEX_POINT('',#8194);
#1993=VERTEX_POINT('',#8195);
#1994=VERTEX_POINT('',#8219);
#1995=VERTEX_POINT('',#8220);
#1996=VERTEX_POINT('',#8243);
#1997=VERTEX_POINT('',#8244);
#1998=VERTEX_POINT('',#8246);
#1999=VERTEX_POINT('',#8252);
#2000=VERTEX_POINT('',#8260);
#2001=VERTEX_POINT('',#8261);
#2002=VERTEX_POINT('',#8263);
#2003=VERTEX_POINT('',#8272);
#2004=VERTEX_POINT('',#8284);
#2005=VERTEX_POINT('',#8285);
#2006=VERTEX_POINT('',#8308);
#2007=VERTEX_POINT('',#8309);
#2008=VERTEX_POINT('',#8333);
#2009=VERTEX_POINT('',#8334);
#2010=VERTEX_POINT('',#8357);
#2011=VERTEX_POINT('',#8358);
#2012=VERTEX_POINT('',#8382);
#2013=VERTEX_POINT('',#8383);
#2014=VERTEX_POINT('',#8406);
#2015=VERTEX_POINT('',#8407);
#2016=VERTEX_POINT('',#8431);
#2017=VERTEX_POINT('',#8432);
#2018=VERTEX_POINT('',#8456);
#2019=VERTEX_POINT('',#8457);
#2020=VERTEX_POINT('',#8480);
#2021=VERTEX_POINT('',#8481);
#2022=VERTEX_POINT('',#8483);
#2023=VERTEX_POINT('',#8489);
#2024=VERTEX_POINT('',#8497);
#2025=VERTEX_POINT('',#8498);
#2026=VERTEX_POINT('',#8500);
#2027=VERTEX_POINT('',#8509);
#2028=VERTEX_POINT('',#8521);
#2029=VERTEX_POINT('',#8522);
#2030=VERTEX_POINT('',#8545);
#2031=VERTEX_POINT('',#8546);
#2032=VERTEX_POINT('',#8570);
#2033=VERTEX_POINT('',#8571);
#2034=VERTEX_POINT('',#8594);
#2035=VERTEX_POINT('',#8595);
#2036=VERTEX_POINT('',#8619);
#2037=VERTEX_POINT('',#8620);
#2038=VERTEX_POINT('',#8643);
#2039=VERTEX_POINT('',#8644);
#2040=VERTEX_POINT('',#8668);
#2041=VERTEX_POINT('',#8669);
#2042=VERTEX_POINT('',#8693);
#2043=VERTEX_POINT('',#8694);
#2044=VERTEX_POINT('',#8717);
#2045=VERTEX_POINT('',#8718);
#2046=VERTEX_POINT('',#8720);
#2047=VERTEX_POINT('',#8726);
#2048=VERTEX_POINT('',#8734);
#2049=VERTEX_POINT('',#8735);
#2050=VERTEX_POINT('',#8737);
#2051=VERTEX_POINT('',#8746);
#2052=VERTEX_POINT('',#8758);
#2053=VERTEX_POINT('',#8759);
#2054=VERTEX_POINT('',#8782);
#2055=VERTEX_POINT('',#8783);
#2056=VERTEX_POINT('',#8807);
#2057=VERTEX_POINT('',#8808);
#2058=VERTEX_POINT('',#8831);
#2059=VERTEX_POINT('',#8832);
#2060=VERTEX_POINT('',#8856);
#2061=VERTEX_POINT('',#8857);
#2062=VERTEX_POINT('',#8880);
#2063=VERTEX_POINT('',#8881);
#2064=VERTEX_POINT('',#8905);
#2065=VERTEX_POINT('',#8906);
#2066=VERTEX_POINT('',#8930);
#2067=VERTEX_POINT('',#8931);
#2068=VERTEX_POINT('',#8954);
#2069=VERTEX_POINT('',#8955);
#2070=VERTEX_POINT('',#8957);
#2071=VERTEX_POINT('',#8963);
#2072=VERTEX_POINT('',#9966);
#2073=VERTEX_POINT('',#9967);
#2074=VERTEX_POINT('',#9969);
#2075=VERTEX_POINT('',#9971);
#2076=VERTEX_POINT('',#12964);
#2077=VERTEX_POINT('',#12965);
#2078=VERTEX_POINT('',#12970);
#2079=VERTEX_POINT('',#12974);
#2316=EDGE_CURVE('',#1880,#1881,#1260,.T.);
#2317=EDGE_CURVE('',#1881,#1882,#247,.T.);
#2318=EDGE_CURVE('',#1883,#1882,#1704,.F.);
#2319=EDGE_CURVE('',#1883,#1880,#248,.T.);
#2320=EDGE_CURVE('',#1884,#1885,#1261,.T.);
#2321=EDGE_CURVE('',#1885,#1881,#249,.T.);
#2322=EDGE_CURVE('',#1880,#1884,#250,.T.);
#2323=EDGE_CURVE('',#1886,#1887,#1262,.T.);
#2324=EDGE_CURVE('',#1887,#1885,#251,.T.);
#2325=EDGE_CURVE('',#1884,#1886,#252,.T.);
#2326=EDGE_CURVE('',#1888,#1889,#1263,.T.);
#2327=EDGE_CURVE('',#1889,#1887,#253,.T.);
#2328=EDGE_CURVE('',#1886,#1888,#254,.T.);
#2329=EDGE_CURVE('',#1890,#1891,#1264,.T.);
#2330=EDGE_CURVE('',#1891,#1889,#255,.T.);
#2331=EDGE_CURVE('',#1888,#1890,#256,.T.);
#2332=EDGE_CURVE('',#1892,#1893,#1265,.T.);
#2333=EDGE_CURVE('',#1893,#1891,#257,.T.);
#2334=EDGE_CURVE('',#1890,#1892,#258,.T.);
#2335=EDGE_CURVE('',#1894,#1895,#1266,.T.);
#2336=EDGE_CURVE('',#1895,#1893,#259,.T.);
#2337=EDGE_CURVE('',#1892,#1894,#260,.T.);
#2338=EDGE_CURVE('',#1896,#1897,#1267,.T.);
#2339=EDGE_CURVE('',#1897,#1895,#261,.T.);
#2340=EDGE_CURVE('',#1894,#1896,#262,.T.);
#2341=EDGE_CURVE('',#1898,#1899,#1268,.T.);
#2342=EDGE_CURVE('',#1899,#1897,#263,.T.);
#2343=EDGE_CURVE('',#1896,#1898,#264,.T.);
#2344=EDGE_CURVE('',#1900,#1901,#1269,.T.);
#2345=EDGE_CURVE('',#1900,#1902,#265,.T.);
#2346=EDGE_CURVE('',#1903,#1902,#1705,.T.);
#2347=EDGE_CURVE('',#1903,#1901,#266,.T.);
#2348=EDGE_CURVE('',#1904,#1905,#1270,.T.);
#2349=EDGE_CURVE('',#1905,#1906,#267,.T.);
#2350=EDGE_CURVE('',#1907,#1906,#1706,.F.);
#2351=EDGE_CURVE('',#1907,#1904,#268,.T.);
#2352=EDGE_CURVE('',#1908,#1909,#1271,.T.);
#2353=EDGE_CURVE('',#1909,#1905,#269,.T.);
#2354=EDGE_CURVE('',#1904,#1908,#270,.T.);
#2355=EDGE_CURVE('',#1910,#1911,#1272,.T.);
#2356=EDGE_CURVE('',#1911,#1909,#271,.T.);
#2357=EDGE_CURVE('',#1908,#1910,#272,.T.);
#2358=EDGE_CURVE('',#1912,#1913,#1273,.T.);
#2359=EDGE_CURVE('',#1913,#1911,#273,.T.);
#2360=EDGE_CURVE('',#1910,#1912,#274,.T.);
#2361=EDGE_CURVE('',#1914,#1915,#1274,.T.);
#2362=EDGE_CURVE('',#1915,#1913,#275,.T.);
#2363=EDGE_CURVE('',#1912,#1914,#276,.T.);
#2364=EDGE_CURVE('',#1916,#1917,#1275,.T.);
#2365=EDGE_CURVE('',#1917,#1915,#277,.T.);
#2366=EDGE_CURVE('',#1914,#1916,#278,.T.);
#2367=EDGE_CURVE('',#1918,#1919,#1276,.T.);
#2368=EDGE_CURVE('',#1919,#1917,#279,.T.);
#2369=EDGE_CURVE('',#1916,#1918,#280,.T.);
#2370=EDGE_CURVE('',#1920,#1921,#1277,.T.);
#2371=EDGE_CURVE('',#1921,#1919,#281,.T.);
#2372=EDGE_CURVE('',#1918,#1920,#282,.T.);
#2373=EDGE_CURVE('',#1922,#1923,#1278,.T.);
#2374=EDGE_CURVE('',#1923,#1921,#283,.T.);
#2375=EDGE_CURVE('',#1920,#1922,#284,.T.);
#2376=EDGE_CURVE('',#1924,#1925,#1279,.T.);
#2377=EDGE_CURVE('',#1924,#1926,#285,.T.);
#2378=EDGE_CURVE('',#1927,#1926,#1707,.T.);
#2379=EDGE_CURVE('',#1927,#1925,#286,.T.);
#2380=EDGE_CURVE('',#1928,#1929,#1280,.T.);
#2381=EDGE_CURVE('',#1929,#1930,#287,.T.);
#2382=EDGE_CURVE('',#1931,#1930,#1708,.F.);
#2383=EDGE_CURVE('',#1931,#1928,#288,.T.);
#2384=EDGE_CURVE('',#1932,#1933,#1281,.T.);
#2385=EDGE_CURVE('',#1933,#1929,#289,.T.);
#2386=EDGE_CURVE('',#1928,#1932,#290,.T.);
#2387=EDGE_CURVE('',#1934,#1935,#1282,.T.);
#2388=EDGE_CURVE('',#1935,#1933,#291,.T.);
#2389=EDGE_CURVE('',#1932,#1934,#292,.T.);
#2390=EDGE_CURVE('',#1936,#1937,#1283,.T.);
#2391=EDGE_CURVE('',#1937,#1935,#293,.T.);
#2392=EDGE_CURVE('',#1934,#1936,#294,.T.);
#2393=EDGE_CURVE('',#1938,#1939,#1284,.T.);
#2394=EDGE_CURVE('',#1939,#1937,#295,.T.);
#2395=EDGE_CURVE('',#1936,#1938,#296,.T.);
#2396=EDGE_CURVE('',#1940,#1941,#1285,.T.);
#2397=EDGE_CURVE('',#1941,#1939,#297,.T.);
#2398=EDGE_CURVE('',#1938,#1940,#298,.T.);
#2399=EDGE_CURVE('',#1942,#1943,#1286,.T.);
#2400=EDGE_CURVE('',#1943,#1941,#299,.T.);
#2401=EDGE_CURVE('',#1940,#1942,#300,.T.);
#2402=EDGE_CURVE('',#1944,#1945,#1287,.T.);
#2403=EDGE_CURVE('',#1945,#1943,#301,.T.);
#2404=EDGE_CURVE('',#1942,#1944,#302,.T.);
#2405=EDGE_CURVE('',#1946,#1947,#1288,.T.);
#2406=EDGE_CURVE('',#1947,#1945,#303,.T.);
#2407=EDGE_CURVE('',#1944,#1946,#304,.T.);
#2408=EDGE_CURVE('',#1948,#1949,#1289,.T.);
#2409=EDGE_CURVE('',#1948,#1950,#305,.T.);
#2410=EDGE_CURVE('',#1951,#1950,#1709,.T.);
#2411=EDGE_CURVE('',#1951,#1949,#306,.T.);
#2412=EDGE_CURVE('',#1952,#1953,#1290,.T.);
#2413=EDGE_CURVE('',#1953,#1954,#307,.T.);
#2414=EDGE_CURVE('',#1955,#1954,#1710,.F.);
#2415=EDGE_CURVE('',#1955,#1952,#308,.T.);
#2416=EDGE_CURVE('',#1956,#1957,#1291,.T.);
#2417=EDGE_CURVE('',#1957,#1953,#309,.T.);
#2418=EDGE_CURVE('',#1952,#1956,#310,.T.);
#2419=EDGE_CURVE('',#1958,#1959,#1292,.T.);
#2420=EDGE_CURVE('',#1959,#1957,#311,.T.);
#2421=EDGE_CURVE('',#1956,#1958,#312,.T.);
#2422=EDGE_CURVE('',#1960,#1961,#1293,.T.);
#2423=EDGE_CURVE('',#1961,#1959,#313,.T.);
#2424=EDGE_CURVE('',#1958,#1960,#314,.T.);
#2425=EDGE_CURVE('',#1962,#1963,#1294,.T.);
#2426=EDGE_CURVE('',#1963,#1961,#315,.T.);
#2427=EDGE_CURVE('',#1960,#1962,#316,.T.);
#2428=EDGE_CURVE('',#1964,#1965,#1295,.T.);
#2429=EDGE_CURVE('',#1965,#1963,#317,.T.);
#2430=EDGE_CURVE('',#1962,#1964,#318,.T.);
#2431=EDGE_CURVE('',#1966,#1967,#1296,.T.);
#2432=EDGE_CURVE('',#1967,#1965,#319,.T.);
#2433=EDGE_CURVE('',#1964,#1966,#320,.T.);
#2434=EDGE_CURVE('',#1968,#1969,#1297,.T.);
#2435=EDGE_CURVE('',#1969,#1967,#321,.T.);
#2436=EDGE_CURVE('',#1966,#1968,#322,.T.);
#2437=EDGE_CURVE('',#1970,#1971,#1298,.T.);
#2438=EDGE_CURVE('',#1971,#1969,#323,.T.);
#2439=EDGE_CURVE('',#1968,#1970,#324,.T.);
#2440=EDGE_CURVE('',#1972,#1973,#1299,.T.);
#2441=EDGE_CURVE('',#1972,#1974,#325,.T.);
#2442=EDGE_CURVE('',#1975,#1974,#1711,.T.);
#2443=EDGE_CURVE('',#1975,#1973,#326,.T.);
#2444=EDGE_CURVE('',#1976,#1977,#1300,.T.);
#2445=EDGE_CURVE('',#1977,#1978,#327,.T.);
#2446=EDGE_CURVE('',#1979,#1978,#1712,.T.);
#2447=EDGE_CURVE('',#1976,#1979,#328,.T.);
#2448=EDGE_CURVE('',#1980,#1981,#1301,.T.);
#2449=EDGE_CURVE('',#1981,#1977,#329,.T.);
#2450=EDGE_CURVE('',#1980,#1976,#330,.T.);
#2451=EDGE_CURVE('',#1982,#1983,#1302,.T.);
#2452=EDGE_CURVE('',#1983,#1981,#331,.T.);
#2453=EDGE_CURVE('',#1982,#1980,#332,.T.);
#2454=EDGE_CURVE('',#1984,#1985,#1303,.T.);
#2455=EDGE_CURVE('',#1985,#1983,#333,.T.);
#2456=EDGE_CURVE('',#1984,#1982,#334,.T.);
#2457=EDGE_CURVE('',#1986,#1987,#1304,.T.);
#2458=EDGE_CURVE('',#1987,#1985,#335,.T.);
#2459=EDGE_CURVE('',#1986,#1984,#336,.T.);
#2460=EDGE_CURVE('',#1988,#1989,#1305,.T.);
#2461=EDGE_CURVE('',#1989,#1987,#337,.T.);
#2462=EDGE_CURVE('',#1988,#1986,#338,.T.);
#2463=EDGE_CURVE('',#1990,#1991,#1306,.T.);
#2464=EDGE_CURVE('',#1991,#1989,#339,.T.);
#2465=EDGE_CURVE('',#1990,#1988,#340,.T.);
#2466=EDGE_CURVE('',#1992,#1993,#1307,.T.);
#2467=EDGE_CURVE('',#1993,#1991,#341,.T.);
#2468=EDGE_CURVE('',#1992,#1990,#342,.T.);
#2469=EDGE_CURVE('',#1994,#1995,#1308,.T.);
#2470=EDGE_CURVE('',#1995,#1993,#343,.T.);
#2471=EDGE_CURVE('',#1994,#1992,#344,.T.);
#2472=EDGE_CURVE('',#1996,#1997,#1309,.T.);
#2473=EDGE_CURVE('',#1998,#1996,#345,.T.);
#2474=EDGE_CURVE('',#1999,#1998,#1713,.T.);
#2475=EDGE_CURVE('',#1999,#1997,#346,.T.);
#2476=EDGE_CURVE('',#2000,#2001,#1310,.T.);
#2477=EDGE_CURVE('',#2001,#2002,#347,.T.);
#2478=EDGE_CURVE('',#2003,#2002,#1714,.T.);
#2479=EDGE_CURVE('',#2000,#2003,#348,.T.);
#2480=EDGE_CURVE('',#2004,#2005,#1311,.T.);
#2481=EDGE_CURVE('',#2005,#2001,#349,.T.);
#2482=EDGE_CURVE('',#2004,#2000,#350,.T.);
#2483=EDGE_CURVE('',#2006,#2007,#1312,.T.);
#2484=EDGE_CURVE('',#2007,#2005,#351,.T.);
#2485=EDGE_CURVE('',#2006,#2004,#352,.T.);
#2486=EDGE_CURVE('',#2008,#2009,#1313,.T.);
#2487=EDGE_CURVE('',#2009,#2007,#353,.T.);
#2488=EDGE_CURVE('',#2008,#2006,#354,.T.);
#2489=EDGE_CURVE('',#2010,#2011,#1314,.T.);
#2490=EDGE_CURVE('',#2011,#2009,#355,.T.);
#2491=EDGE_CURVE('',#2010,#2008,#356,.T.);
#2492=EDGE_CURVE('',#2012,#2013,#1315,.T.);
#2493=EDGE_CURVE('',#2013,#2011,#357,.T.);
#2494=EDGE_CURVE('',#2012,#2010,#358,.T.);
#2495=EDGE_CURVE('',#2014,#2015,#1316,.T.);
#2496=EDGE_CURVE('',#2015,#2013,#359,.T.);
#2497=EDGE_CURVE('',#2014,#2012,#360,.T.);
#2498=EDGE_CURVE('',#2016,#2017,#1317,.T.);
#2499=EDGE_CURVE('',#2017,#2015,#361,.T.);
#2500=EDGE_CURVE('',#2016,#2014,#362,.T.);
#2501=EDGE_CURVE('',#2018,#2019,#1318,.T.);
#2502=EDGE_CURVE('',#2019,#2017,#363,.T.);
#2503=EDGE_CURVE('',#2018,#2016,#364,.T.);
#2504=EDGE_CURVE('',#2020,#2021,#1319,.T.);
#2505=EDGE_CURVE('',#2022,#2020,#365,.T.);
#2506=EDGE_CURVE('',#2023,#2022,#1715,.T.);
#2507=EDGE_CURVE('',#2023,#2021,#366,.T.);
#2508=EDGE_CURVE('',#2024,#2025,#1320,.T.);
#2509=EDGE_CURVE('',#2025,#2026,#367,.T.);
#2510=EDGE_CURVE('',#2027,#2026,#1716,.T.);
#2511=EDGE_CURVE('',#2024,#2027,#368,.T.);
#2512=EDGE_CURVE('',#2028,#2029,#1321,.T.);
#2513=EDGE_CURVE('',#2029,#2025,#369,.T.);
#2514=EDGE_CURVE('',#2028,#2024,#370,.T.);
#2515=EDGE_CURVE('',#2030,#2031,#1322,.T.);
#2516=EDGE_CURVE('',#2031,#2029,#371,.T.);
#2517=EDGE_CURVE('',#2030,#2028,#372,.T.);
#2518=EDGE_CURVE('',#2032,#2033,#1323,.T.);
#2519=EDGE_CURVE('',#2033,#2031,#373,.T.);
#2520=EDGE_CURVE('',#2032,#2030,#374,.T.);
#2521=EDGE_CURVE('',#2034,#2035,#1324,.T.);
#2522=EDGE_CURVE('',#2035,#2033,#375,.T.);
#2523=EDGE_CURVE('',#2034,#2032,#376,.T.);
#2524=EDGE_CURVE('',#2036,#2037,#1325,.T.);
#2525=EDGE_CURVE('',#2037,#2035,#377,.T.);
#2526=EDGE_CURVE('',#2036,#2034,#378,.T.);
#2527=EDGE_CURVE('',#2038,#2039,#1326,.T.);
#2528=EDGE_CURVE('',#2039,#2037,#379,.T.);
#2529=EDGE_CURVE('',#2038,#2036,#380,.T.);
#2530=EDGE_CURVE('',#2040,#2041,#1327,.T.);
#2531=EDGE_CURVE('',#2041,#2039,#381,.T.);
#2532=EDGE_CURVE('',#2040,#2038,#382,.T.);
#2533=EDGE_CURVE('',#2042,#2043,#1328,.T.);
#2534=EDGE_CURVE('',#2043,#2041,#383,.T.);
#2535=EDGE_CURVE('',#2042,#2040,#384,.T.);
#2536=EDGE_CURVE('',#2044,#2045,#1329,.T.);
#2537=EDGE_CURVE('',#2046,#2044,#385,.T.);
#2538=EDGE_CURVE('',#2047,#2046,#1717,.T.);
#2539=EDGE_CURVE('',#2047,#2045,#386,.T.);
#2540=EDGE_CURVE('',#2048,#2049,#1330,.T.);
#2541=EDGE_CURVE('',#2049,#2050,#387,.T.);
#2542=EDGE_CURVE('',#2051,#2050,#1718,.T.);
#2543=EDGE_CURVE('',#2048,#2051,#388,.T.);
#2544=EDGE_CURVE('',#2052,#2053,#1331,.T.);
#2545=EDGE_CURVE('',#2053,#2049,#389,.T.);
#2546=EDGE_CURVE('',#2052,#2048,#390,.T.);
#2547=EDGE_CURVE('',#2054,#2055,#1332,.T.);
#2548=EDGE_CURVE('',#2055,#2053,#391,.T.);
#2549=EDGE_CURVE('',#2054,#2052,#392,.T.);
#2550=EDGE_CURVE('',#2056,#2057,#1333,.T.);
#2551=EDGE_CURVE('',#2057,#2055,#393,.T.);
#2552=EDGE_CURVE('',#2056,#2054,#394,.T.);
#2553=EDGE_CURVE('',#2058,#2059,#1334,.T.);
#2554=EDGE_CURVE('',#2059,#2057,#395,.T.);
#2555=EDGE_CURVE('',#2058,#2056,#396,.T.);
#2556=EDGE_CURVE('',#2060,#2061,#1335,.T.);
#2557=EDGE_CURVE('',#2061,#2059,#397,.T.);
#2558=EDGE_CURVE('',#2060,#2058,#398,.T.);
#2559=EDGE_CURVE('',#2062,#2063,#1336,.T.);
#2560=EDGE_CURVE('',#2063,#2061,#399,.T.);
#2561=EDGE_CURVE('',#2062,#2060,#400,.T.);
#2562=EDGE_CURVE('',#2064,#2065,#1337,.T.);
#2563=EDGE_CURVE('',#2065,#2063,#401,.T.);
#2564=EDGE_CURVE('',#2064,#2062,#402,.T.);
#2565=EDGE_CURVE('',#2066,#2067,#1338,.T.);
#2566=EDGE_CURVE('',#2067,#2065,#403,.T.);
#2567=EDGE_CURVE('',#2066,#2064,#404,.T.);
#2568=EDGE_CURVE('',#2068,#2069,#1339,.T.);
#2569=EDGE_CURVE('',#2070,#2068,#405,.T.);
#2570=EDGE_CURVE('',#2071,#2070,#1719,.T.);
#2571=EDGE_CURVE('',#2071,#2069,#406,.T.);
#2572=EDGE_CURVE('',#2069,#2067,#407,.T.);
#2573=EDGE_CURVE('',#2068,#2066,#408,.T.);
#2574=EDGE_CURVE('',#2050,#1931,#409,.T.);
#2575=EDGE_CURVE('',#1950,#2071,#410,.T.);
#2576=EDGE_CURVE('',#1946,#1948,#411,.T.);
#2577=EDGE_CURVE('',#1930,#2051,#412,.T.);
#2578=EDGE_CURVE('',#1949,#1947,#413,.T.);
#2579=EDGE_CURVE('',#2070,#1951,#414,.T.);
#2580=EDGE_CURVE('',#2072,#2073,#1340,.T.);
#2581=EDGE_CURVE('',#2073,#2074,#1341,.T.);
#2582=EDGE_CURVE('',#2074,#2075,#1342,.T.);
#2583=EDGE_CURVE('',#2075,#2072,#1343,.T.);
#2584=EDGE_CURVE('',#1974,#2047,#415,.T.);
#2585=EDGE_CURVE('',#2046,#1975,#416,.T.);
#2586=EDGE_CURVE('',#1926,#2023,#417,.T.);
#2587=EDGE_CURVE('',#2022,#1927,#418,.T.);
#2588=EDGE_CURVE('',#1902,#1999,#419,.T.);
#2589=EDGE_CURVE('',#1998,#1903,#420,.T.);
#2590=EDGE_CURVE('',#2045,#2043,#421,.T.);
#2591=EDGE_CURVE('',#2044,#2042,#422,.T.);
#2592=EDGE_CURVE('',#2026,#1955,#423,.T.);
#2593=EDGE_CURVE('',#1970,#1972,#424,.T.);
#2594=EDGE_CURVE('',#1954,#2027,#425,.T.);
#2595=EDGE_CURVE('',#1973,#1971,#426,.T.);
#2596=EDGE_CURVE('',#2021,#2019,#427,.T.);
#2597=EDGE_CURVE('',#2020,#2018,#428,.T.);
#2598=EDGE_CURVE('',#2002,#1907,#429,.T.);
#2599=EDGE_CURVE('',#1922,#1924,#430,.T.);
#2600=EDGE_CURVE('',#1906,#2003,#431,.T.);
#2601=EDGE_CURVE('',#1925,#1923,#432,.T.);
#2602=EDGE_CURVE('',#1997,#1995,#433,.T.);
#2603=EDGE_CURVE('',#1996,#1994,#434,.T.);
#2604=EDGE_CURVE('',#1978,#1883,#435,.T.);
#2605=EDGE_CURVE('',#1898,#1900,#436,.T.);
#2606=EDGE_CURVE('',#1882,#1979,#437,.T.);
#2607=EDGE_CURVE('',#1901,#1899,#438,.T.);
#2608=EDGE_CURVE('',#2076,#2077,#1344,.T.);
#2609=EDGE_CURVE('',#2077,#2072,#1345,.T.);
#2610=EDGE_CURVE('',#2076,#2075,#1346,.T.);
#2611=EDGE_CURVE('',#2078,#2076,#1347,.T.);
#2612=EDGE_CURVE('',#2078,#2074,#1348,.T.);
#2613=EDGE_CURVE('',#2079,#2078,#1349,.T.);
#2614=EDGE_CURVE('',#2079,#2073,#1350,.T.);
#2615=EDGE_CURVE('',#2077,#2079,#1351,.T.);
#3066=ORIENTED_EDGE('',*,*,#2316,.T.);
#3067=ORIENTED_EDGE('',*,*,#2317,.T.);
#3068=ORIENTED_EDGE('',*,*,#2318,.F.);
#3069=ORIENTED_EDGE('',*,*,#2319,.T.);
#3070=ORIENTED_EDGE('',*,*,#2320,.T.);
#3071=ORIENTED_EDGE('',*,*,#2321,.T.);
#3072=ORIENTED_EDGE('',*,*,#2316,.F.);
#3073=ORIENTED_EDGE('',*,*,#2322,.T.);
#3074=ORIENTED_EDGE('',*,*,#2323,.T.);
#3075=ORIENTED_EDGE('',*,*,#2324,.T.);
#3076=ORIENTED_EDGE('',*,*,#2320,.F.);
#3077=ORIENTED_EDGE('',*,*,#2325,.T.);
#3078=ORIENTED_EDGE('',*,*,#2326,.T.);
#3079=ORIENTED_EDGE('',*,*,#2327,.T.);
#3080=ORIENTED_EDGE('',*,*,#2323,.F.);
#3081=ORIENTED_EDGE('',*,*,#2328,.T.);
#3082=ORIENTED_EDGE('',*,*,#2329,.T.);
#3083=ORIENTED_EDGE('',*,*,#2330,.T.);
#3084=ORIENTED_EDGE('',*,*,#2326,.F.);
#3085=ORIENTED_EDGE('',*,*,#2331,.T.);
#3086=ORIENTED_EDGE('',*,*,#2332,.T.);
#3087=ORIENTED_EDGE('',*,*,#2333,.T.);
#3088=ORIENTED_EDGE('',*,*,#2329,.F.);
#3089=ORIENTED_EDGE('',*,*,#2334,.T.);
#3090=ORIENTED_EDGE('',*,*,#2335,.T.);
#3091=ORIENTED_EDGE('',*,*,#2336,.T.);
#3092=ORIENTED_EDGE('',*,*,#2332,.F.);
#3093=ORIENTED_EDGE('',*,*,#2337,.T.);
#3094=ORIENTED_EDGE('',*,*,#2338,.T.);
#3095=ORIENTED_EDGE('',*,*,#2339,.T.);
#3096=ORIENTED_EDGE('',*,*,#2335,.F.);
#3097=ORIENTED_EDGE('',*,*,#2340,.T.);
#3098=ORIENTED_EDGE('',*,*,#2341,.T.);
#3099=ORIENTED_EDGE('',*,*,#2342,.T.);
#3100=ORIENTED_EDGE('',*,*,#2338,.F.);
#3101=ORIENTED_EDGE('',*,*,#2343,.T.);
#3102=ORIENTED_EDGE('',*,*,#2344,.F.);
#3103=ORIENTED_EDGE('',*,*,#2345,.T.);
#3104=ORIENTED_EDGE('',*,*,#2346,.F.);
#3105=ORIENTED_EDGE('',*,*,#2347,.T.);
#3106=ORIENTED_EDGE('',*,*,#2348,.T.);
#3107=ORIENTED_EDGE('',*,*,#2349,.T.);
#3108=ORIENTED_EDGE('',*,*,#2350,.F.);
#3109=ORIENTED_EDGE('',*,*,#2351,.T.);
#3110=ORIENTED_EDGE('',*,*,#2352,.T.);
#3111=ORIENTED_EDGE('',*,*,#2353,.T.);
#3112=ORIENTED_EDGE('',*,*,#2348,.F.);
#3113=ORIENTED_EDGE('',*,*,#2354,.T.);
#3114=ORIENTED_EDGE('',*,*,#2355,.T.);
#3115=ORIENTED_EDGE('',*,*,#2356,.T.);
#3116=ORIENTED_EDGE('',*,*,#2352,.F.);
#3117=ORIENTED_EDGE('',*,*,#2357,.T.);
#3118=ORIENTED_EDGE('',*,*,#2358,.T.);
#3119=ORIENTED_EDGE('',*,*,#2359,.T.);
#3120=ORIENTED_EDGE('',*,*,#2355,.F.);
#3121=ORIENTED_EDGE('',*,*,#2360,.T.);
#3122=ORIENTED_EDGE('',*,*,#2361,.T.);
#3123=ORIENTED_EDGE('',*,*,#2362,.T.);
#3124=ORIENTED_EDGE('',*,*,#2358,.F.);
#3125=ORIENTED_EDGE('',*,*,#2363,.T.);
#3126=ORIENTED_EDGE('',*,*,#2364,.T.);
#3127=ORIENTED_EDGE('',*,*,#2365,.T.);
#3128=ORIENTED_EDGE('',*,*,#2361,.F.);
#3129=ORIENTED_EDGE('',*,*,#2366,.T.);
#3130=ORIENTED_EDGE('',*,*,#2367,.T.);
#3131=ORIENTED_EDGE('',*,*,#2368,.T.);
#3132=ORIENTED_EDGE('',*,*,#2364,.F.);
#3133=ORIENTED_EDGE('',*,*,#2369,.T.);
#3134=ORIENTED_EDGE('',*,*,#2370,.T.);
#3135=ORIENTED_EDGE('',*,*,#2371,.T.);
#3136=ORIENTED_EDGE('',*,*,#2367,.F.);
#3137=ORIENTED_EDGE('',*,*,#2372,.T.);
#3138=ORIENTED_EDGE('',*,*,#2373,.T.);
#3139=ORIENTED_EDGE('',*,*,#2374,.T.);
#3140=ORIENTED_EDGE('',*,*,#2370,.F.);
#3141=ORIENTED_EDGE('',*,*,#2375,.T.);
#3142=ORIENTED_EDGE('',*,*,#2376,.F.);
#3143=ORIENTED_EDGE('',*,*,#2377,.T.);
#3144=ORIENTED_EDGE('',*,*,#2378,.F.);
#3145=ORIENTED_EDGE('',*,*,#2379,.T.);
#3146=ORIENTED_EDGE('',*,*,#2380,.T.);
#3147=ORIENTED_EDGE('',*,*,#2381,.T.);
#3148=ORIENTED_EDGE('',*,*,#2382,.F.);
#3149=ORIENTED_EDGE('',*,*,#2383,.T.);
#3150=ORIENTED_EDGE('',*,*,#2384,.T.);
#3151=ORIENTED_EDGE('',*,*,#2385,.T.);
#3152=ORIENTED_EDGE('',*,*,#2380,.F.);
#3153=ORIENTED_EDGE('',*,*,#2386,.T.);
#3154=ORIENTED_EDGE('',*,*,#2387,.T.);
#3155=ORIENTED_EDGE('',*,*,#2388,.T.);
#3156=ORIENTED_EDGE('',*,*,#2384,.F.);
#3157=ORIENTED_EDGE('',*,*,#2389,.T.);
#3158=ORIENTED_EDGE('',*,*,#2390,.T.);
#3159=ORIENTED_EDGE('',*,*,#2391,.T.);
#3160=ORIENTED_EDGE('',*,*,#2387,.F.);
#3161=ORIENTED_EDGE('',*,*,#2392,.T.);
#3162=ORIENTED_EDGE('',*,*,#2393,.T.);
#3163=ORIENTED_EDGE('',*,*,#2394,.T.);
#3164=ORIENTED_EDGE('',*,*,#2390,.F.);
#3165=ORIENTED_EDGE('',*,*,#2395,.T.);
#3166=ORIENTED_EDGE('',*,*,#2396,.T.);
#3167=ORIENTED_EDGE('',*,*,#2397,.T.);
#3168=ORIENTED_EDGE('',*,*,#2393,.F.);
#3169=ORIENTED_EDGE('',*,*,#2398,.T.);
#3170=ORIENTED_EDGE('',*,*,#2399,.T.);
#3171=ORIENTED_EDGE('',*,*,#2400,.T.);
#3172=ORIENTED_EDGE('',*,*,#2396,.F.);
#3173=ORIENTED_EDGE('',*,*,#2401,.T.);
#3174=ORIENTED_EDGE('',*,*,#2402,.T.);
#3175=ORIENTED_EDGE('',*,*,#2403,.T.);
#3176=ORIENTED_EDGE('',*,*,#2399,.F.);
#3177=ORIENTED_EDGE('',*,*,#2404,.T.);
#3178=ORIENTED_EDGE('',*,*,#2405,.T.);
#3179=ORIENTED_EDGE('',*,*,#2406,.T.);
#3180=ORIENTED_EDGE('',*,*,#2402,.F.);
#3181=ORIENTED_EDGE('',*,*,#2407,.T.);
#3182=ORIENTED_EDGE('',*,*,#2408,.F.);
#3183=ORIENTED_EDGE('',*,*,#2409,.T.);
#3184=ORIENTED_EDGE('',*,*,#2410,.F.);
#3185=ORIENTED_EDGE('',*,*,#2411,.T.);
#3186=ORIENTED_EDGE('',*,*,#2412,.T.);
#3187=ORIENTED_EDGE('',*,*,#2413,.T.);
#3188=ORIENTED_EDGE('',*,*,#2414,.F.);
#3189=ORIENTED_EDGE('',*,*,#2415,.T.);
#3190=ORIENTED_EDGE('',*,*,#2416,.T.);
#3191=ORIENTED_EDGE('',*,*,#2417,.T.);
#3192=ORIENTED_EDGE('',*,*,#2412,.F.);
#3193=ORIENTED_EDGE('',*,*,#2418,.T.);
#3194=ORIENTED_EDGE('',*,*,#2419,.T.);
#3195=ORIENTED_EDGE('',*,*,#2420,.T.);
#3196=ORIENTED_EDGE('',*,*,#2416,.F.);
#3197=ORIENTED_EDGE('',*,*,#2421,.T.);
#3198=ORIENTED_EDGE('',*,*,#2422,.T.);
#3199=ORIENTED_EDGE('',*,*,#2423,.T.);
#3200=ORIENTED_EDGE('',*,*,#2419,.F.);
#3201=ORIENTED_EDGE('',*,*,#2424,.T.);
#3202=ORIENTED_EDGE('',*,*,#2425,.T.);
#3203=ORIENTED_EDGE('',*,*,#2426,.T.);
#3204=ORIENTED_EDGE('',*,*,#2422,.F.);
#3205=ORIENTED_EDGE('',*,*,#2427,.T.);
#3206=ORIENTED_EDGE('',*,*,#2428,.T.);
#3207=ORIENTED_EDGE('',*,*,#2429,.T.);
#3208=ORIENTED_EDGE('',*,*,#2425,.F.);
#3209=ORIENTED_EDGE('',*,*,#2430,.T.);
#3210=ORIENTED_EDGE('',*,*,#2431,.T.);
#3211=ORIENTED_EDGE('',*,*,#2432,.T.);
#3212=ORIENTED_EDGE('',*,*,#2428,.F.);
#3213=ORIENTED_EDGE('',*,*,#2433,.T.);
#3214=ORIENTED_EDGE('',*,*,#2434,.T.);
#3215=ORIENTED_EDGE('',*,*,#2435,.T.);
#3216=ORIENTED_EDGE('',*,*,#2431,.F.);
#3217=ORIENTED_EDGE('',*,*,#2436,.T.);
#3218=ORIENTED_EDGE('',*,*,#2437,.T.);
#3219=ORIENTED_EDGE('',*,*,#2438,.T.);
#3220=ORIENTED_EDGE('',*,*,#2434,.F.);
#3221=ORIENTED_EDGE('',*,*,#2439,.T.);
#3222=ORIENTED_EDGE('',*,*,#2440,.F.);
#3223=ORIENTED_EDGE('',*,*,#2441,.T.);
#3224=ORIENTED_EDGE('',*,*,#2442,.F.);
#3225=ORIENTED_EDGE('',*,*,#2443,.T.);
#3226=ORIENTED_EDGE('',*,*,#2444,.T.);
#3227=ORIENTED_EDGE('',*,*,#2445,.T.);
#3228=ORIENTED_EDGE('',*,*,#2446,.F.);
#3229=ORIENTED_EDGE('',*,*,#2447,.F.);
#3230=ORIENTED_EDGE('',*,*,#2448,.T.);
#3231=ORIENTED_EDGE('',*,*,#2449,.T.);
#3232=ORIENTED_EDGE('',*,*,#2444,.F.);
#3233=ORIENTED_EDGE('',*,*,#2450,.F.);
#3234=ORIENTED_EDGE('',*,*,#2451,.T.);
#3235=ORIENTED_EDGE('',*,*,#2452,.T.);
#3236=ORIENTED_EDGE('',*,*,#2448,.F.);
#3237=ORIENTED_EDGE('',*,*,#2453,.F.);
#3238=ORIENTED_EDGE('',*,*,#2454,.T.);
#3239=ORIENTED_EDGE('',*,*,#2455,.T.);
#3240=ORIENTED_EDGE('',*,*,#2451,.F.);
#3241=ORIENTED_EDGE('',*,*,#2456,.F.);
#3242=ORIENTED_EDGE('',*,*,#2457,.T.);
#3243=ORIENTED_EDGE('',*,*,#2458,.T.);
#3244=ORIENTED_EDGE('',*,*,#2454,.F.);
#3245=ORIENTED_EDGE('',*,*,#2459,.F.);
#3246=ORIENTED_EDGE('',*,*,#2460,.T.);
#3247=ORIENTED_EDGE('',*,*,#2461,.T.);
#3248=ORIENTED_EDGE('',*,*,#2457,.F.);
#3249=ORIENTED_EDGE('',*,*,#2462,.F.);
#3250=ORIENTED_EDGE('',*,*,#2463,.T.);
#3251=ORIENTED_EDGE('',*,*,#2464,.T.);
#3252=ORIENTED_EDGE('',*,*,#2460,.F.);
#3253=ORIENTED_EDGE('',*,*,#2465,.F.);
#3254=ORIENTED_EDGE('',*,*,#2466,.T.);
#3255=ORIENTED_EDGE('',*,*,#2467,.T.);
#3256=ORIENTED_EDGE('',*,*,#2463,.F.);
#3257=ORIENTED_EDGE('',*,*,#2468,.F.);
#3258=ORIENTED_EDGE('',*,*,#2469,.T.);
#3259=ORIENTED_EDGE('',*,*,#2470,.T.);
#3260=ORIENTED_EDGE('',*,*,#2466,.F.);
#3261=ORIENTED_EDGE('',*,*,#2471,.F.);
#3262=ORIENTED_EDGE('',*,*,#2472,.F.);
#3263=ORIENTED_EDGE('',*,*,#2473,.F.);
#3264=ORIENTED_EDGE('',*,*,#2474,.F.);
#3265=ORIENTED_EDGE('',*,*,#2475,.T.);
#3266=ORIENTED_EDGE('',*,*,#2476,.T.);
#3267=ORIENTED_EDGE('',*,*,#2477,.T.);
#3268=ORIENTED_EDGE('',*,*,#2478,.F.);
#3269=ORIENTED_EDGE('',*,*,#2479,.F.);
#3270=ORIENTED_EDGE('',*,*,#2480,.T.);
#3271=ORIENTED_EDGE('',*,*,#2481,.T.);
#3272=ORIENTED_EDGE('',*,*,#2476,.F.);
#3273=ORIENTED_EDGE('',*,*,#2482,.F.);
#3274=ORIENTED_EDGE('',*,*,#2483,.T.);
#3275=ORIENTED_EDGE('',*,*,#2484,.T.);
#3276=ORIENTED_EDGE('',*,*,#2480,.F.);
#3277=ORIENTED_EDGE('',*,*,#2485,.F.);
#3278=ORIENTED_EDGE('',*,*,#2486,.T.);
#3279=ORIENTED_EDGE('',*,*,#2487,.T.);
#3280=ORIENTED_EDGE('',*,*,#2483,.F.);
#3281=ORIENTED_EDGE('',*,*,#2488,.F.);
#3282=ORIENTED_EDGE('',*,*,#2489,.T.);
#3283=ORIENTED_EDGE('',*,*,#2490,.T.);
#3284=ORIENTED_EDGE('',*,*,#2486,.F.);
#3285=ORIENTED_EDGE('',*,*,#2491,.F.);
#3286=ORIENTED_EDGE('',*,*,#2492,.T.);
#3287=ORIENTED_EDGE('',*,*,#2493,.T.);
#3288=ORIENTED_EDGE('',*,*,#2489,.F.);
#3289=ORIENTED_EDGE('',*,*,#2494,.F.);
#3290=ORIENTED_EDGE('',*,*,#2495,.T.);
#3291=ORIENTED_EDGE('',*,*,#2496,.T.);
#3292=ORIENTED_EDGE('',*,*,#2492,.F.);
#3293=ORIENTED_EDGE('',*,*,#2497,.F.);
#3294=ORIENTED_EDGE('',*,*,#2498,.T.);
#3295=ORIENTED_EDGE('',*,*,#2499,.T.);
#3296=ORIENTED_EDGE('',*,*,#2495,.F.);
#3297=ORIENTED_EDGE('',*,*,#2500,.F.);
#3298=ORIENTED_EDGE('',*,*,#2501,.T.);
#3299=ORIENTED_EDGE('',*,*,#2502,.T.);
#3300=ORIENTED_EDGE('',*,*,#2498,.F.);
#3301=ORIENTED_EDGE('',*,*,#2503,.F.);
#3302=ORIENTED_EDGE('',*,*,#2504,.F.);
#3303=ORIENTED_EDGE('',*,*,#2505,.F.);
#3304=ORIENTED_EDGE('',*,*,#2506,.F.);
#3305=ORIENTED_EDGE('',*,*,#2507,.T.);
#3306=ORIENTED_EDGE('',*,*,#2508,.T.);
#3307=ORIENTED_EDGE('',*,*,#2509,.T.);
#3308=ORIENTED_EDGE('',*,*,#2510,.F.);
#3309=ORIENTED_EDGE('',*,*,#2511,.F.);
#3310=ORIENTED_EDGE('',*,*,#2512,.T.);
#3311=ORIENTED_EDGE('',*,*,#2513,.T.);
#3312=ORIENTED_EDGE('',*,*,#2508,.F.);
#3313=ORIENTED_EDGE('',*,*,#2514,.F.);
#3314=ORIENTED_EDGE('',*,*,#2515,.T.);
#3315=ORIENTED_EDGE('',*,*,#2516,.T.);
#3316=ORIENTED_EDGE('',*,*,#2512,.F.);
#3317=ORIENTED_EDGE('',*,*,#2517,.F.);
#3318=ORIENTED_EDGE('',*,*,#2518,.T.);
#3319=ORIENTED_EDGE('',*,*,#2519,.T.);
#3320=ORIENTED_EDGE('',*,*,#2515,.F.);
#3321=ORIENTED_EDGE('',*,*,#2520,.F.);
#3322=ORIENTED_EDGE('',*,*,#2521,.T.);
#3323=ORIENTED_EDGE('',*,*,#2522,.T.);
#3324=ORIENTED_EDGE('',*,*,#2518,.F.);
#3325=ORIENTED_EDGE('',*,*,#2523,.F.);
#3326=ORIENTED_EDGE('',*,*,#2524,.T.);
#3327=ORIENTED_EDGE('',*,*,#2525,.T.);
#3328=ORIENTED_EDGE('',*,*,#2521,.F.);
#3329=ORIENTED_EDGE('',*,*,#2526,.F.);
#3330=ORIENTED_EDGE('',*,*,#2527,.T.);
#3331=ORIENTED_EDGE('',*,*,#2528,.T.);
#3332=ORIENTED_EDGE('',*,*,#2524,.F.);
#3333=ORIENTED_EDGE('',*,*,#2529,.F.);
#3334=ORIENTED_EDGE('',*,*,#2530,.T.);
#3335=ORIENTED_EDGE('',*,*,#2531,.T.);
#3336=ORIENTED_EDGE('',*,*,#2527,.F.);
#3337=ORIENTED_EDGE('',*,*,#2532,.F.);
#3338=ORIENTED_EDGE('',*,*,#2533,.T.);
#3339=ORIENTED_EDGE('',*,*,#2534,.T.);
#3340=ORIENTED_EDGE('',*,*,#2530,.F.);
#3341=ORIENTED_EDGE('',*,*,#2535,.F.);
#3342=ORIENTED_EDGE('',*,*,#2536,.F.);
#3343=ORIENTED_EDGE('',*,*,#2537,.F.);
#3344=ORIENTED_EDGE('',*,*,#2538,.F.);
#3345=ORIENTED_EDGE('',*,*,#2539,.T.);
#3346=ORIENTED_EDGE('',*,*,#2540,.T.);
#3347=ORIENTED_EDGE('',*,*,#2541,.T.);
#3348=ORIENTED_EDGE('',*,*,#2542,.F.);
#3349=ORIENTED_EDGE('',*,*,#2543,.F.);
#3350=ORIENTED_EDGE('',*,*,#2544,.T.);
#3351=ORIENTED_EDGE('',*,*,#2545,.T.);
#3352=ORIENTED_EDGE('',*,*,#2540,.F.);
#3353=ORIENTED_EDGE('',*,*,#2546,.F.);
#3354=ORIENTED_EDGE('',*,*,#2547,.T.);
#3355=ORIENTED_EDGE('',*,*,#2548,.T.);
#3356=ORIENTED_EDGE('',*,*,#2544,.F.);
#3357=ORIENTED_EDGE('',*,*,#2549,.F.);
#3358=ORIENTED_EDGE('',*,*,#2550,.T.);
#3359=ORIENTED_EDGE('',*,*,#2551,.T.);
#3360=ORIENTED_EDGE('',*,*,#2547,.F.);
#3361=ORIENTED_EDGE('',*,*,#2552,.F.);
#3362=ORIENTED_EDGE('',*,*,#2553,.T.);
#3363=ORIENTED_EDGE('',*,*,#2554,.T.);
#3364=ORIENTED_EDGE('',*,*,#2550,.F.);
#3365=ORIENTED_EDGE('',*,*,#2555,.F.);
#3366=ORIENTED_EDGE('',*,*,#2556,.T.);
#3367=ORIENTED_EDGE('',*,*,#2557,.T.);
#3368=ORIENTED_EDGE('',*,*,#2553,.F.);
#3369=ORIENTED_EDGE('',*,*,#2558,.F.);
#3370=ORIENTED_EDGE('',*,*,#2559,.T.);
#3371=ORIENTED_EDGE('',*,*,#2560,.T.);
#3372=ORIENTED_EDGE('',*,*,#2556,.F.);
#3373=ORIENTED_EDGE('',*,*,#2561,.F.);
#3374=ORIENTED_EDGE('',*,*,#2562,.T.);
#3375=ORIENTED_EDGE('',*,*,#2563,.T.);
#3376=ORIENTED_EDGE('',*,*,#2559,.F.);
#3377=ORIENTED_EDGE('',*,*,#2564,.F.);
#3378=ORIENTED_EDGE('',*,*,#2565,.T.);
#3379=ORIENTED_EDGE('',*,*,#2566,.T.);
#3380=ORIENTED_EDGE('',*,*,#2562,.F.);
#3381=ORIENTED_EDGE('',*,*,#2567,.F.);
#3382=ORIENTED_EDGE('',*,*,#2568,.F.);
#3383=ORIENTED_EDGE('',*,*,#2569,.F.);
#3384=ORIENTED_EDGE('',*,*,#2570,.F.);
#3385=ORIENTED_EDGE('',*,*,#2571,.T.);
#3386=ORIENTED_EDGE('',*,*,#2568,.T.);
#3387=ORIENTED_EDGE('',*,*,#2572,.T.);
#3388=ORIENTED_EDGE('',*,*,#2565,.F.);
#3389=ORIENTED_EDGE('',*,*,#2573,.F.);
#3390=ORIENTED_EDGE('',*,*,#2574,.F.);
#3391=ORIENTED_EDGE('',*,*,#2541,.F.);
#3392=ORIENTED_EDGE('',*,*,#2545,.F.);
#3393=ORIENTED_EDGE('',*,*,#2548,.F.);
#3394=ORIENTED_EDGE('',*,*,#2551,.F.);
#3395=ORIENTED_EDGE('',*,*,#2554,.F.);
#3396=ORIENTED_EDGE('',*,*,#2557,.F.);
#3397=ORIENTED_EDGE('',*,*,#2560,.F.);
#3398=ORIENTED_EDGE('',*,*,#2563,.F.);
#3399=ORIENTED_EDGE('',*,*,#2566,.F.);
#3400=ORIENTED_EDGE('',*,*,#2572,.F.);
#3401=ORIENTED_EDGE('',*,*,#2571,.F.);
#3402=ORIENTED_EDGE('',*,*,#2575,.F.);
#3403=ORIENTED_EDGE('',*,*,#2409,.F.);
#3404=ORIENTED_EDGE('',*,*,#2576,.F.);
#3405=ORIENTED_EDGE('',*,*,#2407,.F.);
#3406=ORIENTED_EDGE('',*,*,#2404,.F.);
#3407=ORIENTED_EDGE('',*,*,#2401,.F.);
#3408=ORIENTED_EDGE('',*,*,#2398,.F.);
#3409=ORIENTED_EDGE('',*,*,#2395,.F.);
#3410=ORIENTED_EDGE('',*,*,#2392,.F.);
#3411=ORIENTED_EDGE('',*,*,#2389,.F.);
#3412=ORIENTED_EDGE('',*,*,#2386,.F.);
#3413=ORIENTED_EDGE('',*,*,#2383,.F.);
#3414=ORIENTED_EDGE('',*,*,#2577,.F.);
#3415=ORIENTED_EDGE('',*,*,#2381,.F.);
#3416=ORIENTED_EDGE('',*,*,#2385,.F.);
#3417=ORIENTED_EDGE('',*,*,#2388,.F.);
#3418=ORIENTED_EDGE('',*,*,#2391,.F.);
#3419=ORIENTED_EDGE('',*,*,#2394,.F.);
#3420=ORIENTED_EDGE('',*,*,#2397,.F.);
#3421=ORIENTED_EDGE('',*,*,#2400,.F.);
#3422=ORIENTED_EDGE('',*,*,#2403,.F.);
#3423=ORIENTED_EDGE('',*,*,#2406,.F.);
#3424=ORIENTED_EDGE('',*,*,#2578,.F.);
#3425=ORIENTED_EDGE('',*,*,#2411,.F.);
#3426=ORIENTED_EDGE('',*,*,#2579,.F.);
#3427=ORIENTED_EDGE('',*,*,#2569,.T.);
#3428=ORIENTED_EDGE('',*,*,#2573,.T.);
#3429=ORIENTED_EDGE('',*,*,#2567,.T.);
#3430=ORIENTED_EDGE('',*,*,#2564,.T.);
#3431=ORIENTED_EDGE('',*,*,#2561,.T.);
#3432=ORIENTED_EDGE('',*,*,#2558,.T.);
#3433=ORIENTED_EDGE('',*,*,#2555,.T.);
#3434=ORIENTED_EDGE('',*,*,#2552,.T.);
#3435=ORIENTED_EDGE('',*,*,#2549,.T.);
#3436=ORIENTED_EDGE('',*,*,#2546,.T.);
#3437=ORIENTED_EDGE('',*,*,#2543,.T.);
#3438=ORIENTED_EDGE('',*,*,#2580,.T.);
#3439=ORIENTED_EDGE('',*,*,#2581,.T.);
#3440=ORIENTED_EDGE('',*,*,#2582,.T.);
#3441=ORIENTED_EDGE('',*,*,#2583,.T.);
#3442=ORIENTED_EDGE('',*,*,#2584,.T.);
#3443=ORIENTED_EDGE('',*,*,#2538,.T.);
#3444=ORIENTED_EDGE('',*,*,#2585,.T.);
#3445=ORIENTED_EDGE('',*,*,#2442,.T.);
#3446=ORIENTED_EDGE('',*,*,#2575,.T.);
#3447=ORIENTED_EDGE('',*,*,#2570,.T.);
#3448=ORIENTED_EDGE('',*,*,#2579,.T.);
#3449=ORIENTED_EDGE('',*,*,#2410,.T.);
#3450=ORIENTED_EDGE('',*,*,#2586,.T.);
#3451=ORIENTED_EDGE('',*,*,#2506,.T.);
#3452=ORIENTED_EDGE('',*,*,#2587,.T.);
#3453=ORIENTED_EDGE('',*,*,#2378,.T.);
#3454=ORIENTED_EDGE('',*,*,#2588,.T.);
#3455=ORIENTED_EDGE('',*,*,#2474,.T.);
#3456=ORIENTED_EDGE('',*,*,#2589,.T.);
#3457=ORIENTED_EDGE('',*,*,#2346,.T.);
#3458=ORIENTED_EDGE('',*,*,#2536,.T.);
#3459=ORIENTED_EDGE('',*,*,#2590,.T.);
#3460=ORIENTED_EDGE('',*,*,#2533,.F.);
#3461=ORIENTED_EDGE('',*,*,#2591,.F.);
#3462=ORIENTED_EDGE('',*,*,#2592,.F.);
#3463=ORIENTED_EDGE('',*,*,#2509,.F.);
#3464=ORIENTED_EDGE('',*,*,#2513,.F.);
#3465=ORIENTED_EDGE('',*,*,#2516,.F.);
#3466=ORIENTED_EDGE('',*,*,#2519,.F.);
#3467=ORIENTED_EDGE('',*,*,#2522,.F.);
#3468=ORIENTED_EDGE('',*,*,#2525,.F.);
#3469=ORIENTED_EDGE('',*,*,#2528,.F.);
#3470=ORIENTED_EDGE('',*,*,#2531,.F.);
#3471=ORIENTED_EDGE('',*,*,#2534,.F.);
#3472=ORIENTED_EDGE('',*,*,#2590,.F.);
#3473=ORIENTED_EDGE('',*,*,#2539,.F.);
#3474=ORIENTED_EDGE('',*,*,#2584,.F.);
#3475=ORIENTED_EDGE('',*,*,#2441,.F.);
#3476=ORIENTED_EDGE('',*,*,#2593,.F.);
#3477=ORIENTED_EDGE('',*,*,#2439,.F.);
#3478=ORIENTED_EDGE('',*,*,#2436,.F.);
#3479=ORIENTED_EDGE('',*,*,#2433,.F.);
#3480=ORIENTED_EDGE('',*,*,#2430,.F.);
#3481=ORIENTED_EDGE('',*,*,#2427,.F.);
#3482=ORIENTED_EDGE('',*,*,#2424,.F.);
#3483=ORIENTED_EDGE('',*,*,#2421,.F.);
#3484=ORIENTED_EDGE('',*,*,#2418,.F.);
#3485=ORIENTED_EDGE('',*,*,#2415,.F.);
#3486=ORIENTED_EDGE('',*,*,#2594,.F.);
#3487=ORIENTED_EDGE('',*,*,#2413,.F.);
#3488=ORIENTED_EDGE('',*,*,#2417,.F.);
#3489=ORIENTED_EDGE('',*,*,#2420,.F.);
#3490=ORIENTED_EDGE('',*,*,#2423,.F.);
#3491=ORIENTED_EDGE('',*,*,#2426,.F.);
#3492=ORIENTED_EDGE('',*,*,#2429,.F.);
#3493=ORIENTED_EDGE('',*,*,#2432,.F.);
#3494=ORIENTED_EDGE('',*,*,#2435,.F.);
#3495=ORIENTED_EDGE('',*,*,#2438,.F.);
#3496=ORIENTED_EDGE('',*,*,#2595,.F.);
#3497=ORIENTED_EDGE('',*,*,#2443,.F.);
#3498=ORIENTED_EDGE('',*,*,#2585,.F.);
#3499=ORIENTED_EDGE('',*,*,#2537,.T.);
#3500=ORIENTED_EDGE('',*,*,#2591,.T.);
#3501=ORIENTED_EDGE('',*,*,#2535,.T.);
#3502=ORIENTED_EDGE('',*,*,#2532,.T.);
#3503=ORIENTED_EDGE('',*,*,#2529,.T.);
#3504=ORIENTED_EDGE('',*,*,#2526,.T.);
#3505=ORIENTED_EDGE('',*,*,#2523,.T.);
#3506=ORIENTED_EDGE('',*,*,#2520,.T.);
#3507=ORIENTED_EDGE('',*,*,#2517,.T.);
#3508=ORIENTED_EDGE('',*,*,#2514,.T.);
#3509=ORIENTED_EDGE('',*,*,#2511,.T.);
#3510=ORIENTED_EDGE('',*,*,#2504,.T.);
#3511=ORIENTED_EDGE('',*,*,#2596,.T.);
#3512=ORIENTED_EDGE('',*,*,#2501,.F.);
#3513=ORIENTED_EDGE('',*,*,#2597,.F.);
#3514=ORIENTED_EDGE('',*,*,#2598,.F.);
#3515=ORIENTED_EDGE('',*,*,#2477,.F.);
#3516=ORIENTED_EDGE('',*,*,#2481,.F.);
#3517=ORIENTED_EDGE('',*,*,#2484,.F.);
#3518=ORIENTED_EDGE('',*,*,#2487,.F.);
#3519=ORIENTED_EDGE('',*,*,#2490,.F.);
#3520=ORIENTED_EDGE('',*,*,#2493,.F.);
#3521=ORIENTED_EDGE('',*,*,#2496,.F.);
#3522=ORIENTED_EDGE('',*,*,#2499,.F.);
#3523=ORIENTED_EDGE('',*,*,#2502,.F.);
#3524=ORIENTED_EDGE('',*,*,#2596,.F.);
#3525=ORIENTED_EDGE('',*,*,#2507,.F.);
#3526=ORIENTED_EDGE('',*,*,#2586,.F.);
#3527=ORIENTED_EDGE('',*,*,#2377,.F.);
#3528=ORIENTED_EDGE('',*,*,#2599,.F.);
#3529=ORIENTED_EDGE('',*,*,#2375,.F.);
#3530=ORIENTED_EDGE('',*,*,#2372,.F.);
#3531=ORIENTED_EDGE('',*,*,#2369,.F.);
#3532=ORIENTED_EDGE('',*,*,#2366,.F.);
#3533=ORIENTED_EDGE('',*,*,#2363,.F.);
#3534=ORIENTED_EDGE('',*,*,#2360,.F.);
#3535=ORIENTED_EDGE('',*,*,#2357,.F.);
#3536=ORIENTED_EDGE('',*,*,#2354,.F.);
#3537=ORIENTED_EDGE('',*,*,#2351,.F.);
#3538=ORIENTED_EDGE('',*,*,#2600,.F.);
#3539=ORIENTED_EDGE('',*,*,#2349,.F.);
#3540=ORIENTED_EDGE('',*,*,#2353,.F.);
#3541=ORIENTED_EDGE('',*,*,#2356,.F.);
#3542=ORIENTED_EDGE('',*,*,#2359,.F.);
#3543=ORIENTED_EDGE('',*,*,#2362,.F.);
#3544=ORIENTED_EDGE('',*,*,#2365,.F.);
#3545=ORIENTED_EDGE('',*,*,#2368,.F.);
#3546=ORIENTED_EDGE('',*,*,#2371,.F.);
#3547=ORIENTED_EDGE('',*,*,#2374,.F.);
#3548=ORIENTED_EDGE('',*,*,#2601,.F.);
#3549=ORIENTED_EDGE('',*,*,#2379,.F.);
#3550=ORIENTED_EDGE('',*,*,#2587,.F.);
#3551=ORIENTED_EDGE('',*,*,#2505,.T.);
#3552=ORIENTED_EDGE('',*,*,#2597,.T.);
#3553=ORIENTED_EDGE('',*,*,#2503,.T.);
#3554=ORIENTED_EDGE('',*,*,#2500,.T.);
#3555=ORIENTED_EDGE('',*,*,#2497,.T.);
#3556=ORIENTED_EDGE('',*,*,#2494,.T.);
#3557=ORIENTED_EDGE('',*,*,#2491,.T.);
#3558=ORIENTED_EDGE('',*,*,#2488,.T.);
#3559=ORIENTED_EDGE('',*,*,#2485,.T.);
#3560=ORIENTED_EDGE('',*,*,#2482,.T.);
#3561=ORIENTED_EDGE('',*,*,#2479,.T.);
#3562=ORIENTED_EDGE('',*,*,#2472,.T.);
#3563=ORIENTED_EDGE('',*,*,#2602,.T.);
#3564=ORIENTED_EDGE('',*,*,#2469,.F.);
#3565=ORIENTED_EDGE('',*,*,#2603,.F.);
#3566=ORIENTED_EDGE('',*,*,#2604,.F.);
#3567=ORIENTED_EDGE('',*,*,#2445,.F.);
#3568=ORIENTED_EDGE('',*,*,#2449,.F.);
#3569=ORIENTED_EDGE('',*,*,#2452,.F.);
#3570=ORIENTED_EDGE('',*,*,#2455,.F.);
#3571=ORIENTED_EDGE('',*,*,#2458,.F.);
#3572=ORIENTED_EDGE('',*,*,#2461,.F.);
#3573=ORIENTED_EDGE('',*,*,#2464,.F.);
#3574=ORIENTED_EDGE('',*,*,#2467,.F.);
#3575=ORIENTED_EDGE('',*,*,#2470,.F.);
#3576=ORIENTED_EDGE('',*,*,#2602,.F.);
#3577=ORIENTED_EDGE('',*,*,#2475,.F.);
#3578=ORIENTED_EDGE('',*,*,#2588,.F.);
#3579=ORIENTED_EDGE('',*,*,#2345,.F.);
#3580=ORIENTED_EDGE('',*,*,#2605,.F.);
#3581=ORIENTED_EDGE('',*,*,#2343,.F.);
#3582=ORIENTED_EDGE('',*,*,#2340,.F.);
#3583=ORIENTED_EDGE('',*,*,#2337,.F.);
#3584=ORIENTED_EDGE('',*,*,#2334,.F.);
#3585=ORIENTED_EDGE('',*,*,#2331,.F.);
#3586=ORIENTED_EDGE('',*,*,#2328,.F.);
#3587=ORIENTED_EDGE('',*,*,#2325,.F.);
#3588=ORIENTED_EDGE('',*,*,#2322,.F.);
#3589=ORIENTED_EDGE('',*,*,#2319,.F.);
#3590=ORIENTED_EDGE('',*,*,#2606,.F.);
#3591=ORIENTED_EDGE('',*,*,#2317,.F.);
#3592=ORIENTED_EDGE('',*,*,#2321,.F.);
#3593=ORIENTED_EDGE('',*,*,#2324,.F.);
#3594=ORIENTED_EDGE('',*,*,#2327,.F.);
#3595=ORIENTED_EDGE('',*,*,#2330,.F.);
#3596=ORIENTED_EDGE('',*,*,#2333,.F.);
#3597=ORIENTED_EDGE('',*,*,#2336,.F.);
#3598=ORIENTED_EDGE('',*,*,#2339,.F.);
#3599=ORIENTED_EDGE('',*,*,#2342,.F.);
#3600=ORIENTED_EDGE('',*,*,#2607,.F.);
#3601=ORIENTED_EDGE('',*,*,#2347,.F.);
#3602=ORIENTED_EDGE('',*,*,#2589,.F.);
#3603=ORIENTED_EDGE('',*,*,#2473,.T.);
#3604=ORIENTED_EDGE('',*,*,#2603,.T.);
#3605=ORIENTED_EDGE('',*,*,#2471,.T.);
#3606=ORIENTED_EDGE('',*,*,#2468,.T.);
#3607=ORIENTED_EDGE('',*,*,#2465,.T.);
#3608=ORIENTED_EDGE('',*,*,#2462,.T.);
#3609=ORIENTED_EDGE('',*,*,#2459,.T.);
#3610=ORIENTED_EDGE('',*,*,#2456,.T.);
#3611=ORIENTED_EDGE('',*,*,#2453,.T.);
#3612=ORIENTED_EDGE('',*,*,#2450,.T.);
#3613=ORIENTED_EDGE('',*,*,#2447,.T.);
#3614=ORIENTED_EDGE('',*,*,#2440,.T.);
#3615=ORIENTED_EDGE('',*,*,#2595,.T.);
#3616=ORIENTED_EDGE('',*,*,#2437,.F.);
#3617=ORIENTED_EDGE('',*,*,#2593,.T.);
#3618=ORIENTED_EDGE('',*,*,#2408,.T.);
#3619=ORIENTED_EDGE('',*,*,#2578,.T.);
#3620=ORIENTED_EDGE('',*,*,#2405,.F.);
#3621=ORIENTED_EDGE('',*,*,#2576,.T.);
#3622=ORIENTED_EDGE('',*,*,#2376,.T.);
#3623=ORIENTED_EDGE('',*,*,#2601,.T.);
#3624=ORIENTED_EDGE('',*,*,#2373,.F.);
#3625=ORIENTED_EDGE('',*,*,#2599,.T.);
#3626=ORIENTED_EDGE('',*,*,#2344,.T.);
#3627=ORIENTED_EDGE('',*,*,#2607,.T.);
#3628=ORIENTED_EDGE('',*,*,#2341,.F.);
#3629=ORIENTED_EDGE('',*,*,#2605,.T.);
#3630=ORIENTED_EDGE('',*,*,#2608,.T.);
#3631=ORIENTED_EDGE('',*,*,#2609,.T.);
#3632=ORIENTED_EDGE('',*,*,#2583,.F.);
#3633=ORIENTED_EDGE('',*,*,#2610,.F.);
#3634=ORIENTED_EDGE('',*,*,#2611,.T.);
#3635=ORIENTED_EDGE('',*,*,#2610,.T.);
#3636=ORIENTED_EDGE('',*,*,#2582,.F.);
#3637=ORIENTED_EDGE('',*,*,#2612,.F.);
#3638=ORIENTED_EDGE('',*,*,#2613,.T.);
#3639=ORIENTED_EDGE('',*,*,#2612,.T.);
#3640=ORIENTED_EDGE('',*,*,#2581,.F.);
#3641=ORIENTED_EDGE('',*,*,#2614,.F.);
#3642=ORIENTED_EDGE('',*,*,#2615,.T.);
#3643=ORIENTED_EDGE('',*,*,#2614,.T.);
#3644=ORIENTED_EDGE('',*,*,#2580,.F.);
#3645=ORIENTED_EDGE('',*,*,#2609,.F.);
#3646=ORIENTED_EDGE('',*,*,#2615,.F.);
#3647=ORIENTED_EDGE('',*,*,#2608,.F.);
#3648=ORIENTED_EDGE('',*,*,#2611,.F.);
#3649=ORIENTED_EDGE('',*,*,#2613,.F.);
#3650=ORIENTED_EDGE('',*,*,#2574,.T.);
#3651=ORIENTED_EDGE('',*,*,#2382,.T.);
#3652=ORIENTED_EDGE('',*,*,#2577,.T.);
#3653=ORIENTED_EDGE('',*,*,#2542,.T.);
#3654=ORIENTED_EDGE('',*,*,#2592,.T.);
#3655=ORIENTED_EDGE('',*,*,#2414,.T.);
#3656=ORIENTED_EDGE('',*,*,#2594,.T.);
#3657=ORIENTED_EDGE('',*,*,#2510,.T.);
#3658=ORIENTED_EDGE('',*,*,#2598,.T.);
#3659=ORIENTED_EDGE('',*,*,#2350,.T.);
#3660=ORIENTED_EDGE('',*,*,#2600,.T.);
#3661=ORIENTED_EDGE('',*,*,#2478,.T.);
#3662=ORIENTED_EDGE('',*,*,#2604,.T.);
#3663=ORIENTED_EDGE('',*,*,#2318,.T.);
#3664=ORIENTED_EDGE('',*,*,#2606,.T.);
#3665=ORIENTED_EDGE('',*,*,#2446,.T.);
#3826=CYLINDRICAL_SURFACE('',#4487,2.5175);
#3827=CYLINDRICAL_SURFACE('',#4489,2.5175);
#3828=CYLINDRICAL_SURFACE('',#4490,2.5175);
#3829=CYLINDRICAL_SURFACE('',#4491,2.5175);
#3830=CYLINDRICAL_SURFACE('',#4492,2.5175);
#3831=CYLINDRICAL_SURFACE('',#4493,2.5175);
#3832=CYLINDRICAL_SURFACE('',#4494,2.5175);
#3833=CYLINDRICAL_SURFACE('',#4495,2.5175);
#3834=CYLINDRICAL_SURFACE('',#4496,2.5175);
#3835=CYLINDRICAL_SURFACE('',#4497,2.5175);
#3836=CYLINDRICAL_SURFACE('',#4499,2.5175);
#3837=CYLINDRICAL_SURFACE('',#4501,2.5175);
#3838=CYLINDRICAL_SURFACE('',#4502,2.5175);
#3839=CYLINDRICAL_SURFACE('',#4503,2.5175);
#3840=CYLINDRICAL_SURFACE('',#4504,2.5175);
#3841=CYLINDRICAL_SURFACE('',#4505,2.5175);
#3842=CYLINDRICAL_SURFACE('',#4506,2.5175);
#3843=CYLINDRICAL_SURFACE('',#4507,2.5175);
#3844=CYLINDRICAL_SURFACE('',#4508,2.5175);
#3845=CYLINDRICAL_SURFACE('',#4509,2.5175);
#3846=CYLINDRICAL_SURFACE('',#4511,2.5175);
#3847=CYLINDRICAL_SURFACE('',#4513,2.5175);
#3848=CYLINDRICAL_SURFACE('',#4514,2.5175);
#3849=CYLINDRICAL_SURFACE('',#4515,2.5175);
#3850=CYLINDRICAL_SURFACE('',#4516,2.5175);
#3851=CYLINDRICAL_SURFACE('',#4517,2.5175);
#3852=CYLINDRICAL_SURFACE('',#4518,2.5175);
#3853=CYLINDRICAL_SURFACE('',#4519,2.5175);
#3854=CYLINDRICAL_SURFACE('',#4520,2.5175);
#3855=CYLINDRICAL_SURFACE('',#4521,2.5175);
#3856=CYLINDRICAL_SURFACE('',#4523,2.5175);
#3857=CYLINDRICAL_SURFACE('',#4525,2.5175);
#3858=CYLINDRICAL_SURFACE('',#4526,2.5175);
#3859=CYLINDRICAL_SURFACE('',#4527,2.5175);
#3860=CYLINDRICAL_SURFACE('',#4528,2.5175);
#3861=CYLINDRICAL_SURFACE('',#4529,2.5175);
#3862=CYLINDRICAL_SURFACE('',#4530,2.5175);
#3863=CYLINDRICAL_SURFACE('',#4531,2.5175);
#3864=CYLINDRICAL_SURFACE('',#4532,2.5175);
#3865=CYLINDRICAL_SURFACE('',#4533,2.5175);
#3866=CYLINDRICAL_SURFACE('',#4535,3.0735);
#3867=CYLINDRICAL_SURFACE('',#4537,3.0735);
#3868=CYLINDRICAL_SURFACE('',#4538,3.0735);
#3869=CYLINDRICAL_SURFACE('',#4539,3.0735);
#3870=CYLINDRICAL_SURFACE('',#4540,3.0735);
#3871=CYLINDRICAL_SURFACE('',#4541,3.0735);
#3872=CYLINDRICAL_SURFACE('',#4542,3.0735);
#3873=CYLINDRICAL_SURFACE('',#4543,3.0735);
#3874=CYLINDRICAL_SURFACE('',#4544,3.0735);
#3875=CYLINDRICAL_SURFACE('',#4545,3.0735);
#3876=CYLINDRICAL_SURFACE('',#4547,3.07350000000001);
#3877=CYLINDRICAL_SURFACE('',#4549,3.07350000000001);
#3878=CYLINDRICAL_SURFACE('',#4550,3.07350000000001);
#3879=CYLINDRICAL_SURFACE('',#4551,3.07350000000001);
#3880=CYLINDRICAL_SURFACE('',#4552,3.07350000000001);
#3881=CYLINDRICAL_SURFACE('',#4553,3.07350000000001);
#3882=CYLINDRICAL_SURFACE('',#4554,3.07350000000001);
#3883=CYLINDRICAL_SURFACE('',#4555,3.07350000000001);
#3884=CYLINDRICAL_SURFACE('',#4556,3.07350000000001);
#3885=CYLINDRICAL_SURFACE('',#4557,3.07350000000001);
#3886=CYLINDRICAL_SURFACE('',#4559,3.0735);
#3887=CYLINDRICAL_SURFACE('',#4561,3.0735);
#3888=CYLINDRICAL_SURFACE('',#4562,3.0735);
#3889=CYLINDRICAL_SURFACE('',#4563,3.0735);
#3890=CYLINDRICAL_SURFACE('',#4564,3.0735);
#3891=CYLINDRICAL_SURFACE('',#4565,3.0735);
#3892=CYLINDRICAL_SURFACE('',#4566,3.0735);
#3893=CYLINDRICAL_SURFACE('',#4567,3.0735);
#3894=CYLINDRICAL_SURFACE('',#4568,3.0735);
#3895=CYLINDRICAL_SURFACE('',#4569,3.0735);
#3896=CYLINDRICAL_SURFACE('',#4571,3.07350000000001);
#3897=CYLINDRICAL_SURFACE('',#4573,3.07350000000001);
#3898=CYLINDRICAL_SURFACE('',#4574,3.07350000000001);
#3899=CYLINDRICAL_SURFACE('',#4575,3.07350000000001);
#3900=CYLINDRICAL_SURFACE('',#4576,3.07350000000001);
#3901=CYLINDRICAL_SURFACE('',#4577,3.07350000000001);
#3902=CYLINDRICAL_SURFACE('',#4578,3.07350000000001);
#3903=CYLINDRICAL_SURFACE('',#4579,3.07350000000001);
#3904=CYLINDRICAL_SURFACE('',#4580,3.07350000000001);
#3905=CYLINDRICAL_SURFACE('',#4581,3.07350000000001);
#3906=CYLINDRICAL_SURFACE('',#4583,3.07350000000001);
#3907=CYLINDRICAL_SURFACE('',#4585,3.0735);
#3908=CYLINDRICAL_SURFACE('',#4586,3.07350000000001);
#3909=CYLINDRICAL_SURFACE('',#4587,3.0735);
#3910=CYLINDRICAL_SURFACE('',#4588,2.5175);
#3911=CYLINDRICAL_SURFACE('',#4589,2.5175);
#3912=CYLINDRICAL_SURFACE('',#4590,2.5175);
#3913=CYLINDRICAL_SURFACE('',#4591,2.5175);
#4008=ADVANCED_FACE('',(#711),#3826,.F.);
#4009=ADVANCED_FACE('',(#712),#3827,.F.);
#4010=ADVANCED_FACE('',(#713),#3828,.F.);
#4011=ADVANCED_FACE('',(#714),#3829,.F.);
#4012=ADVANCED_FACE('',(#715),#3830,.F.);
#4013=ADVANCED_FACE('',(#716),#3831,.F.);
#4014=ADVANCED_FACE('',(#717),#3832,.F.);
#4015=ADVANCED_FACE('',(#718),#3833,.F.);
#4016=ADVANCED_FACE('',(#719),#3834,.F.);
#4017=ADVANCED_FACE('',(#720),#3835,.F.);
#4018=ADVANCED_FACE('',(#721),#3836,.F.);
#4019=ADVANCED_FACE('',(#722),#3837,.F.);
#4020=ADVANCED_FACE('',(#723),#3838,.F.);
#4021=ADVANCED_FACE('',(#724),#3839,.F.);
#4022=ADVANCED_FACE('',(#725),#3840,.F.);
#4023=ADVANCED_FACE('',(#726),#3841,.F.);
#4024=ADVANCED_FACE('',(#727),#3842,.F.);
#4025=ADVANCED_FACE('',(#728),#3843,.F.);
#4026=ADVANCED_FACE('',(#729),#3844,.F.);
#4027=ADVANCED_FACE('',(#730),#3845,.F.);
#4028=ADVANCED_FACE('',(#731),#3846,.F.);
#4029=ADVANCED_FACE('',(#732),#3847,.F.);
#4030=ADVANCED_FACE('',(#733),#3848,.F.);
#4031=ADVANCED_FACE('',(#734),#3849,.F.);
#4032=ADVANCED_FACE('',(#735),#3850,.F.);
#4033=ADVANCED_FACE('',(#736),#3851,.F.);
#4034=ADVANCED_FACE('',(#737),#3852,.F.);
#4035=ADVANCED_FACE('',(#738),#3853,.F.);
#4036=ADVANCED_FACE('',(#739),#3854,.F.);
#4037=ADVANCED_FACE('',(#740),#3855,.F.);
#4038=ADVANCED_FACE('',(#741),#3856,.F.);
#4039=ADVANCED_FACE('',(#742),#3857,.F.);
#4040=ADVANCED_FACE('',(#743),#3858,.F.);
#4041=ADVANCED_FACE('',(#744),#3859,.F.);
#4042=ADVANCED_FACE('',(#745),#3860,.F.);
#4043=ADVANCED_FACE('',(#746),#3861,.F.);
#4044=ADVANCED_FACE('',(#747),#3862,.F.);
#4045=ADVANCED_FACE('',(#748),#3863,.F.);
#4046=ADVANCED_FACE('',(#749),#3864,.F.);
#4047=ADVANCED_FACE('',(#750),#3865,.F.);
#4048=ADVANCED_FACE('',(#751),#3866,.F.);
#4049=ADVANCED_FACE('',(#752),#3867,.F.);
#4050=ADVANCED_FACE('',(#753),#3868,.F.);
#4051=ADVANCED_FACE('',(#754),#3869,.F.);
#4052=ADVANCED_FACE('',(#755),#3870,.F.);
#4053=ADVANCED_FACE('',(#756),#3871,.F.);
#4054=ADVANCED_FACE('',(#757),#3872,.F.);
#4055=ADVANCED_FACE('',(#758),#3873,.F.);
#4056=ADVANCED_FACE('',(#759),#3874,.F.);
#4057=ADVANCED_FACE('',(#760),#3875,.F.);
#4058=ADVANCED_FACE('',(#761),#3876,.F.);
#4059=ADVANCED_FACE('',(#762),#3877,.F.);
#4060=ADVANCED_FACE('',(#763),#3878,.F.);
#4061=ADVANCED_FACE('',(#764),#3879,.F.);
#4062=ADVANCED_FACE('',(#765),#3880,.F.);
#4063=ADVANCED_FACE('',(#766),#3881,.F.);
#4064=ADVANCED_FACE('',(#767),#3882,.F.);
#4065=ADVANCED_FACE('',(#768),#3883,.F.);
#4066=ADVANCED_FACE('',(#769),#3884,.F.);
#4067=ADVANCED_FACE('',(#770),#3885,.F.);
#4068=ADVANCED_FACE('',(#771),#3886,.F.);
#4069=ADVANCED_FACE('',(#772),#3887,.F.);
#4070=ADVANCED_FACE('',(#773),#3888,.F.);
#4071=ADVANCED_FACE('',(#774),#3889,.F.);
#4072=ADVANCED_FACE('',(#775),#3890,.F.);
#4073=ADVANCED_FACE('',(#776),#3891,.F.);
#4074=ADVANCED_FACE('',(#777),#3892,.F.);
#4075=ADVANCED_FACE('',(#778),#3893,.F.);
#4076=ADVANCED_FACE('',(#779),#3894,.F.);
#4077=ADVANCED_FACE('',(#780),#3895,.F.);
#4078=ADVANCED_FACE('',(#781),#3896,.F.);
#4079=ADVANCED_FACE('',(#782),#3897,.F.);
#4080=ADVANCED_FACE('',(#783),#3898,.F.);
#4081=ADVANCED_FACE('',(#784),#3899,.F.);
#4082=ADVANCED_FACE('',(#785),#3900,.F.);
#4083=ADVANCED_FACE('',(#786),#3901,.F.);
#4084=ADVANCED_FACE('',(#787),#3902,.F.);
#4085=ADVANCED_FACE('',(#788),#3903,.F.);
#4086=ADVANCED_FACE('',(#789),#3904,.F.);
#4087=ADVANCED_FACE('',(#790),#3905,.F.);
#4088=ADVANCED_FACE('',(#791),#3906,.F.);
#4089=ADVANCED_FACE('',(#792),#239,.F.);
#4090=ADVANCED_FACE('',(#793),#240,.F.);
#4091=ADVANCED_FACE('',(#794,#531,#532,#533,#534),#602,.T.);
#4092=ADVANCED_FACE('',(#795),#3907,.F.);
#4093=ADVANCED_FACE('',(#796),#241,.F.);
#4094=ADVANCED_FACE('',(#797),#242,.F.);
#4095=ADVANCED_FACE('',(#798),#3908,.F.);
#4096=ADVANCED_FACE('',(#799),#243,.F.);
#4097=ADVANCED_FACE('',(#800),#244,.F.);
#4098=ADVANCED_FACE('',(#801),#3909,.F.);
#4099=ADVANCED_FACE('',(#802),#245,.F.);
#4100=ADVANCED_FACE('',(#803),#246,.F.);
#4101=ADVANCED_FACE('',(#804),#3910,.F.);
#4102=ADVANCED_FACE('',(#805),#3911,.F.);
#4103=ADVANCED_FACE('',(#806),#3912,.F.);
#4104=ADVANCED_FACE('',(#807),#3913,.F.);
#4105=ADVANCED_FACE('',(#808),#603,.T.);
#4106=ADVANCED_FACE('',(#809),#604,.T.);
#4107=ADVANCED_FACE('',(#810),#605,.T.);
#4108=ADVANCED_FACE('',(#811),#606,.T.);
#4109=ADVANCED_FACE('',(#812,#535,#536,#537,#538),#607,.F.);
#4158=CLOSED_SHELL('',(#4008,#4009,#4010,#4011,#4012,#4013,#4014,#4015,
#4016,#4017,#4018,#4019,#4020,#4021,#4022,#4023,#4024,#4025,#4026,#4027,
#4028,#4029,#4030,#4031,#4032,#4033,#4034,#4035,#4036,#4037,#4038,#4039,
#4040,#4041,#4042,#4043,#4044,#4045,#4046,#4047,#4048,#4049,#4050,#4051,
#4052,#4053,#4054,#4055,#4056,#4057,#4058,#4059,#4060,#4061,#4062,#4063,
#4064,#4065,#4066,#4067,#4068,#4069,#4070,#4071,#4072,#4073,#4074,#4075,
#4076,#4077,#4078,#4079,#4080,#4081,#4082,#4083,#4084,#4085,#4086,#4087,
#4088,#4089,#4090,#4091,#4092,#4093,#4094,#4095,#4096,#4097,#4098,#4099,
#4100,#4101,#4102,#4103,#4104,#4105,#4106,#4107,#4108,#4109));
#4486=AXIS2_PLACEMENT_3D('',#6185,#5155,#5156);
#4487=AXIS2_PLACEMENT_3D('',#6186,#5157,#5158);
#4488=AXIS2_PLACEMENT_3D('',#6196,#5160,#5161);
#4489=AXIS2_PLACEMENT_3D('',#6207,#5162,#5163);
#4490=AXIS2_PLACEMENT_3D('',#6258,#5165,#5166);
#4491=AXIS2_PLACEMENT_3D('',#6309,#5168,#5169);
#4492=AXIS2_PLACEMENT_3D('',#6357,#5171,#5172);
#4493=AXIS2_PLACEMENT_3D('',#6405,#5174,#5175);
#4494=AXIS2_PLACEMENT_3D('',#6456,#5177,#5178);
#4495=AXIS2_PLACEMENT_3D('',#6507,#5180,#5181);
#4496=AXIS2_PLACEMENT_3D('',#6555,#5183,#5184);
#4497=AXIS2_PLACEMENT_3D('',#6606,#5186,#5187);
#4498=AXIS2_PLACEMENT_3D('',#6625,#5189,#5190);
#4499=AXIS2_PLACEMENT_3D('',#6645,#5191,#5192);
#4500=AXIS2_PLACEMENT_3D('',#6655,#5194,#5195);
#4501=AXIS2_PLACEMENT_3D('',#6666,#5196,#5197);
#4502=AXIS2_PLACEMENT_3D('',#6717,#5199,#5200);
#4503=AXIS2_PLACEMENT_3D('',#6768,#5202,#5203);
#4504=AXIS2_PLACEMENT_3D('',#6816,#5205,#5206);
#4505=AXIS2_PLACEMENT_3D('',#6864,#5208,#5209);
#4506=AXIS2_PLACEMENT_3D('',#6915,#5211,#5212);
#4507=AXIS2_PLACEMENT_3D('',#6966,#5214,#5215);
#4508=AXIS2_PLACEMENT_3D('',#7014,#5217,#5218);
#4509=AXIS2_PLACEMENT_3D('',#7065,#5220,#5221);
#4510=AXIS2_PLACEMENT_3D('',#7084,#5223,#5224);
#4511=AXIS2_PLACEMENT_3D('',#7104,#5225,#5226);
#4512=AXIS2_PLACEMENT_3D('',#7114,#5228,#5229);
#4513=AXIS2_PLACEMENT_3D('',#7125,#5230,#5231);
#4514=AXIS2_PLACEMENT_3D('',#7176,#5233,#5234);
#4515=AXIS2_PLACEMENT_3D('',#7227,#5236,#5237);
#4516=AXIS2_PLACEMENT_3D('',#7275,#5239,#5240);
#4517=AXIS2_PLACEMENT_3D('',#7323,#5242,#5243);
#4518=AXIS2_PLACEMENT_3D('',#7374,#5245,#5246);
#4519=AXIS2_PLACEMENT_3D('',#7425,#5248,#5249);
#4520=AXIS2_PLACEMENT_3D('',#7473,#5251,#5252);
#4521=AXIS2_PLACEMENT_3D('',#7524,#5254,#5255);
#4522=AXIS2_PLACEMENT_3D('',#7543,#5257,#5258);
#4523=AXIS2_PLACEMENT_3D('',#7563,#5259,#5260);
#4524=AXIS2_PLACEMENT_3D('',#7573,#5262,#5263);
#4525=AXIS2_PLACEMENT_3D('',#7584,#5264,#5265);
#4526=AXIS2_PLACEMENT_3D('',#7635,#5267,#5268);
#4527=AXIS2_PLACEMENT_3D('',#7686,#5270,#5271);
#4528=AXIS2_PLACEMENT_3D('',#7734,#5273,#5274);
#4529=AXIS2_PLACEMENT_3D('',#7782,#5276,#5277);
#4530=AXIS2_PLACEMENT_3D('',#7833,#5279,#5280);
#4531=AXIS2_PLACEMENT_3D('',#7884,#5282,#5283);
#4532=AXIS2_PLACEMENT_3D('',#7932,#5285,#5286);
#4533=AXIS2_PLACEMENT_3D('',#7983,#5288,#5289);
#4534=AXIS2_PLACEMENT_3D('',#8002,#5291,#5292);
#4535=AXIS2_PLACEMENT_3D('',#8022,#5293,#5294);
#4536=AXIS2_PLACEMENT_3D('',#8036,#5296,#5297);
#4537=AXIS2_PLACEMENT_3D('',#8046,#5298,#5299);
#4538=AXIS2_PLACEMENT_3D('',#8070,#5301,#5302);
#4539=AXIS2_PLACEMENT_3D('',#8095,#5304,#5305);
#4540=AXIS2_PLACEMENT_3D('',#8119,#5307,#5308);
#4541=AXIS2_PLACEMENT_3D('',#8144,#5310,#5311);
#4542=AXIS2_PLACEMENT_3D('',#8168,#5313,#5314);
#4543=AXIS2_PLACEMENT_3D('',#8193,#5316,#5317);
#4544=AXIS2_PLACEMENT_3D('',#8218,#5319,#5320);
#4545=AXIS2_PLACEMENT_3D('',#8242,#5322,#5323);
#4546=AXIS2_PLACEMENT_3D('',#8253,#5325,#5326);
#4547=AXIS2_PLACEMENT_3D('',#8259,#5327,#5328);
#4548=AXIS2_PLACEMENT_3D('',#8273,#5330,#5331);
#4549=AXIS2_PLACEMENT_3D('',#8283,#5332,#5333);
#4550=AXIS2_PLACEMENT_3D('',#8307,#5335,#5336);
#4551=AXIS2_PLACEMENT_3D('',#8332,#5338,#5339);
#4552=AXIS2_PLACEMENT_3D('',#8356,#5341,#5342);
#4553=AXIS2_PLACEMENT_3D('',#8381,#5344,#5345);
#4554=AXIS2_PLACEMENT_3D('',#8405,#5347,#5348);
#4555=AXIS2_PLACEMENT_3D('',#8430,#5350,#5351);
#4556=AXIS2_PLACEMENT_3D('',#8455,#5353,#5354);
#4557=AXIS2_PLACEMENT_3D('',#8479,#5356,#5357);
#4558=AXIS2_PLACEMENT_3D('',#8490,#5359,#5360);
#4559=AXIS2_PLACEMENT_3D('',#8496,#5361,#5362);
#4560=AXIS2_PLACEMENT_3D('',#8510,#5364,#5365);
#4561=AXIS2_PLACEMENT_3D('',#8520,#5366,#5367);
#4562=AXIS2_PLACEMENT_3D('',#8544,#5369,#5370);
#4563=AXIS2_PLACEMENT_3D('',#8569,#5372,#5373);
#4564=AXIS2_PLACEMENT_3D('',#8593,#5375,#5376);
#4565=AXIS2_PLACEMENT_3D('',#8618,#5378,#5379);
#4566=AXIS2_PLACEMENT_3D('',#8642,#5381,#5382);
#4567=AXIS2_PLACEMENT_3D('',#8667,#5384,#5385);
#4568=AXIS2_PLACEMENT_3D('',#8692,#5387,#5388);
#4569=AXIS2_PLACEMENT_3D('',#8716,#5390,#5391);
#4570=AXIS2_PLACEMENT_3D('',#8727,#5393,#5394);
#4571=AXIS2_PLACEMENT_3D('',#8733,#5395,#5396);
#4572=AXIS2_PLACEMENT_3D('',#8747,#5398,#5399);
#4573=AXIS2_PLACEMENT_3D('',#8757,#5400,#5401);
#4574=AXIS2_PLACEMENT_3D('',#8781,#5403,#5404);
#4575=AXIS2_PLACEMENT_3D('',#8806,#5406,#5407);
#4576=AXIS2_PLACEMENT_3D('',#8830,#5409,#5410);
#4577=AXIS2_PLACEMENT_3D('',#8855,#5412,#5413);
#4578=AXIS2_PLACEMENT_3D('',#8879,#5415,#5416);
#4579=AXIS2_PLACEMENT_3D('',#8904,#5418,#5419);
#4580=AXIS2_PLACEMENT_3D('',#8929,#5421,#5422);
#4581=AXIS2_PLACEMENT_3D('',#8953,#5424,#5425);
#4582=AXIS2_PLACEMENT_3D('',#8964,#5427,#5428);
#4583=AXIS2_PLACEMENT_3D('',#8970,#5429,#5430);
#4584=AXIS2_PLACEMENT_3D('',#9965,#5431,#5432);
#4585=AXIS2_PLACEMENT_3D('',#10547,#5437,#5438);
#4586=AXIS2_PLACEMENT_3D('',#11351,#5439,#5440);
#4587=AXIS2_PLACEMENT_3D('',#12155,#5441,#5442);
#4588=AXIS2_PLACEMENT_3D('',#12959,#5443,#5444);
#4589=AXIS2_PLACEMENT_3D('',#12960,#5445,#5446);
#4590=AXIS2_PLACEMENT_3D('',#12961,#5447,#5448);
#4591=AXIS2_PLACEMENT_3D('',#12962,#5449,#5450);
#4592=AXIS2_PLACEMENT_3D('',#12963,#5451,#5452);
#4593=AXIS2_PLACEMENT_3D('',#12969,#5456,#5457);
#4594=AXIS2_PLACEMENT_3D('',#12973,#5460,#5461);
#4595=AXIS2_PLACEMENT_3D('',#12977,#5464,#5465);
#4596=AXIS2_PLACEMENT_3D('',#12979,#5467,#5468);
#5155=DIRECTION('axis',(0.,0.,1.));
#5156=DIRECTION('refdir',(1.,0.,0.));
#5157=DIRECTION('center_axis',(0.,0.,-1.));
#5158=DIRECTION('ref_axis',(-0.346966786786352,0.93787741675933,0.));
#5159=DIRECTION('',(0.,0.,-1.));
#5160=DIRECTION('center_axis',(0.,0.,-1.));
#5161=DIRECTION('ref_axis',(1.,0.,0.));
#5162=DIRECTION('center_axis',(0.,0.,-1.));
#5163=DIRECTION('ref_axis',(1.,0.,0.));
#5164=DIRECTION('',(0.,0.,-1.));
#5165=DIRECTION('center_axis',(0.,0.,-1.));
#5166=DIRECTION('ref_axis',(1.,0.,0.));
#5167=DIRECTION('',(0.,0.,-1.));
#5168=DIRECTION('center_axis',(0.,0.,-1.));
#5169=DIRECTION('ref_axis',(1.,0.,0.));
#5170=DIRECTION('',(0.,0.,-1.));
#5171=DIRECTION('center_axis',(0.,0.,-1.));
#5172=DIRECTION('ref_axis',(1.,0.,0.));
#5173=DIRECTION('',(0.,0.,-1.));
#5174=DIRECTION('center_axis',(0.,0.,-1.));
#5175=DIRECTION('ref_axis',(1.,0.,0.));
#5176=DIRECTION('',(0.,0.,-1.));
#5177=DIRECTION('center_axis',(0.,0.,-1.));
#5178=DIRECTION('ref_axis',(1.,0.,0.));
#5179=DIRECTION('',(0.,0.,-1.));
#5180=DIRECTION('center_axis',(0.,0.,-1.));
#5181=DIRECTION('ref_axis',(1.,0.,0.));
#5182=DIRECTION('',(0.,0.,-1.));
#5183=DIRECTION('center_axis',(0.,0.,-1.));
#5184=DIRECTION('ref_axis',(1.,0.,0.));
#5185=DIRECTION('',(0.,0.,-1.));
#5186=DIRECTION('center_axis',(0.,0.,-1.));
#5187=DIRECTION('ref_axis',(0.937993686897822,-0.346652337854271,0.));
#5188=DIRECTION('',(0.,0.,-1.));
#5189=DIRECTION('center_axis',(0.,0.,-1.));
#5190=DIRECTION('ref_axis',(1.,0.,0.));
#5191=DIRECTION('center_axis',(0.,0.,-1.));
#5192=DIRECTION('ref_axis',(-0.346967010928538,0.937877333838128,0.));
#5193=DIRECTION('',(0.,0.,-1.));
#5194=DIRECTION('center_axis',(0.,0.,-1.));
#5195=DIRECTION('ref_axis',(1.,0.,0.));
#5196=DIRECTION('center_axis',(0.,0.,-1.));
#5197=DIRECTION('ref_axis',(1.,0.,0.));
#5198=DIRECTION('',(0.,0.,-1.));
#5199=DIRECTION('center_axis',(0.,0.,-1.));
#5200=DIRECTION('ref_axis',(1.,0.,0.));
#5201=DIRECTION('',(0.,0.,-1.));
#5202=DIRECTION('center_axis',(0.,0.,-1.));
#5203=DIRECTION('ref_axis',(1.,0.,0.));
#5204=DIRECTION('',(0.,0.,-1.));
#5205=DIRECTION('center_axis',(0.,0.,-1.));
#5206=DIRECTION('ref_axis',(1.,0.,0.));
#5207=DIRECTION('',(0.,0.,-1.));
#5208=DIRECTION('center_axis',(0.,0.,-1.));
#5209=DIRECTION('ref_axis',(1.,0.,0.));
#5210=DIRECTION('',(0.,0.,-1.));
#5211=DIRECTION('center_axis',(0.,0.,-1.));
#5212=DIRECTION('ref_axis',(1.,0.,0.));
#5213=DIRECTION('',(0.,0.,-1.));
#5214=DIRECTION('center_axis',(0.,0.,-1.));
#5215=DIRECTION('ref_axis',(1.,0.,0.));
#5216=DIRECTION('',(0.,0.,-1.));
#5217=DIRECTION('center_axis',(0.,0.,-1.));
#5218=DIRECTION('ref_axis',(1.,0.,0.));
#5219=DIRECTION('',(0.,0.,-1.));
#5220=DIRECTION('center_axis',(0.,0.,-1.));
#5221=DIRECTION('ref_axis',(0.937993710434555,-0.346652274167091,0.));
#5222=DIRECTION('',(0.,0.,-1.));
#5223=DIRECTION('center_axis',(0.,0.,-1.));
#5224=DIRECTION('ref_axis',(1.,0.,0.));
#5225=DIRECTION('center_axis',(0.,0.,-1.));
#5226=DIRECTION('ref_axis',(-0.346967093288461,0.937877303369133,0.));
#5227=DIRECTION('',(0.,0.,-1.));
#5228=DIRECTION('center_axis',(0.,0.,-1.));
#5229=DIRECTION('ref_axis',(1.,0.,0.));
#5230=DIRECTION('center_axis',(0.,0.,-1.));
#5231=DIRECTION('ref_axis',(1.,0.,0.));
#5232=DIRECTION('',(0.,0.,-1.));
#5233=DIRECTION('center_axis',(0.,0.,-1.));
#5234=DIRECTION('ref_axis',(1.,0.,0.));
#5235=DIRECTION('',(0.,0.,-1.));
#5236=DIRECTION('center_axis',(0.,0.,-1.));
#5237=DIRECTION('ref_axis',(1.,0.,0.));
#5238=DIRECTION('',(0.,0.,-1.));
#5239=DIRECTION('center_axis',(0.,0.,-1.));
#5240=DIRECTION('ref_axis',(1.,0.,0.));
#5241=DIRECTION('',(0.,0.,-1.));
#5242=DIRECTION('center_axis',(0.,0.,-1.));
#5243=DIRECTION('ref_axis',(1.,0.,0.));
#5244=DIRECTION('',(0.,0.,-1.));
#5245=DIRECTION('center_axis',(0.,0.,-1.));
#5246=DIRECTION('ref_axis',(1.,0.,0.));
#5247=DIRECTION('',(0.,0.,-1.));
#5248=DIRECTION('center_axis',(0.,0.,-1.));
#5249=DIRECTION('ref_axis',(1.,0.,0.));
#5250=DIRECTION('',(0.,0.,-1.));
#5251=DIRECTION('center_axis',(0.,0.,-1.));
#5252=DIRECTION('ref_axis',(1.,0.,0.));
#5253=DIRECTION('',(0.,0.,-1.));
#5254=DIRECTION('center_axis',(0.,0.,-1.));
#5255=DIRECTION('ref_axis',(0.937993719003489,-0.346652250980724,0.));
#5256=DIRECTION('',(0.,0.,-1.));
#5257=DIRECTION('center_axis',(0.,0.,-1.));
#5258=DIRECTION('ref_axis',(1.,0.,0.));
#5259=DIRECTION('center_axis',(0.,0.,-1.));
#5260=DIRECTION('ref_axis',(-0.346966676108421,0.93787745770451,0.));
#5261=DIRECTION('',(0.,0.,-1.));
#5262=DIRECTION('center_axis',(0.,0.,-1.));
#5263=DIRECTION('ref_axis',(1.,0.,0.));
#5264=DIRECTION('center_axis',(0.,0.,-1.));
#5265=DIRECTION('ref_axis',(1.,0.,0.));
#5266=DIRECTION('',(0.,0.,-1.));
#5267=DIRECTION('center_axis',(0.,0.,-1.));
#5268=DIRECTION('ref_axis',(1.,0.,0.));
#5269=DIRECTION('',(0.,0.,-1.));
#5270=DIRECTION('center_axis',(0.,0.,-1.));
#5271=DIRECTION('ref_axis',(1.,0.,0.));
#5272=DIRECTION('',(0.,0.,-1.));
#5273=DIRECTION('center_axis',(0.,0.,-1.));
#5274=DIRECTION('ref_axis',(1.,0.,0.));
#5275=DIRECTION('',(0.,0.,-1.));
#5276=DIRECTION('center_axis',(0.,0.,-1.));
#5277=DIRECTION('ref_axis',(1.,0.,0.));
#5278=DIRECTION('',(0.,0.,-1.));
#5279=DIRECTION('center_axis',(0.,0.,-1.));
#5280=DIRECTION('ref_axis',(1.,0.,0.));
#5281=DIRECTION('',(0.,0.,-1.));
#5282=DIRECTION('center_axis',(0.,0.,-1.));
#5283=DIRECTION('ref_axis',(1.,0.,0.));
#5284=DIRECTION('',(0.,0.,-1.));
#5285=DIRECTION('center_axis',(0.,0.,-1.));
#5286=DIRECTION('ref_axis',(1.,0.,0.));
#5287=DIRECTION('',(0.,0.,-1.));
#5288=DIRECTION('center_axis',(0.,0.,-1.));
#5289=DIRECTION('ref_axis',(0.937993675279511,-0.346652369291823,0.));
#5290=DIRECTION('',(0.,0.,-1.));
#5291=DIRECTION('center_axis',(0.,0.,-1.));
#5292=DIRECTION('ref_axis',(1.,0.,0.));
#5293=DIRECTION('center_axis',(0.,0.,-1.));
#5294=DIRECTION('ref_axis',(1.,-4.04571266497536E-14,0.));
#5295=DIRECTION('',(1.22464679914735E-16,-4.9695666632586E-30,-1.));
#5296=DIRECTION('center_axis',(0.,0.,1.));
#5297=DIRECTION('ref_axis',(1.,-4.04571266497536E-14,0.));
#5298=DIRECTION('center_axis',(0.,0.,-1.));
#5299=DIRECTION('ref_axis',(1.,-4.04571266497536E-14,0.));
#5300=DIRECTION('',(1.22464679914735E-16,-4.9695666632586E-30,-1.));
#5301=DIRECTION('center_axis',(0.,0.,-1.));
#5302=DIRECTION('ref_axis',(1.,-4.04571266497536E-14,0.));
#5303=DIRECTION('',(1.22464679914735E-16,-4.9695666632586E-30,-1.));
#5304=DIRECTION('center_axis',(0.,0.,-1.));
#5305=DIRECTION('ref_axis',(1.,-4.04571266497536E-14,0.));
#5306=DIRECTION('',(1.22464679914735E-16,-4.9695666632586E-30,-1.));
#5307=DIRECTION('center_axis',(0.,0.,-1.));
#5308=DIRECTION('ref_axis',(1.,-4.04571266497536E-14,0.));
#5309=DIRECTION('',(1.22464679914735E-16,-4.9695666632586E-30,-1.));
#5310=DIRECTION('center_axis',(0.,0.,-1.));
#5311=DIRECTION('ref_axis',(1.,-4.04571266497536E-14,0.));
#5312=DIRECTION('',(1.22464679914735E-16,-4.9695666632586E-30,-1.));
#5313=DIRECTION('center_axis',(0.,0.,-1.));
#5314=DIRECTION('ref_axis',(1.,-4.04571266497536E-14,0.));
#5315=DIRECTION('',(1.22464679914735E-16,-4.9695666632586E-30,-1.));
#5316=DIRECTION('center_axis',(0.,0.,-1.));
#5317=DIRECTION('ref_axis',(1.,-4.04571266497536E-14,0.));
#5318=DIRECTION('',(1.22464679914735E-16,-4.9695666632586E-30,-1.));
#5319=DIRECTION('center_axis',(0.,0.,-1.));
#5320=DIRECTION('ref_axis',(1.,-4.04571266497536E-14,0.));
#5321=DIRECTION('',(1.22464679914735E-16,-4.9695666632586E-30,-1.));
#5322=DIRECTION('center_axis',(0.,0.,-1.));
#5323=DIRECTION('ref_axis',(-0.609230889865466,-0.792992889522808,0.));
#5324=DIRECTION('',(1.22464679914735E-16,-4.9695666632586E-30,-1.));
#5325=DIRECTION('center_axis',(0.,0.,-1.));
#5326=DIRECTION('ref_axis',(1.,-4.04571266497536E-14,0.));
#5327=DIRECTION('center_axis',(0.,0.,-1.));
#5328=DIRECTION('ref_axis',(1.,-3.75673318890567E-14,0.));
#5329=DIRECTION('',(1.22464679914735E-16,-4.61566887287058E-30,-1.));
#5330=DIRECTION('center_axis',(0.,0.,1.));
#5331=DIRECTION('ref_axis',(1.,-3.75673318890567E-14,0.));
#5332=DIRECTION('center_axis',(0.,0.,-1.));
#5333=DIRECTION('ref_axis',(1.,-3.75673318890567E-14,0.));
#5334=DIRECTION('',(1.22464679914735E-16,-4.61566887287058E-30,-1.));
#5335=DIRECTION('center_axis',(0.,0.,-1.));
#5336=DIRECTION('ref_axis',(1.,-3.75673318890567E-14,0.));
#5337=DIRECTION('',(1.22464679914735E-16,-4.61566887287058E-30,-1.));
#5338=DIRECTION('center_axis',(0.,0.,-1.));
#5339=DIRECTION('ref_axis',(1.,-3.75673318890567E-14,0.));
#5340=DIRECTION('',(1.22464679914735E-16,-4.61566887287058E-30,-1.));
#5341=DIRECTION('center_axis',(0.,0.,-1.));
#5342=DIRECTION('ref_axis',(1.,-3.75673318890567E-14,0.));
#5343=DIRECTION('',(1.22464679914735E-16,-4.61566887287058E-30,-1.));
#5344=DIRECTION('center_axis',(0.,0.,-1.));
#5345=DIRECTION('ref_axis',(1.,-3.75673318890567E-14,0.));
#5346=DIRECTION('',(1.22464679914735E-16,-4.61566887287058E-30,-1.));
#5347=DIRECTION('center_axis',(0.,0.,-1.));
#5348=DIRECTION('ref_axis',(1.,-3.75673318890567E-14,0.));
#5349=DIRECTION('',(1.22464679914735E-16,-4.61566887287058E-30,-1.));
#5350=DIRECTION('center_axis',(0.,0.,-1.));
#5351=DIRECTION('ref_axis',(1.,-3.75673318890567E-14,0.));
#5352=DIRECTION('',(1.22464679914735E-16,-4.61566887287058E-30,-1.));
#5353=DIRECTION('center_axis',(0.,0.,-1.));
#5354=DIRECTION('ref_axis',(1.,-3.75673318890567E-14,0.));
#5355=DIRECTION('',(1.22464679914735E-16,-4.61566887287058E-30,-1.));
#5356=DIRECTION('center_axis',(0.,0.,-1.));
#5357=DIRECTION('ref_axis',(-0.609230947703889,-0.792992845087408,0.));
#5358=DIRECTION('',(1.22464679914735E-16,-4.61566887287058E-30,-1.));
#5359=DIRECTION('center_axis',(0.,0.,-1.));
#5360=DIRECTION('ref_axis',(1.,-3.75673318890567E-14,0.));
#5361=DIRECTION('center_axis',(0.,0.,-1.));
#5362=DIRECTION('ref_axis',(1.,-3.46775371283601E-14,0.));
#5363=DIRECTION('',(1.22464679914735E-16,-4.26177108248259E-30,-1.));
#5364=DIRECTION('center_axis',(0.,0.,1.));
#5365=DIRECTION('ref_axis',(1.,-3.46775371283601E-14,0.));
#5366=DIRECTION('center_axis',(0.,0.,-1.));
#5367=DIRECTION('ref_axis',(1.,-3.46775371283601E-14,0.));
#5368=DIRECTION('',(1.22464679914735E-16,-4.26177108248259E-30,-1.));
#5369=DIRECTION('center_axis',(0.,0.,-1.));
#5370=DIRECTION('ref_axis',(1.,-3.46775371283601E-14,0.));
#5371=DIRECTION('',(1.22464679914735E-16,-4.26177108248259E-30,-1.));
#5372=DIRECTION('center_axis',(0.,0.,-1.));
#5373=DIRECTION('ref_axis',(1.,-3.46775371283601E-14,0.));
#5374=DIRECTION('',(1.22464679914735E-16,-4.26177108248259E-30,-1.));
#5375=DIRECTION('center_axis',(0.,0.,-1.));
#5376=DIRECTION('ref_axis',(1.,-3.46775371283601E-14,0.));
#5377=DIRECTION('',(1.22464679914735E-16,-4.26177108248259E-30,-1.));
#5378=DIRECTION('center_axis',(0.,0.,-1.));
#5379=DIRECTION('ref_axis',(1.,-3.46775371283601E-14,0.));
#5380=DIRECTION('',(1.22464679914735E-16,-4.26177108248259E-30,-1.));
#5381=DIRECTION('center_axis',(0.,0.,-1.));
#5382=DIRECTION('ref_axis',(1.,-3.46775371283601E-14,0.));
#5383=DIRECTION('',(1.22464679914735E-16,-4.26177108248259E-30,-1.));
#5384=DIRECTION('center_axis',(0.,0.,-1.));
#5385=DIRECTION('ref_axis',(1.,-3.46775371283601E-14,0.));
#5386=DIRECTION('',(1.22464679914735E-16,-4.26177108248259E-30,-1.));
#5387=DIRECTION('center_axis',(0.,0.,-1.));
#5388=DIRECTION('ref_axis',(1.,-3.46775371283601E-14,0.));
#5389=DIRECTION('',(1.22464679914735E-16,-4.26177108248259E-30,-1.));
#5390=DIRECTION('center_axis',(0.,0.,-1.));
#5391=DIRECTION('ref_axis',(-0.609230907205664,-0.792992876200892,0.));
#5392=DIRECTION('',(1.22464679914735E-16,-4.26177108248259E-30,-1.));
#5393=DIRECTION('center_axis',(0.,0.,-1.));
#5394=DIRECTION('ref_axis',(1.,-3.46775371283601E-14,0.));
#5395=DIRECTION('center_axis',(0.,0.,-1.));
#5396=DIRECTION('ref_axis',(1.,-3.17877423676634E-14,0.));
#5397=DIRECTION('',(1.22464679914735E-16,-3.90787329209458E-30,-1.));
#5398=DIRECTION('center_axis',(0.,0.,1.));
#5399=DIRECTION('ref_axis',(1.,-3.17877423676634E-14,0.));
#5400=DIRECTION('center_axis',(0.,0.,-1.));
#5401=DIRECTION('ref_axis',(1.,-3.17877423676634E-14,0.));
#5402=DIRECTION('',(1.22464679914735E-16,-3.90787329209458E-30,-1.));
#5403=DIRECTION('center_axis',(0.,0.,-1.));
#5404=DIRECTION('ref_axis',(1.,-3.17877423676634E-14,0.));
#5405=DIRECTION('',(1.22464679914735E-16,-3.90787329209458E-30,-1.));
#5406=DIRECTION('center_axis',(0.,0.,-1.));
#5407=DIRECTION('ref_axis',(1.,-3.17877423676634E-14,0.));
#5408=DIRECTION('',(1.22464679914735E-16,-3.90787329209458E-30,-1.));
#5409=DIRECTION('center_axis',(0.,0.,-1.));
#5410=DIRECTION('ref_axis',(1.,-3.17877423676634E-14,0.));
#5411=DIRECTION('',(1.22464679914735E-16,-3.90787329209458E-30,-1.));
#5412=DIRECTION('center_axis',(0.,0.,-1.));
#5413=DIRECTION('ref_axis',(1.,-3.17877423676634E-14,0.));
#5414=DIRECTION('',(1.22464679914735E-16,-3.90787329209458E-30,-1.));
#5415=DIRECTION('center_axis',(0.,0.,-1.));
#5416=DIRECTION('ref_axis',(1.,-3.17877423676634E-14,0.));
#5417=DIRECTION('',(1.22464679914735E-16,-3.90787329209458E-30,-1.));
#5418=DIRECTION('center_axis',(0.,0.,-1.));
#5419=DIRECTION('ref_axis',(1.,-3.17877423676634E-14,0.));
#5420=DIRECTION('',(1.22464679914735E-16,-3.90787329209458E-30,-1.));
#5421=DIRECTION('center_axis',(0.,0.,-1.));
#5422=DIRECTION('ref_axis',(1.,-3.17877423676634E-14,0.));
#5423=DIRECTION('',(1.22464679914735E-16,-3.90787329209458E-30,-1.));
#5424=DIRECTION('center_axis',(0.,0.,-1.));
#5425=DIRECTION('ref_axis',(-0.609230926478059,-0.792992861394531,0.));
#5426=DIRECTION('',(1.22464679914735E-16,-3.90787329209458E-30,-1.));
#5427=DIRECTION('center_axis',(0.,0.,-1.));
#5428=DIRECTION('ref_axis',(1.,-3.17877423676634E-14,0.));
#5429=DIRECTION('center_axis',(0.,0.,-1.));
#5430=DIRECTION('ref_axis',(1.,-3.17877423676634E-14,0.));
#5431=DIRECTION('center_axis',(0.,0.,1.));
#5432=DIRECTION('ref_axis',(1.,0.,0.));
#5433=DIRECTION('',(0.,-1.,0.));
#5434=DIRECTION('',(1.,0.,0.));
#5435=DIRECTION('',(0.,1.,0.));
#5436=DIRECTION('',(-1.,0.,0.));
#5437=DIRECTION('center_axis',(0.,0.,-1.));
#5438=DIRECTION('ref_axis',(1.,-3.46775371283601E-14,0.));
#5439=DIRECTION('center_axis',(0.,0.,-1.));
#5440=DIRECTION('ref_axis',(1.,-3.75673318890567E-14,0.));
#5441=DIRECTION('center_axis',(0.,0.,-1.));
#5442=DIRECTION('ref_axis',(1.,-4.04571266497536E-14,0.));
#5443=DIRECTION('center_axis',(0.,0.,-1.));
#5444=DIRECTION('ref_axis',(1.,0.,0.));
#5445=DIRECTION('center_axis',(0.,0.,-1.));
#5446=DIRECTION('ref_axis',(1.,0.,0.));
#5447=DIRECTION('center_axis',(0.,0.,-1.));
#5448=DIRECTION('ref_axis',(1.,0.,0.));
#5449=DIRECTION('center_axis',(0.,0.,-1.));
#5450=DIRECTION('ref_axis',(1.,0.,0.));
#5451=DIRECTION('center_axis',(0.,1.,0.));
#5452=DIRECTION('ref_axis',(-1.,0.,0.));
#5453=DIRECTION('',(-1.,0.,0.));
#5454=DIRECTION('',(0.,0.,1.));
#5455=DIRECTION('',(0.,0.,1.));
#5456=DIRECTION('center_axis',(1.,0.,0.));
#5457=DIRECTION('ref_axis',(0.,1.,0.));
#5458=DIRECTION('',(0.,1.,0.));
#5459=DIRECTION('',(0.,0.,1.));
#5460=DIRECTION('center_axis',(0.,-1.,0.));
#5461=DIRECTION('ref_axis',(1.,0.,0.));
#5462=DIRECTION('',(1.,0.,0.));
#5463=DIRECTION('',(0.,0.,1.));
#5464=DIRECTION('center_axis',(-1.,0.,0.));
#5465=DIRECTION('ref_axis',(0.,-1.,0.));
#5466=DIRECTION('',(0.,-1.,0.));
#5467=DIRECTION('center_axis',(0.,0.,1.));
#5468=DIRECTION('ref_axis',(1.,0.,0.));
#6185=CARTESIAN_POINT('',(0.,0.,0.));
#6186=CARTESIAN_POINT('Origin',(40.,30.,5.));
#6187=CARTESIAN_POINT('',(37.4865492426837,30.0006055736961,0.387416697508023));
#6188=CARTESIAN_POINT('',(37.4843813836159,29.9964988963182,0.112583302491979));
#6189=CARTESIAN_POINT('',(37.4825,30.,5.));
#6190=CARTESIAN_POINT('',(38.086534003335,31.635987203375,0.));
#6191=CARTESIAN_POINT('Ctrl Pts',(37.4843813836159,29.9964988963182,0.112583302491979));
#6192=CARTESIAN_POINT('Ctrl Pts',(37.4896308378643,30.5890976659027,0.0750555349946511));
#6193=CARTESIAN_POINT('Ctrl Pts',(37.700778171916,31.1848035603044,0.0375277674973235));
#6194=CARTESIAN_POINT('Ctrl Pts',(38.086534003335,31.635987203375,-4.44089209850063E-15));
#6195=CARTESIAN_POINT('',(41.9171065683076,31.6387569269747,-6.03363952037314E-16));
#6196=CARTESIAN_POINT('Origin',(40.,30.,0.));
#6197=CARTESIAN_POINT('Ctrl Pts',(41.9171095224698,31.6387591744824,-4.02677955152094E-16));
#6198=CARTESIAN_POINT('Ctrl Pts',(41.3863013821206,32.2578627143831,0.0517824693358733));
#6199=CARTESIAN_POINT('Ctrl Pts',(40.5267002275034,32.5973566946348,0.103564938671747));
#6200=CARTESIAN_POINT('Ctrl Pts',(39.7163628727442,32.5055173392451,0.15534740800762));
#6201=CARTESIAN_POINT('Ctrl Pts',(38.8880955008986,32.4116458904295,0.208275647749515));
#6202=CARTESIAN_POINT('Ctrl Pts',(38.1112961294035,31.867142043505,0.26120388749141));
#6203=CARTESIAN_POINT('Ctrl Pts',(37.7410321515366,31.1206209684195,0.314132127233305));
#6204=CARTESIAN_POINT('Ctrl Pts',(37.5701426815768,30.7760759992598,0.338560317324878));
#6205=CARTESIAN_POINT('Ctrl Pts',(37.485850848764,30.3884985785696,0.36298850741645));
#6206=CARTESIAN_POINT('Ctrl Pts',(37.4865492426837,30.0006055736961,0.387416697508023));
#6207=CARTESIAN_POINT('Origin',(40.,30.,5.));
#6208=CARTESIAN_POINT('',(37.4826513052474,29.9976965354932,1.38741669750802));
#6209=CARTESIAN_POINT('',(37.4783311322817,30.0001213195654,1.11258330249198));
#6210=CARTESIAN_POINT('',(37.4825,30.,5.));
#6211=CARTESIAN_POINT('Ctrl Pts',(37.4783311322817,30.0001213195654,1.11258330249198));
#6212=CARTESIAN_POINT('Ctrl Pts',(37.4783275808006,30.0058437240052,1.11221987985458));
#6213=CARTESIAN_POINT('Ctrl Pts',(37.4783453684107,30.0115661037913,1.11185645721718));
#6214=CARTESIAN_POINT('Ctrl Pts',(37.4783845615425,30.0172883349493,1.11149303457978));
#6215=CARTESIAN_POINT('Ctrl Pts',(37.4840925809837,30.8506641113011,1.05856479483789));
#6216=CARTESIAN_POINT('Ctrl Pts',(37.9438224654611,31.6808874105992,1.00563655509599));
#6217=CARTESIAN_POINT('Ctrl Pts',(38.6471444516464,32.1280310844825,0.952708315354099));
#6218=CARTESIAN_POINT('Ctrl Pts',(39.3504664378318,32.5751747583658,0.899780075612205));
#6219=CARTESIAN_POINT('Ctrl Pts',(40.2973805257251,32.6392388068343,0.84685183587031));
#6220=CARTESIAN_POINT('Ctrl Pts',(41.0544290556679,32.2906973355318,0.793923596128415));
#6221=CARTESIAN_POINT('Ctrl Pts',(41.8114775856107,31.9421558642292,0.740995356386521));
#6222=CARTESIAN_POINT('Ctrl Pts',(42.378660557603,31.1810088731556,0.688067116644628));
#6223=CARTESIAN_POINT('Ctrl Pts',(42.496385640448,30.3560668613964,0.635138876902733));
#6224=CARTESIAN_POINT('Ctrl Pts',(42.6141107232931,29.5311248496373,0.582210637160839));
#6225=CARTESIAN_POINT('Ctrl Pts',(42.282377916991,28.6423878171925,0.529282397418944));
#6226=CARTESIAN_POINT('Ctrl Pts',(41.6529742937847,28.0958630035297,0.47635415767705));
#6227=CARTESIAN_POINT('Ctrl Pts',(41.0235706705784,27.5493381898668,0.423425917935155));
#6228=CARTESIAN_POINT('Ctrl Pts',(40.0964962304679,27.3450255949858,0.370497678193261));
#6229=CARTESIAN_POINT('Ctrl Pts',(39.2962221198814,27.5780866114451,0.317569438451365));
#6230=CARTESIAN_POINT('Ctrl Pts',(38.495948009295,27.8111476279043,0.264641198709472));
#6231=CARTESIAN_POINT('Ctrl Pts',(37.8224742282327,28.4815822557037,0.211712958967577));
#6232=CARTESIAN_POINT('Ctrl Pts',(37.5841055938905,29.2787075728659,0.158784719225683));
#6233=CARTESIAN_POINT('Ctrl Pts',(37.5147477320938,29.5106462578148,0.143384246981115));
#6234=CARTESIAN_POINT('Ctrl Pts',(37.4822271367784,29.7533109447887,0.127983774736547));
#6235=CARTESIAN_POINT('Ctrl Pts',(37.4843813836159,29.9964988963182,0.112583302491979));
#6236=CARTESIAN_POINT('Ctrl Pts',(37.4865492426837,30.0006055736961,0.387416697508023));
#6237=CARTESIAN_POINT('Ctrl Pts',(37.4873640497288,29.548055881866,0.415916747158346));
#6238=CARTESIAN_POINT('Ctrl Pts',(37.6038640135046,29.0950766299899,0.444416796808668));
#6239=CARTESIAN_POINT('Ctrl Pts',(37.8334964929258,28.7095041526117,0.472916846458991));
#6240=CARTESIAN_POINT('Ctrl Pts',(38.2599533964209,27.9934467151356,0.525845086200884));
#6241=CARTESIAN_POINT('Ctrl Pts',(39.0765957876499,27.5098701434296,0.578773325942778));
#6242=CARTESIAN_POINT('Ctrl Pts',(39.9094857112398,27.479971270026,0.631701565684672));
#6243=CARTESIAN_POINT('Ctrl Pts',(40.7423756348297,27.4500723966223,0.684629805426567));
#6244=CARTESIAN_POINT('Ctrl Pts',(41.5915130907804,27.8738512215209,0.737558045168462));
#6245=CARTESIAN_POINT('Ctrl Pts',(42.0682758200043,28.5574047494562,0.790486284910356));
#6246=CARTESIAN_POINT('Ctrl Pts',(42.5450385492282,29.2409582773914,0.843414524652251));
#6247=CARTESIAN_POINT('Ctrl Pts',(42.6494265517252,30.1842865083634,0.896342764394145));
#6248=CARTESIAN_POINT('Ctrl Pts',(42.333625344339,30.9555495584931,0.949271004136039));
#6249=CARTESIAN_POINT('Ctrl Pts',(42.0178241369527,31.7268126086228,1.00219924387793));
#6250=CARTESIAN_POINT('Ctrl Pts',(41.2818337196832,32.3260104779102,1.05512748361983));
#6251=CARTESIAN_POINT('Ctrl Pts',(40.4625635148939,32.4788849033583,1.10805572336172));
#6252=CARTESIAN_POINT('Ctrl Pts',(39.6432933101047,32.6317593288063,1.16098396310362));
#6253=CARTESIAN_POINT('Ctrl Pts',(38.7407433177957,32.3383103104151,1.21391220284551));
#6254=CARTESIAN_POINT('Ctrl Pts',(38.1680403886987,31.7328518944262,1.26684044258741));
#6255=CARTESIAN_POINT('Ctrl Pts',(37.733147316435,31.273085308157,1.30703252756095));
#6256=CARTESIAN_POINT('Ctrl Pts',(37.488457870222,30.6334010406233,1.34722461253449));
#6257=CARTESIAN_POINT('Ctrl Pts',(37.4826513052474,29.9976965354932,1.38741669750802));
#6258=CARTESIAN_POINT('Origin',(40.,30.,5.));
#6259=CARTESIAN_POINT('',(37.4786864827572,30.000865351545,2.38741669750803));
#6260=CARTESIAN_POINT('',(37.4841918288605,30.0021290961335,2.11258330249198));
#6261=CARTESIAN_POINT('',(37.4825,30.,5.));
#6262=CARTESIAN_POINT('Ctrl Pts',(37.4841918288605,30.0021290961335,2.11258330249198));
#6263=CARTESIAN_POINT('Ctrl Pts',(37.4821415438194,30.257605834553,2.09645598497262));
#6264=CARTESIAN_POINT('Ctrl Pts',(37.517933068672,30.5125215673247,2.08032866745325));
#6265=CARTESIAN_POINT('Ctrl Pts',(37.5939458442133,30.7548191659607,2.06420134993388));
#6266=CARTESIAN_POINT('Ctrl Pts',(37.8434121551767,31.5500156004633,2.01127311019199));
#6267=CARTESIAN_POINT('Ctrl Pts',(38.5260961730752,32.2093038013217,1.9583448704501));
#6268=CARTESIAN_POINT('Ctrl Pts',(39.3295050503994,32.4309016291222,1.9054166307082));
#6269=CARTESIAN_POINT('Ctrl Pts',(40.1329139277237,32.6524994569227,1.85248839096631));
#6270=CARTESIAN_POINT('Ctrl Pts',(41.0570476644737,32.4364069116652,1.79956015122441));
#6271=CARTESIAN_POINT('Ctrl Pts',(41.6788914300393,31.8815353981424,1.74663191148252));
#6272=CARTESIAN_POINT('Ctrl Pts',(42.300735195605,31.3266638846196,1.69370367174062));
#6273=CARTESIAN_POINT('Ctrl Pts',(42.6202889899864,30.4330134028314,1.64077543199873));
#6274=CARTESIAN_POINT('Ctrl Pts',(42.4912801935499,29.6096514151861,1.58784719225683));
#6275=CARTESIAN_POINT('Ctrl Pts',(42.3622713971135,28.7862894275408,1.53491895251494));
#6276=CARTESIAN_POINT('Ctrl Pts',(41.7847000098592,28.0332159340385,1.48199071277304));
#6277=CARTESIAN_POINT('Ctrl Pts',(41.0229435846798,27.6951314558291,1.42906247303115));
#6278=CARTESIAN_POINT('Ctrl Pts',(40.2611871595004,27.3570469776196,1.37613423328926));
#6279=CARTESIAN_POINT('Ctrl Pts',(39.315245696396,27.4339515147031,1.32320599354736));
#6280=CARTESIAN_POINT('Ctrl Pts',(38.6181180420463,27.8906679099476,1.27027775380547));
#6281=CARTESIAN_POINT('Ctrl Pts',(37.9257770946035,28.3442483407671,1.21771293670097));
#6282=CARTESIAN_POINT('Ctrl Pts',(37.478844812322,29.1724427111836,1.16514811959648));
#6283=CARTESIAN_POINT('Ctrl Pts',(37.4783311322817,30.0001213195654,1.11258330249198));
#6284=CARTESIAN_POINT('Ctrl Pts',(37.4826513052474,29.9976965354932,1.38741669750802));
#6285=CARTESIAN_POINT('Ctrl Pts',(37.4808113083864,29.7962531177255,1.40015285227638));
#6286=CARTESIAN_POINT('Ctrl Pts',(37.502958569874,29.5952093250312,1.41288900704473));
#6287=CARTESIAN_POINT('Ctrl Pts',(37.5506420393601,29.4004166824566,1.42562516181309));
#6288=CARTESIAN_POINT('Ctrl Pts',(37.7488024850036,28.5909077000624,1.47855340155498));
#6289=CARTESIAN_POINT('Ctrl Pts',(38.3879792421759,27.8893575488604,1.53148164129688));
#6290=CARTESIAN_POINT('Ctrl Pts',(39.1755924364077,27.6168925555489,1.58440988103877));
#6291=CARTESIAN_POINT('Ctrl Pts',(39.9632056306395,27.3444275622373,1.63733812078067));
#6292=CARTESIAN_POINT('Ctrl Pts',(40.8992552619309,27.5010477268163,1.69026636052256));
#6293=CARTESIAN_POINT('Ctrl Pts',(41.5552733407625,28.0150626943082,1.74319460026446));
#6294=CARTESIAN_POINT('Ctrl Pts',(42.2112914195941,28.5290776618002,1.79612284000635));
#6295=CARTESIAN_POINT('Ctrl Pts',(42.5872779459659,29.4004874322051,1.84905107974825));
#6296=CARTESIAN_POINT('Ctrl Pts',(42.5111276934142,30.2304107639936,1.90197931949014));
#6297=CARTESIAN_POINT('Ctrl Pts',(42.4349774408626,31.060334095782,1.95490755923204));
#6298=CARTESIAN_POINT('Ctrl Pts',(41.9066904093874,31.848770988954,2.00783579897393));
#6299=CARTESIAN_POINT('Ctrl Pts',(41.1680858742699,32.23482127651,2.06076403871582));
#6300=CARTESIAN_POINT('Ctrl Pts',(40.4294813391524,32.6208715640661,2.11369227845772));
#6301=CARTESIAN_POINT('Ctrl Pts',(39.4805593003925,32.6045352460063,2.16662051819961));
#6302=CARTESIAN_POINT('Ctrl Pts',(38.7556808583415,32.1932899824628,2.21954875794151));
#6303=CARTESIAN_POINT('Ctrl Pts',(38.0308024162905,31.7820447189193,2.2724769976834));
#6304=CARTESIAN_POINT('Ctrl Pts',(37.5299675709483,30.9758905098923,2.3254052374253));
#6305=CARTESIAN_POINT('Ctrl Pts',(37.482429398745,30.1438378634159,2.37833347716719));
#6306=CARTESIAN_POINT('Ctrl Pts',(37.4797099954244,30.0962406036797,2.3813612172808));
#6307=CARTESIAN_POINT('Ctrl Pts',(37.4784739461469,30.0485585946962,2.38438895739441));
#6308=CARTESIAN_POINT('Ctrl Pts',(37.4786864827572,30.000865351545,2.38741669750803));
#6309=CARTESIAN_POINT('Origin',(40.,30.,5.));
#6310=CARTESIAN_POINT('',(37.4852129709663,30.0017637215755,3.38741669750803));
#6311=CARTESIAN_POINT('',(37.485883012183,29.9986698324052,3.11258330249198));
#6312=CARTESIAN_POINT('',(37.4825,30.,5.));
#6313=CARTESIAN_POINT('Ctrl Pts',(37.485883012183,29.9986698324052,3.11258330249198));
#6314=CARTESIAN_POINT('Ctrl Pts',(37.4883076973175,30.504721507644,3.08069209009065));
#6315=CARTESIAN_POINT('Ctrl Pts',(37.636377858221,31.0120786438038,3.04880087768932));
#6316=CARTESIAN_POINT('Ctrl Pts',(37.920388915981,31.4262068815774,3.01690966528799));
#6317=CARTESIAN_POINT('Ctrl Pts',(38.3917477707431,32.1135146695953,2.96398142554609));
#6318=CARTESIAN_POINT('Ctrl Pts',(39.2375472597066,32.5440293317411,2.9110531858042));
#6319=CARTESIAN_POINT('Ctrl Pts',(40.0706296546987,32.5206863623676,2.8581249460623));
#6320=CARTESIAN_POINT('Ctrl Pts',(40.9037120496908,32.497343392994,2.80519670632041));
#6321=CARTESIAN_POINT('Ctrl Pts',(41.7240773507114,32.0201427921011,2.75226846657851));
#6322=CARTESIAN_POINT('Ctrl Pts',(42.1562101132269,31.3075191431985,2.69934022683662));
#6323=CARTESIAN_POINT('Ctrl Pts',(42.5883428757425,30.594895494296,2.64641198709473));
#6324=CARTESIAN_POINT('Ctrl Pts',(42.6322430997529,29.6468487973838,2.59348374735283));
#6325=CARTESIAN_POINT('Ctrl Pts',(42.2678158280527,28.8973396974625,2.54055550761094));
#6326=CARTESIAN_POINT('Ctrl Pts',(41.9033885563526,28.1478305975413,2.48762726786904));
#6327=CARTESIAN_POINT('Ctrl Pts',(41.1306337889419,27.5968590946111,2.43469902812715));
#6328=CARTESIAN_POINT('Ctrl Pts',(40.3032736225135,27.4966276437265,2.38177078838525));
#6329=CARTESIAN_POINT('Ctrl Pts',(39.4759134560852,27.3963961928419,2.32884254864336));
#6330=CARTESIAN_POINT('Ctrl Pts',(38.5939478906392,27.746904794003,2.27591430890146));
#6331=CARTESIAN_POINT('Ctrl Pts',(38.0610894099303,28.387711428657,2.22298606915957));
#6332=CARTESIAN_POINT('Ctrl Pts',(37.6905937425927,28.8332632784178,2.18618514693704));
#6333=CARTESIAN_POINT('Ctrl Pts',(37.4888703738348,29.419156784157,2.14938422471451));
#6334=CARTESIAN_POINT('Ctrl Pts',(37.4841918288605,30.0021290961335,2.11258330249198));
#6335=CARTESIAN_POINT('Ctrl Pts',(37.4786864827572,30.000865351545,2.38741669750803));
#6336=CARTESIAN_POINT('Ctrl Pts',(37.4821893207308,29.2148280521618,2.43731719713631));
#6337=CARTESIAN_POINT('Ctrl Pts',(37.8791668909914,28.4257392519124,2.48721769676459));
#6338=CARTESIAN_POINT('Ctrl Pts',(38.5139722677769,27.9627045952532,2.53711819639288));
#6339=CARTESIAN_POINT('Ctrl Pts',(39.1872948080768,27.4715750574926,2.59004643613477));
#6340=CARTESIAN_POINT('Ctrl Pts',(40.128181387741,27.347267065897,2.64297467587667));
#6341=CARTESIAN_POINT('Ctrl Pts',(40.9059489619732,27.6466815962724,2.69590291561856));
#6342=CARTESIAN_POINT('Ctrl Pts',(41.6837165362054,27.9460961266478,2.74883115536045));
#6343=CARTESIAN_POINT('Ctrl Pts',(42.2983651050056,28.669233178994,2.80175939510235));
#6344=CARTESIAN_POINT('Ctrl Pts',(42.4685443548906,29.4850827307125,2.85468763484424));
#6345=CARTESIAN_POINT('Ctrl Pts',(42.6387236047757,30.300932282431,2.90761587458614));
#6346=CARTESIAN_POINT('Ctrl Pts',(42.3644335357456,31.2094943335216,2.96054411432803));
#6347=CARTESIAN_POINT('Ctrl Pts',(41.7712281653103,31.7948821143088,3.01347235406993));
#6348=CARTESIAN_POINT('Ctrl Pts',(41.1780227948749,32.3802698950961,3.06640059381182));
#6349=CARTESIAN_POINT('Ctrl Pts',(40.2659021230343,32.6424834055799,3.11932883355372));
#6350=CARTESIAN_POINT('Ctrl Pts',(39.4523818516077,32.4614965746811,3.17225707329561));
#6351=CARTESIAN_POINT('Ctrl Pts',(38.6388615801811,32.2805097437823,3.22518531303751));
#6352=CARTESIAN_POINT('Ctrl Pts',(37.9239417091685,31.6563225715008,3.2781135527794));
#6353=CARTESIAN_POINT('Ctrl Pts',(37.6348709055651,30.8746515816341,3.33104179252129));
#6354=CARTESIAN_POINT('Ctrl Pts',(37.5322392470085,30.597127220351,3.34983342751687));
#6355=CARTESIAN_POINT('Ctrl Pts',(37.4832872705902,30.299751503466,3.36862506251245));
#6356=CARTESIAN_POINT('Ctrl Pts',(37.4852129709663,30.0017637215755,3.38741669750803));
#6357=CARTESIAN_POINT('Origin',(40.,30.,5.));
#6358=CARTESIAN_POINT('',(37.4850671861185,29.9981671622093,4.38741669750803));
#6359=CARTESIAN_POINT('',(37.4793386265487,29.9985765177349,4.11258330249198));
#6360=CARTESIAN_POINT('',(37.4825,30.,5.));
#6361=CARTESIAN_POINT('Ctrl Pts',(37.4793386265487,29.9985765177349,4.11258330249198));
#6362=CARTESIAN_POINT('Ctrl Pts',(37.4844207242438,30.7497576670511,4.06492819520868));
#6363=CARTESIAN_POINT('Ctrl Pts',(37.8421139480676,31.5051391927042,4.01727308792539));
#6364=CARTESIAN_POINT('Ctrl Pts',(38.4291013453193,31.9725936575687,3.96961798064209));
#6365=CARTESIAN_POINT('Ctrl Pts',(39.0810400662316,32.4917728892444,3.91668974090019));
#6366=CARTESIAN_POINT('Ctrl Pts',(40.0158241202065,32.6557803161201,3.8637615011583));
#6367=CARTESIAN_POINT('Ctrl Pts',(40.8055638275036,32.3895428935737,3.8108332614164));
#6368=CARTESIAN_POINT('Ctrl Pts',(41.5953035348006,32.1233054710273,3.75790502167451));
#6369=CARTESIAN_POINT('Ctrl Pts',(42.2399988954197,31.4268231990587,3.70497678193261));
#6370=CARTESIAN_POINT('Ctrl Pts',(42.4445459328977,30.6189050842116,3.65204854219072));
#6371=CARTESIAN_POINT('Ctrl Pts',(42.6490929703756,29.8109869693645,3.59912030244883));
#6372=CARTESIAN_POINT('Ctrl Pts',(42.4134916847125,28.8916330116387,3.54619206270693));
#6373=CARTESIAN_POINT('Ctrl Pts',(41.8455866185718,28.2816698932712,3.49326382296504));
#6374=CARTESIAN_POINT('Ctrl Pts',(41.2776815524311,27.6717067749037,3.44033558322314));
#6375=CARTESIAN_POINT('Ctrl Pts',(40.377472705813,27.3711344958944,3.38740734348125));
#6376=CARTESIAN_POINT('Ctrl Pts',(39.5570232426543,27.5175375312054,3.33447910373935));
#6377=CARTESIAN_POINT('Ctrl Pts',(38.7365737794957,27.6639405665165,3.28155086399746));
#6378=CARTESIAN_POINT('Ctrl Pts',(37.9958836997965,28.2573189161479,3.22862262425556));
#6379=CARTESIAN_POINT('Ctrl Pts',(37.6739977702273,29.0260585479087,3.17569438451367));
#6380=CARTESIAN_POINT('Ctrl Pts',(37.5460599598276,29.3316042590449,3.15465735717311));
#6381=CARTESIAN_POINT('Ctrl Pts',(37.4842835694643,29.6648530181128,3.13362032983254));
#6382=CARTESIAN_POINT('Ctrl Pts',(37.485883012183,29.9986698324052,3.11258330249198));
#6383=CARTESIAN_POINT('Ctrl Pts',(37.4852129709663,30.0017637215755,3.38741669750803));
#6384=CARTESIAN_POINT('Ctrl Pts',(37.4887111696391,29.4604435473585,3.42155330225434));
#6385=CARTESIAN_POINT('Ctrl Pts',(37.6601047626962,28.9171035699204,3.45568990700066));
#6386=CARTESIAN_POINT('Ctrl Pts',(37.9825965759643,28.4870775147433,3.48982651174698));
#6387=CARTESIAN_POINT('Ctrl Pts',(38.4826147861612,27.8203292451712,3.54275475148887));
#6388=CARTESIAN_POINT('Ctrl Pts',(39.3458729427491,27.4259875134789,3.59568299123076));
#6389=CARTESIAN_POINT('Ctrl Pts',(40.1772217549583,27.4845589905516,3.64861123097266));
#6390=CARTESIAN_POINT('Ctrl Pts',(41.0085705671675,27.5431304676243,3.70153947071455));
#6391=CARTESIAN_POINT('Ctrl Pts',(41.8080100349979,28.0546151534619,3.75446771045645));
#6392=CARTESIAN_POINT('Ctrl Pts',(42.209603344971,28.7848851576249,3.80739595019834));
#6393=CARTESIAN_POINT('Ctrl Pts',(42.6111966549441,29.5151551617878,3.86032418994024));
#6394=CARTESIAN_POINT('Ctrl Pts',(42.6149438070599,30.464210484276,3.91325242968213));
#6395=CARTESIAN_POINT('Ctrl Pts',(42.2191295734494,31.1976288901078,3.96618066942403));
#6396=CARTESIAN_POINT('Ctrl Pts',(41.8233153398388,31.9310472959396,4.01910890916592));
#6397=CARTESIAN_POINT('Ctrl Pts',(41.0279397205019,32.448828785115,4.07203714890782));
#6398=CARTESIAN_POINT('Ctrl Pts',(40.1970793356802,32.5139631575899,4.12496538864971));
#6399=CARTESIAN_POINT('Ctrl Pts',(39.3662189508584,32.5790975300648,4.17789362839161));
#6400=CARTESIAN_POINT('Ctrl Pts',(38.4998738005519,32.1915847858392,4.2308218681335));
#6401=CARTESIAN_POINT('Ctrl Pts',(37.9946062216704,31.5288056829042,4.28375010787539));
#6402=CARTESIAN_POINT('Ctrl Pts',(37.6647295999779,31.0960937090058,4.31830563775294));
#6403=CARTESIAN_POINT('Ctrl Pts',(37.4887608118784,30.5460505789162,4.35286116763048));
#6404=CARTESIAN_POINT('Ctrl Pts',(37.4850671861185,29.9981671622093,4.38741669750803));
#6405=CARTESIAN_POINT('Origin',(40.,30.,5.));
#6406=CARTESIAN_POINT('',(37.4785970161092,29.9992487947885,5.38741669750803));
#6407=CARTESIAN_POINT('',(37.4815746018733,30.0022201830298,5.11258330249198));
#6408=CARTESIAN_POINT('',(37.4825,30.,5.));
#6409=CARTESIAN_POINT('Ctrl Pts',(37.4815746018733,30.0022201830298,5.11258330249198));
#6410=CARTESIAN_POINT('Ctrl Pts',(37.4800512156624,30.1679668107362,5.10209254006861));
#6411=CARTESIAN_POINT('Ctrl Pts',(37.4950143152585,30.3334397255082,5.09160177764524));
#6412=CARTESIAN_POINT('Ctrl Pts',(37.5274671055976,30.4954083235571,5.08111101522187));
#6413=CARTESIAN_POINT('Ctrl Pts',(37.6911986818205,31.3125760795527,5.02818277547997));
#6414=CARTESIAN_POINT('Ctrl Pts',(38.3001177231744,32.0405439805073,4.97525453573808));
#6415=CARTESIAN_POINT('Ctrl Pts',(39.0754965679032,32.3460907324736,4.92232629599619));
#6416=CARTESIAN_POINT('Ctrl Pts',(39.8508754126321,32.65163748444,4.8693980562543));
#6417=CARTESIAN_POINT('Ctrl Pts',(40.7927140607359,32.5347630874181,4.8164698165124));
#6418=CARTESIAN_POINT('Ctrl Pts',(41.4698936502493,32.0489658313164,4.7635415767705));
#6419=CARTESIAN_POINT('Ctrl Pts',(42.1470732397627,31.5631685752146,4.71061333702861));
#6420=CARTESIAN_POINT('Ctrl Pts',(42.5595937706857,30.7084484600331,4.65768509728672));
#6421=CARTESIAN_POINT('Ctrl Pts',(42.5186273772392,29.8760465588431,4.60475685754482));
#6422=CARTESIAN_POINT('Ctrl Pts',(42.4776609837926,29.0436446576532,4.55182861780293));
#6423=CARTESIAN_POINT('Ctrl Pts',(41.9832076659765,28.2335609704548,4.49890037806103));
#6424=CARTESIAN_POINT('Ctrl Pts',(41.2615993460398,27.8166046141265,4.44597213831914));
#6425=CARTESIAN_POINT('Ctrl Pts',(40.5399910261032,27.3996482577982,4.39304389857724));
#6426=CARTESIAN_POINT('Ctrl Pts',(39.591227704046,27.3758192323399,4.34011565883535));
#6427=CARTESIAN_POINT('Ctrl Pts',(38.8495979541372,27.7560250772875,4.28718741909346));
#6428=CARTESIAN_POINT('Ctrl Pts',(38.1079682042285,28.136230922235,4.23425917935156));
#6429=CARTESIAN_POINT('Ctrl Pts',(37.5734720264681,28.9204716375883,4.18133093960966));
#6430=CARTESIAN_POINT('Ctrl Pts',(37.4907706315128,29.7497675135028,4.12840269986777));
#6431=CARTESIAN_POINT('Ctrl Pts',(37.48253126039,29.8323885683951,4.12312956740917));
#6432=CARTESIAN_POINT('Ctrl Pts',(37.478776282325,29.9154568286489,4.11785643495058));
#6433=CARTESIAN_POINT('Ctrl Pts',(37.4793386265487,29.9985765177349,4.11258330249198));
#6434=CARTESIAN_POINT('Ctrl Pts',(37.4850671861185,29.9981671622093,4.38741669750803));
#6435=CARTESIAN_POINT('Ctrl Pts',(37.4831033350453,29.7068649280859,4.40578940737238));
#6436=CARTESIAN_POINT('Ctrl Pts',(37.5298400476381,29.4161732245676,4.42416211723673));
#6437=CARTESIAN_POINT('Ctrl Pts',(37.6280379842563,29.1440518601549,4.44253482710108));
#6438=CARTESIAN_POINT('Ctrl Pts',(37.9109273331798,28.3601226019852,4.49546306684297));
#6439=CARTESIAN_POINT('Ctrl Pts',(38.620896038483,27.7303095472902,4.54839130658487));
#6440=CARTESIAN_POINT('Ctrl Pts',(39.4329617893699,27.5429044198622,4.60131954632676));
#6441=CARTESIAN_POINT('Ctrl Pts',(40.2450275402567,27.3554992924343,4.65424778606866));
#6442=CARTESIAN_POINT('Ctrl Pts',(41.1591903367271,27.6105020922735,4.70717602581055));
#6443=CARTESIAN_POINT('Ctrl Pts',(41.7569997093075,28.1911873939695,4.76010426555245));
#6444=CARTESIAN_POINT('Ctrl Pts',(42.354809081888,28.7718726956655,4.81303250529434));
#6445=CARTESIAN_POINT('Ctrl Pts',(42.6362650305784,29.6782404992184,4.86596074503623));
#6446=CARTESIAN_POINT('Ctrl Pts',(42.4725334195783,30.4954084287838,4.91888898477813));
#6447=CARTESIAN_POINT('Ctrl Pts',(42.3088018085782,31.3125763583491,4.97181722452002));
#6448=CARTESIAN_POINT('Ctrl Pts',(41.6998826378874,32.040544413927,5.02474546426192));
#6449=CARTESIAN_POINT('Ctrl Pts',(40.924503628465,32.3460912307927,5.07767370400381));
#6450=CARTESIAN_POINT('Ctrl Pts',(40.1491246190426,32.6516380476584,5.13060194374571));
#6451=CARTESIAN_POINT('Ctrl Pts',(39.2072857708885,32.5347636258119,5.1835301834876));
#6452=CARTESIAN_POINT('Ctrl Pts',(38.5301060375394,32.0489662665249,5.2364584232295));
#6453=CARTESIAN_POINT('Ctrl Pts',(37.886304263532,31.5871136942834,5.28677784798901));
#6454=CARTESIAN_POINT('Ctrl Pts',(37.4817146699033,30.7918100700275,5.33709727274852));
#6455=CARTESIAN_POINT('Ctrl Pts',(37.4785970161092,29.9992487947885,5.38741669750803));
#6456=CARTESIAN_POINT('Origin',(40.,30.,5.));
#6457=CARTESIAN_POINT('',(37.4828502770433,30.0023011685704,6.38741669750802));
#6458=CARTESIAN_POINT('',(37.486585582131,30.0000546151574,6.11258330249198));
#6459=CARTESIAN_POINT('',(37.4825,30.,5.));
#6460=CARTESIAN_POINT('Ctrl Pts',(37.486585582131,30.0000546151574,6.11258330249198));
#6461=CARTESIAN_POINT('Ctrl Pts',(37.4865049295332,30.4169561491143,6.08632864518665));
#6462=CARTESIAN_POINT('Ctrl Pts',(37.584530250577,30.8338220003565,6.06007398788131));
#6463=CARTESIAN_POINT('Ctrl Pts',(37.7808708979026,31.1976286357266,6.03381933057598));
#6464=CARTESIAN_POINT('Ctrl Pts',(38.1766850474407,31.9310468857773,5.98089109083408));
#6465=CARTESIAN_POINT('Ctrl Pts',(38.9720604978366,32.4488282649741,5.92796285109219));
#6466=CARTESIAN_POINT('Ctrl Pts',(39.8029207061802,32.5139626236142,5.87503461135029));
#6467=CARTESIAN_POINT('Ctrl Pts',(40.6337809145239,32.5790969822544,5.8221063716084));
#6468=CARTESIAN_POINT('Ctrl Pts',(41.5001258808154,32.1915843203379,5.7691781318665));
#6469=CARTESIAN_POINT('Ctrl Pts',(42.005393352376,31.5288053581798,5.71624989212461));
#6470=CARTESIAN_POINT('Ctrl Pts',(42.5106608239366,30.8660263960216,5.66332165238271));
#6471=CARTESIAN_POINT('Ctrl Pts',(42.6548508007663,29.9279811336217,5.61039341264082));
#6472=CARTESIAN_POINT('Ctrl Pts',(42.3719615119296,29.1440520419617,5.55746517289892));
#6473=CARTESIAN_POINT('Ctrl Pts',(42.0890722230929,28.3601229503016,5.50453693315703));
#6474=CARTESIAN_POINT('Ctrl Pts',(41.3791036685898,27.7303100293814,5.45160869341513));
#6475=CARTESIAN_POINT('Ctrl Pts',(40.567038090189,27.5429049417591,5.39868045367324));
#6476=CARTESIAN_POINT('Ctrl Pts',(39.7549725117881,27.3554998541367,5.34575221393134));
#6477=CARTESIAN_POINT('Ctrl Pts',(38.8408099094895,27.6105025998123,5.29282397418945));
#6478=CARTESIAN_POINT('Ctrl Pts',(38.2430006638861,28.1911877781685,5.23989573444756));
#6479=CARTESIAN_POINT('Ctrl Pts',(37.7636815626878,28.6567769269077,5.19745825712903));
#6480=CARTESIAN_POINT('Ctrl Pts',(37.4877370393744,29.3317380512216,5.15502077981051));
#6481=CARTESIAN_POINT('Ctrl Pts',(37.4815746018733,30.0022201830298,5.11258330249198));
#6482=CARTESIAN_POINT('Ctrl Pts',(37.4785970161092,29.9992487947885,5.38741669750803));
#6483=CARTESIAN_POINT('Ctrl Pts',(37.4784353810753,29.9581583860809,5.39002551249041));
#6484=CARTESIAN_POINT('Ctrl Pts',(37.4793528677292,29.9170753485691,5.39263432747279));
#6485=CARTESIAN_POINT('Ctrl Pts',(37.4813720877943,29.8760465325149,5.39524314245518));
#6486=CARTESIAN_POINT('Ctrl Pts',(37.5223384899423,29.0436444545195,5.44817138219707));
#6487=CARTESIAN_POINT('Ctrl Pts',(38.0167919127822,28.2335605952563,5.50109962193897));
#6488=CARTESIAN_POINT('Ctrl Pts',(38.7384003859914,27.8166041503647,5.55402786168086));
#6489=CARTESIAN_POINT('Ctrl Pts',(39.4600088592005,27.3996477054731,5.60695610142276));
#6490=CARTESIAN_POINT('Ctrl Pts',(40.4087723827788,27.3758186749531,5.65988434116465));
#6491=CARTESIAN_POINT('Ctrl Pts',(41.1504022902127,27.756024600658,5.71281258090654));
#6492=CARTESIAN_POINT('Ctrl Pts',(41.8920321976466,28.1362305263629,5.76574082064844));
#6493=CARTESIAN_POINT('Ctrl Pts',(42.4265284889361,28.9204714082927,5.81866906039033));
#6494=CARTESIAN_POINT('Ctrl Pts',(42.5092299014576,29.7497674603527,5.87159730013223));
#6495=CARTESIAN_POINT('Ctrl Pts',(42.591931313979,30.5790635124127,5.92452553987413));
#6496=CARTESIAN_POINT('Ctrl Pts',(42.2228378477325,31.4534147346028,5.97745377961602));
#6497=CARTESIAN_POINT('Ctrl Pts',(41.5708989883459,31.9725940765548,6.03038201935791));
#6498=CARTESIAN_POINT('Ctrl Pts',(40.9189601289592,32.4917734185068,6.08331025909981));
#6499=CARTESIAN_POINT('Ctrl Pts',(39.9841758764325,32.6557808802207,6.1362384988417));
#6500=CARTESIAN_POINT('Ctrl Pts',(39.1944360013915,32.3895434011234,6.1891667385836));
#6501=CARTESIAN_POINT('Ctrl Pts',(38.4046961263506,32.123305922026,6.24209497832549));
#6502=CARTESIAN_POINT('Ctrl Pts',(37.7600006287953,31.4268235021173,6.29502321806738));
#6503=CARTESIAN_POINT('Ctrl Pts',(37.5554535478708,30.6189052156672,6.34795145780928));
#6504=CARTESIAN_POINT('Ctrl Pts',(37.5046142755673,30.418100698789,6.36110653770886));
#6505=CARTESIAN_POINT('Ctrl Pts',(37.4809651294343,30.2104122419562,6.37426161760844));
#6506=CARTESIAN_POINT('Ctrl Pts',(37.4828502770433,30.0023011685704,6.38741669750802));
#6507=CARTESIAN_POINT('Origin',(40.,30.,5.));
#6508=CARTESIAN_POINT('',(37.4864394344908,29.9993677916106,7.38741669750803));
#6509=CARTESIAN_POINT('',(37.4817751445882,29.9977519262233,7.11258330249198));
#6510=CARTESIAN_POINT('',(37.4825,30.,5.));
#6511=CARTESIAN_POINT('Ctrl Pts',(37.4817751445882,29.9977519262233,7.11258330249198));
#6512=CARTESIAN_POINT('Ctrl Pts',(37.4879010544836,30.6617513350285,7.07056475030468));
#6513=CARTESIAN_POINT('Ctrl Pts',(37.7578397626965,31.3301554940639,7.02854619811738));
#6514=CARTESIAN_POINT('Ctrl Pts',(38.22877221091,31.7948817330614,6.98652764593008));
#6515=CARTESIAN_POINT('Ctrl Pts',(38.8219774553499,32.3802693895033,6.93359940618818));
#6516=CARTESIAN_POINT('Ctrl Pts',(39.7340979334441,32.6424828443064,6.88067116644629));
#6517=CARTESIAN_POINT('Ctrl Pts',(40.5476180320737,32.4614960518533,6.82774292670439));
#6518=CARTESIAN_POINT('Ctrl Pts',(41.3611381307034,32.2805092594003,6.7748146869625));
#6519=CARTESIAN_POINT('Ctrl Pts',(42.0760578498686,31.6563222196911,6.7218864472206));
#6520=CARTESIAN_POINT('Ctrl Pts',(42.3651285920733,30.8746513958526,6.66895820747871));
#6521=CARTESIAN_POINT('Ctrl Pts',(42.654199334278,30.0929805720141,6.61602996773681));
#6522=CARTESIAN_POINT('Ctrl Pts',(42.5174210995221,29.1538259640462,6.56310172799492));
#6523=CARTESIAN_POINT('Ctrl Pts',(42.0174029955306,28.487077836095,6.51017348825303));
#6524=CARTESIAN_POINT('Ctrl Pts',(41.517384891539,27.8203297081438,6.45724524851113));
#6525=CARTESIAN_POINT('Ctrl Pts',(40.6541269183117,27.4259880602093,6.40431700876923));
#6526=CARTESIAN_POINT('Ctrl Pts',(39.8227782826846,27.4845595248407,6.35138876902734));
#6527=CARTESIAN_POINT('Ctrl Pts',(38.9914296470575,27.5431309894721,6.29846052928544));
#6528=CARTESIAN_POINT('Ctrl Pts',(38.1919903490306,28.0546155666694,6.24553228954355));
#6529=CARTESIAN_POINT('Ctrl Pts',(37.7903971243573,28.7848854157204,6.19260404980166));
#6530=CARTESIAN_POINT('Ctrl Pts',(37.5880112139904,29.1529103701602,6.1659304673651));
#6531=CARTESIAN_POINT('Ctrl Pts',(37.4866675216396,29.5765009079199,6.13925688492854));
#6532=CARTESIAN_POINT('Ctrl Pts',(37.486585582131,30.0000546151574,6.11258330249198));
#6533=CARTESIAN_POINT('Ctrl Pts',(37.4828502770433,30.0023011685704,6.38741669750802));
#6534=CARTESIAN_POINT('Ctrl Pts',(37.488549845404,29.3730967053584,6.42718985735034));
#6535=CARTESIAN_POINT('Ctrl Pts',(37.7276581251219,28.7400291086663,6.46696301719265));
#6536=CARTESIAN_POINT('Ctrl Pts',(38.1544129894185,28.2816695282955,6.50673617703496));
#6537=CARTESIAN_POINT('Ctrl Pts',(38.7223181761841,27.6717062803654,6.55966441677686));
#6538=CARTESIAN_POINT('Ctrl Pts',(39.622527214009,27.3711339374966,6.61259265651875));
#6539=CARTESIAN_POINT('Ctrl Pts',(40.4429768514351,27.5175370039119,6.66552089626065));
#6540=CARTESIAN_POINT('Ctrl Pts',(41.2634264888611,27.6639400703271,6.71844913600254));
#6541=CARTESIAN_POINT('Ctrl Pts',(42.0041167258884,28.2573185460263,6.77137737574444));
#6542=CARTESIAN_POINT('Ctrl Pts',(42.3260027238261,29.026058341056,6.82430561548633));
#6543=CARTESIAN_POINT('Ctrl Pts',(42.6478887217638,29.7947981360857,6.87723385522822));
#6544=CARTESIAN_POINT('Ctrl Pts',(42.5509704806119,30.7388992504459,6.93016209497012));
#6545=CARTESIAN_POINT('Ctrl Pts',(42.0796115257342,31.4262071844781,6.98309033471202));
#6546=CARTESIAN_POINT('Ctrl Pts',(41.6082525708565,32.1135151185102,7.03601857445391));
#6547=CARTESIAN_POINT('Ctrl Pts',(40.7624529022529,32.5440298722143,7.0889468141958));
#6548=CARTESIAN_POINT('Ctrl Pts',(39.9293703303048,32.5206868978311,7.1418750539377));
#6549=CARTESIAN_POINT('Ctrl Pts',(39.0962877583566,32.4973439234479,7.19480329367959));
#6550=CARTESIAN_POINT('Ctrl Pts',(38.2759222830639,32.0201432209773,7.24773153342149));
#6551=CARTESIAN_POINT('Ctrl Pts',(37.8437894287741,31.3075194208077,7.30065977316339));
#6552=CARTESIAN_POINT('Ctrl Pts',(37.6076803275377,30.9181554478826,7.32957874794493));
#6553=CARTESIAN_POINT('Ctrl Pts',(37.4874710852924,30.4585101478601,7.35849772272648));
#6554=CARTESIAN_POINT('Ctrl Pts',(37.4864394344908,29.9993677916106,7.38741669750803));
#6555=CARTESIAN_POINT('Origin',(40.,30.,5.));
#6556=CARTESIAN_POINT('',(37.4805317771007,29.9980220368919,8.38741669750803));
#6557=CARTESIAN_POINT('',(37.4791973108607,30.0013273487219,8.11258330249198));
#6558=CARTESIAN_POINT('',(37.4825,30.,5.));
#6559=CARTESIAN_POINT('Ctrl Pts',(37.4791973108607,30.0013273487219,8.11258330249198));
#6560=CARTESIAN_POINT('Ctrl Pts',(37.4787079525275,30.0778322873578,8.10772909516461));
#6561=CARTESIAN_POINT('Ctrl Pts',(37.4818888734735,30.1542959784042,8.10287488783723));
#6562=CARTESIAN_POINT('Ctrl Pts',(37.4888728396115,30.2304107157375,8.09802068050986));
#6563=CARTESIAN_POINT('Ctrl Pts',(37.5650230757208,31.0603338718311,8.04509244076797));
#6564=CARTESIAN_POINT('Ctrl Pts',(38.0933099956412,31.8487705962177,7.99216420102607));
#6565=CARTESIAN_POINT('Ctrl Pts',(38.8319143740251,32.2348208014644,7.93923596128418));
#6566=CARTESIAN_POINT('Ctrl Pts',(39.570518752409,32.620871006711,7.88630772154228));
#6567=CARTESIAN_POINT('Ctrl Pts',(40.5194405892562,32.6045346928177,7.83337948180038));
#6568=CARTESIAN_POINT('Ctrl Pts',(41.2443188772582,32.1932895167892,7.78045124205849));
#6569=CARTESIAN_POINT('Ctrl Pts',(41.9691971652602,31.7820443407606,7.7275230023166));
#6570=CARTESIAN_POINT('Ctrl Pts',(42.4700319044171,30.9758903025967,7.67459476257471));
#6571=CARTESIAN_POINT('Ctrl Pts',(42.5175700665678,30.1438378327645,7.62166652283281));
#6572=CARTESIAN_POINT('Ctrl Pts',(42.5651082287186,29.3117853629323,7.56873828309092));
#6573=CARTESIAN_POINT('Ctrl Pts',(42.1593498138633,28.4538344614319,7.51581004334902));
#6574=CARTESIAN_POINT('Ctrl Pts',(41.4860274165556,27.962705028035,7.46288180360712));
#6575=CARTESIAN_POINT('Ctrl Pts',(40.8127050192479,27.4715755946381,7.40995356386523));
#6576=CARTESIAN_POINT('Ctrl Pts',(39.8718186394878,27.3472676293449,7.35702532412334));
#6577=CARTESIAN_POINT('Ctrl Pts',(39.0940512304695,27.6466820960993,7.30409708438144));
#6578=CARTESIAN_POINT('Ctrl Pts',(38.3162838214513,27.9460965628537,7.25116884463955));
#6579=CARTESIAN_POINT('Ctrl Pts',(37.7016353831749,28.6692334616558,7.19824060489765));
#6580=CARTESIAN_POINT('Ctrl Pts',(37.5314561694296,29.4850828400972,7.14531236515576));
#6581=CARTESIAN_POINT('Ctrl Pts',(37.4963784479845,29.6532475448712,7.13440267760117));
#6582=CARTESIAN_POINT('Ctrl Pts',(37.480184614704,29.8253512672427,7.12349299004657));
#6583=CARTESIAN_POINT('Ctrl Pts',(37.4817751445882,29.9977519262233,7.11258330249198));
#6584=CARTESIAN_POINT('Ctrl Pts',(37.4864394344908,29.9993677916106,7.38741669750803));
#6585=CARTESIAN_POINT('Ctrl Pts',(37.4855829318786,29.6181761840593,7.41142596246837));
#6586=CARTESIAN_POINT('Ctrl Pts',(37.5668724532984,29.2373312426116,7.43543522742871));
#6587=CARTESIAN_POINT('Ctrl Pts',(37.7321836902776,28.8973394634674,7.45944449238906));
#6588=CARTESIAN_POINT('Ctrl Pts',(38.0966110393577,28.1478302041652,7.51237273213095));
#6589=CARTESIAN_POINT('Ctrl Pts',(38.8693659708049,27.5968585834295,7.56530097187285));
#6590=CARTESIAN_POINT('Ctrl Pts',(39.6967263130212,27.4966271115958,7.61822921161475));
#6591=CARTESIAN_POINT('Ctrl Pts',(40.5240866552375,27.396395639762,7.67115745135664));
#6592=CARTESIAN_POINT('Ctrl Pts',(41.406052408223,27.7469043168303,7.72408569109854));
#6593=CARTESIAN_POINT('Ctrl Pts',(41.9389110020029,28.3877110869611,7.77701393084043));
#6594=CARTESIAN_POINT('Ctrl Pts',(42.4717695957828,29.0285178570919,7.82994217058232));
#6595=CARTESIAN_POINT('Ctrl Pts',(42.6555210303571,29.9596227202852,7.88287041032422));
#6596=CARTESIAN_POINT('Ctrl Pts',(42.4060546666335,30.7548193248618,7.93579865006612));
#6597=CARTESIAN_POINT('Ctrl Pts',(42.1565883029099,31.5500159294385,7.98872688980801));
#6598=CARTESIAN_POINT('Ctrl Pts',(41.4739041408884,32.2093042753983,8.04165512954991));
#6599=CARTESIAN_POINT('Ctrl Pts',(40.670495092448,32.4309021481149,8.0945833692918));
#6600=CARTESIAN_POINT('Ctrl Pts',(39.8670860440077,32.6525000208315,8.1475116090337));
#6601=CARTESIAN_POINT('Ctrl Pts',(38.9429521091486,32.4364074203047,8.20043984877559));
#6602=CARTESIAN_POINT('Ctrl Pts',(38.3211082124662,31.8815357928507,8.25336808851748));
#6603=CARTESIAN_POINT('Ctrl Pts',(37.7961376122345,31.413104257428,8.298050958181));
#6604=CARTESIAN_POINT('Ctrl Pts',(37.4866093473163,30.7032246572373,8.34273382784451));
#6605=CARTESIAN_POINT('Ctrl Pts',(37.4805317771007,29.9980220368919,8.38741669750803));
#6606=CARTESIAN_POINT('Origin',(40.,30.,5.));
#6607=CARTESIAN_POINT('',(37.480218046669,30.0018167092234,9.38741669750803));
#6608=CARTESIAN_POINT('',(37.4857777211518,30.0014129073083,9.11258330249198));
#6609=CARTESIAN_POINT('',(37.4825,30.,5.));
#6610=CARTESIAN_POINT('',(41.9134659966651,31.6359872033749,10.));
#6611=CARTESIAN_POINT('Ctrl Pts',(37.480218046669,30.0018167092234,9.38741669750803));
#6612=CARTESIAN_POINT('Ctrl Pts',(37.4861413026091,29.2855374632777,9.43282641244634));
#6613=CARTESIAN_POINT('Ctrl Pts',(37.8070286664086,28.564752250932,9.47823612738464));
#6614=CARTESIAN_POINT('Ctrl Pts',(38.3470250748122,28.0958621231864,9.52364584232295));
#6615=CARTESIAN_POINT('Ctrl Pts',(38.9764291440202,27.5493374615002,9.57657408206485));
#6616=CARTESIAN_POINT('Ctrl Pts',(39.9035049870189,27.3450262249946,9.62950232180674));
#6617=CARTESIAN_POINT('Ctrl Pts',(40.7037784842569,27.5780866607079,9.68243056154864));
#6618=CARTESIAN_POINT('Ctrl Pts',(41.5040519814949,27.8111470964211,9.73535880129053));
#6619=CARTESIAN_POINT('Ctrl Pts',(42.1775231329722,28.4815792043531,9.78828704103243));
#6620=CARTESIAN_POINT('Ctrl Pts',(42.415891769617,29.278704654386,9.84121528077432));
#6621=CARTESIAN_POINT('Ctrl Pts',(42.6542604062617,30.075830104419,9.89414352051621));
#6622=CARTESIAN_POINT('Ctrl Pts',(42.4575265280738,30.9996488965529,9.94707176025811));
#6623=CARTESIAN_POINT('Ctrl Pts',(41.9134659966651,31.6359872033749,10.));
#6624=CARTESIAN_POINT('',(38.0828938975876,31.638757370194,10.));
#6625=CARTESIAN_POINT('Origin',(40.,30.,10.));
#6626=CARTESIAN_POINT('Ctrl Pts',(38.082890958175,31.6387596071244,10.));
#6627=CARTESIAN_POINT('Ctrl Pts',(38.6136992476573,32.2578638410584,9.94821753066412));
#6628=CARTESIAN_POINT('Ctrl Pts',(39.473300026191,32.5973559811872,9.89643506132825));
#6629=CARTESIAN_POINT('Ctrl Pts',(40.2836371055782,32.5055162560996,9.84465259199238));
#6630=CARTESIAN_POINT('Ctrl Pts',(41.1119041959588,32.4116444294059,9.79172435225048));
#6631=CARTESIAN_POINT('Ctrl Pts',(41.8887033912065,31.867141740819,9.73879611250859));
#6632=CARTESIAN_POINT('Ctrl Pts',(42.2589673171139,31.1206210491648,9.68586787276669));
#6633=CARTESIAN_POINT('Ctrl Pts',(42.6292312430212,30.3741003575106,9.6329396330248));
#6634=CARTESIAN_POINT('Ctrl Pts',(42.5929598995882,29.4255616627892,9.58001139328291));
#6635=CARTESIAN_POINT('Ctrl Pts',(42.1665030878871,28.7095042477308,9.52708315354101));
#6636=CARTESIAN_POINT('Ctrl Pts',(41.740046276186,27.9934468326725,9.47415491379912));
#6637=CARTESIAN_POINT('Ctrl Pts',(40.9234039962168,27.5098706972773,9.42122667405722));
#6638=CARTESIAN_POINT('Ctrl Pts',(40.0905142414943,27.4799719042595,9.36829843431532));
#6639=CARTESIAN_POINT('Ctrl Pts',(39.2576244867719,27.4500731112417,9.31537019457343));
#6640=CARTESIAN_POINT('Ctrl Pts',(38.408487257296,27.8738516606013,9.26244195483154));
#6641=CARTESIAN_POINT('Ctrl Pts',(37.9317246371012,28.557405001666,9.20951371508965));
#6642=CARTESIAN_POINT('Ctrl Pts',(37.640684052642,28.9746813473057,9.17720357755709));
#6643=CARTESIAN_POINT('Ctrl Pts',(37.4884093731962,29.4887631226718,9.14489344002454));
#6644=CARTESIAN_POINT('Ctrl Pts',(37.4857777211518,30.0014129073083,9.11258330249198));
#6645=CARTESIAN_POINT('Origin',(-40.,30.,5.));
#6646=CARTESIAN_POINT('',(-42.5134503279812,30.0006057610914,0.387416697508013));
#6647=CARTESIAN_POINT('',(-42.5156179788862,29.9964982081097,0.112583302491982));
#6648=CARTESIAN_POINT('',(-42.5175,30.,5.));
#6649=CARTESIAN_POINT('',(-41.9134659966651,31.635987203375,0.));
#6650=CARTESIAN_POINT('Ctrl Pts',(-42.5156179788862,29.9964982081097,0.112583302491982));
#6651=CARTESIAN_POINT('Ctrl Pts',(-42.510368759274,30.5890972399227,0.0750555349946548));
#6652=CARTESIAN_POINT('Ctrl Pts',(-42.2992218280841,31.1848035603044,0.0375277674973275));
#6653=CARTESIAN_POINT('Ctrl Pts',(-41.9134659966651,31.635987203375,0.));
#6654=CARTESIAN_POINT('',(-38.0828938060045,31.6387572824072,1.01111975331451E-14));
#6655=CARTESIAN_POINT('Origin',(-40.,30.,0.));
#6656=CARTESIAN_POINT('Ctrl Pts',(-38.0828908636836,31.6387595214235,6.73072708679001E-15));
#6657=CARTESIAN_POINT('Ctrl Pts',(-38.6136991238565,32.2578636190535,0.0517824693358767));
#6658=CARTESIAN_POINT('Ctrl Pts',(-39.4732999763485,32.5973561213315,0.103564938671746));
#6659=CARTESIAN_POINT('Ctrl Pts',(-40.2836371098419,32.5055164690084,0.155347408007616));
#6660=CARTESIAN_POINT('Ctrl Pts',(-41.111904255526,32.4116447166893,0.20827564774951));
#6661=CARTESIAN_POINT('Ctrl Pts',(-41.888703485337,31.8671418001444,0.261203887491404));
#6662=CARTESIAN_POINT('Ctrl Pts',(-42.2589674214213,31.120621033114,0.314132127233298));
#6663=CARTESIAN_POINT('Ctrl Pts',(-42.4298568720969,30.7760762061322,0.33856031732487));
#6664=CARTESIAN_POINT('Ctrl Pts',(-42.514148706906,30.3884987950563,0.362988507416442));
#6665=CARTESIAN_POINT('Ctrl Pts',(-42.5134503279812,30.0006057610914,0.387416697508013));
#6666=CARTESIAN_POINT('Origin',(-40.,30.,5.));
#6667=CARTESIAN_POINT('',(-42.5173482652661,29.997696535754,1.38741669750801));
#6668=CARTESIAN_POINT('',(-42.5216690254717,30.000121302647,1.11258330249199));
#6669=CARTESIAN_POINT('',(-42.5175,30.,5.));
#6670=CARTESIAN_POINT('Ctrl Pts',(-42.5216690254717,30.000121302647,1.11258330249199));
#6671=CARTESIAN_POINT('Ctrl Pts',(-42.5216725769877,30.0058437075332,1.11221987985459));
#6672=CARTESIAN_POINT('Ctrl Pts',(-42.5216547894118,30.0115660877676,1.11185645721719));
#6673=CARTESIAN_POINT('Ctrl Pts',(-42.5216155963134,30.0172883193759,1.11149303457979));
#6674=CARTESIAN_POINT('Ctrl Pts',(-42.515907581752,30.8506641613213,1.0585647948379));
#6675=CARTESIAN_POINT('Ctrl Pts',(-42.0561776880642,31.6808875687602,1.005636555096));
#6676=CARTESIAN_POINT('Ctrl Pts',(-41.3528556457226,32.1280312515289,0.952708315354107));
#6677=CARTESIAN_POINT('Ctrl Pts',(-40.6495336033811,32.5751749342975,0.899780075612213));
#6678=CARTESIAN_POINT('Ctrl Pts',(-39.7026194123857,32.6392388923959,0.846851835870317));
#6679=CARTESIAN_POINT('Ctrl Pts',(-38.9455708556586,32.2906974313558,0.793923596128423));
#6680=CARTESIAN_POINT('Ctrl Pts',(-38.1885222989315,31.9421559703156,0.74099535638653));
#6681=CARTESIAN_POINT('Ctrl Pts',(-37.6213393764727,31.181009090137,0.688067116644636));
#6682=CARTESIAN_POINT('Ctrl Pts',(-37.5036142405306,30.3560669733062,0.635138876902743));
#6683=CARTESIAN_POINT('Ctrl Pts',(-37.3858891045884,29.5311248564754,0.582210637160847));
#6684=CARTESIAN_POINT('Ctrl Pts',(-37.717621755163,28.6423875029925,0.529282397418951));
#6685=CARTESIAN_POINT('Ctrl Pts',(-38.3470255141114,28.0958627356919,0.476354157677056));
#6686=CARTESIAN_POINT('Ctrl Pts',(-38.9764292730598,27.5493379683914,0.423425917935162));
#6687=CARTESIAN_POINT('Ctrl Pts',(-39.9035041403819,27.3450257872733,0.370497678193267));
#6688=CARTESIAN_POINT('Ctrl Pts',(-40.7037780644453,27.5780866271583,0.317569438451373));
#6689=CARTESIAN_POINT('Ctrl Pts',(-41.5040519885087,27.8111474670432,0.264641198709479));
#6690=CARTESIAN_POINT('Ctrl Pts',(-42.1775249693132,28.4815813279313,0.211712958967585));
#6691=CARTESIAN_POINT('Ctrl Pts',(-42.4158936042045,29.2787066853087,0.158784719225691));
#6692=CARTESIAN_POINT('Ctrl Pts',(-42.485251466161,29.5106453819591,0.143384246981121));
#6693=CARTESIAN_POINT('Ctrl Pts',(-42.5177721294348,29.753310148968,0.127983774736552));
#6694=CARTESIAN_POINT('Ctrl Pts',(-42.5156179788862,29.9964982081097,0.112583302491982));
#6695=CARTESIAN_POINT('Ctrl Pts',(-42.5134503279812,30.0006057610914,0.387416697508013));
#6696=CARTESIAN_POINT('Ctrl Pts',(-42.5126355384304,29.5480560353207,0.415916747158336));
#6697=CARTESIAN_POINT('Ctrl Pts',(-42.3961356098422,29.0950766968195,0.444416796808659));
#6698=CARTESIAN_POINT('Ctrl Pts',(-42.1665031701499,28.7095042291822,0.472916846458981));
#6699=CARTESIAN_POINT('Ctrl Pts',(-41.7400463404364,27.9934468097964,0.525845086200876));
#6700=CARTESIAN_POINT('Ctrl Pts',(-40.9234040386519,27.5098705885405,0.578773325942772));
#6701=CARTESIAN_POINT('Ctrl Pts',(-40.0905142507848,27.4799717796994,0.631701565684667));
#6702=CARTESIAN_POINT('Ctrl Pts',(-39.2576244629178,27.4500729708583,0.684629805426561));
#6703=CARTESIAN_POINT('Ctrl Pts',(-38.4084871889682,27.8738515744319,0.737558045168454));
#6704=CARTESIAN_POINT('Ctrl Pts',(-37.9317245473703,28.5574049522032,0.790486284910349));
#6705=CARTESIAN_POINT('Ctrl Pts',(-37.4549619057724,29.2409583299746,0.843414524652243));
#6706=CARTESIAN_POINT('Ctrl Pts',(-37.3505738965262,30.1842864819436,0.896342764394139));
#6707=CARTESIAN_POINT('Ctrl Pts',(-37.6663750453751,30.9555494190257,0.949271004136033));
#6708=CARTESIAN_POINT('Ctrl Pts',(-37.982176194224,31.7268123561078,1.00219924387793));
#6709=CARTESIAN_POINT('Ctrl Pts',(-38.718166501168,32.326010078303,1.05512748361982));
#6710=CARTESIAN_POINT('Ctrl Pts',(-39.5374365691663,32.4788844674016,1.10805572336172));
#6711=CARTESIAN_POINT('Ctrl Pts',(-40.3567066371647,32.6317588565003,1.16098396310361));
#6712=CARTESIAN_POINT('Ctrl Pts',(-41.2592564662174,32.3383099125024,1.2139122028455));
#6713=CARTESIAN_POINT('Ctrl Pts',(-41.831959295633,31.7328516054719,1.2668404425874));
#6714=CARTESIAN_POINT('Ctrl Pts',(-42.2668522922017,31.2730851019424,1.30703252756094));
#6715=CARTESIAN_POINT('Ctrl Pts',(-42.5115416993795,30.6334009370801,1.34722461253448));
#6716=CARTESIAN_POINT('Ctrl Pts',(-42.5173482652661,29.997696535754,1.38741669750801));
#6717=CARTESIAN_POINT('Origin',(-40.,30.,5.));
#6718=CARTESIAN_POINT('',(-42.521313086871,30.0008653513074,2.38741669750802));
#6719=CARTESIAN_POINT('',(-42.515808333435,30.0021290957888,2.11258330249199));
#6720=CARTESIAN_POINT('',(-42.5175,30.,5.));
#6721=CARTESIAN_POINT('Ctrl Pts',(-42.515808333435,30.0021290957888,2.11258330249199));
#6722=CARTESIAN_POINT('Ctrl Pts',(-42.5178586186008,30.2576058506372,2.09645598497262));
#6723=CARTESIAN_POINT('Ctrl Pts',(-42.4820670914407,30.5125215998601,2.08032866745326));
#6724=CARTESIAN_POINT('Ctrl Pts',(-42.4060543110146,30.7548192142433,2.06420134993389));
#6725=CARTESIAN_POINT('Ctrl Pts',(-42.1565879840197,31.5500157004268,2.011273110192));
#6726=CARTESIAN_POINT('Ctrl Pts',(-41.4739039223289,32.2093039453825,1.9583448704501));
#6727=CARTESIAN_POINT('Ctrl Pts',(-40.6704949930077,32.430901786829,1.90541663070821));
#6728=CARTESIAN_POINT('Ctrl Pts',(-39.8670860636866,32.6524996282756,1.85248839096631));
#6729=CARTESIAN_POINT('Ctrl Pts',(-38.9429522667351,32.4364070662131,1.79956015122442));
#6730=CARTESIAN_POINT('Ctrl Pts',(-38.3211084613291,31.8815355180746,1.74663191148252));
#6731=CARTESIAN_POINT('Ctrl Pts',(-37.6992646559231,31.3266639699361,1.69370367174063));
#6732=CARTESIAN_POINT('Ctrl Pts',(-37.3797108420626,30.4330134357218,1.64077543199874));
#6733=CARTESIAN_POINT('Ctrl Pts',(-37.5087196462193,29.6096513927718,1.58784719225684));
#6734=CARTESIAN_POINT('Ctrl Pts',(-37.637728450376,28.7862893498218,1.53491895251495));
#6735=CARTESIAN_POINT('Ctrl Pts',(-38.2152998725499,28.0332157981361,1.48199071277305));
#6736=CARTESIAN_POINT('Ctrl Pts',(-38.9770563481404,27.6951313019726,1.42906247303116));
#6737=CARTESIAN_POINT('Ctrl Pts',(-39.7388128237309,27.3570468058091,1.37613423328926));
#6738=CARTESIAN_POINT('Ctrl Pts',(-40.6847543527379,27.4339513651679,1.32320599354737));
#6739=CARTESIAN_POINT('Ctrl Pts',(-41.3818820495239,27.8906677830732,1.27027775380548));
#6740=CARTESIAN_POINT('Ctrl Pts',(-42.0742230391115,28.344248236398,1.21771293670098));
#6741=CARTESIAN_POINT('Ctrl Pts',(-42.5211553403926,29.1724426297002,1.16514811959648));
#6742=CARTESIAN_POINT('Ctrl Pts',(-42.5216690254717,30.000121302647,1.11258330249199));
#6743=CARTESIAN_POINT('Ctrl Pts',(-42.5173482652661,29.997696535754,1.38741669750801));
#6744=CARTESIAN_POINT('Ctrl Pts',(-42.5191882624162,29.79625315088,1.40015285227637));
#6745=CARTESIAN_POINT('Ctrl Pts',(-42.4970410052288,29.595209391193,1.41288900704473));
#6746=CARTESIAN_POINT('Ctrl Pts',(-42.4493575441589,29.4004167811413,1.42562516181308));
#6747=CARTESIAN_POINT('Ctrl Pts',(-42.2511971334908,28.5909079339042,1.47855340155498));
#6748=CARTESIAN_POINT('Ctrl Pts',(-41.6120204823761,27.8893579094928,1.53148164129687));
#6749=CARTESIAN_POINT('Ctrl Pts',(-40.8244074219312,27.6168929643317,1.58440988103877));
#6750=CARTESIAN_POINT('Ctrl Pts',(-40.0367943614864,27.3444280191707,1.63733812078066));
#6751=CARTESIAN_POINT('Ctrl Pts',(-39.1007448917115,27.50104815326,1.69026636052255));
#6752=CARTESIAN_POINT('Ctrl Pts',(-38.4447269252528,28.0150630321248,1.74319460026445));
#6753=CARTESIAN_POINT('Ctrl Pts',(-37.7887089587941,28.5290779109896,1.79612284000634));
#6754=CARTESIAN_POINT('Ctrl Pts',(-37.4127224956517,29.4004875346298,1.84905107974824));
#6755=CARTESIAN_POINT('Ctrl Pts',(-37.4888727349885,30.2304107252086,1.90197931949013));
#6756=CARTESIAN_POINT('Ctrl Pts',(-37.5650229743253,31.0603339157874,1.95490755923203));
#6757=CARTESIAN_POINT('Ctrl Pts',(-38.0933099161414,31.8487706733048,2.00783579897392));
#6758=CARTESIAN_POINT('Ctrl Pts',(-38.8319143252891,32.2348208947076,2.06076403871582));
#6759=CARTESIAN_POINT('Ctrl Pts',(-39.5705187344369,32.6208711161104,2.11369227845771));
#6760=CARTESIAN_POINT('Ctrl Pts',(-40.5194406109162,32.6045348013986,2.16662051819961));
#6761=CARTESIAN_POINT('Ctrl Pts',(-41.2443189291553,32.1932896081922,2.2195487579415));
#6762=CARTESIAN_POINT('Ctrl Pts',(-41.9691972473944,31.7820444149859,2.27247699768339));
#6763=CARTESIAN_POINT('Ctrl Pts',(-42.4700320073933,30.975890343285,2.32540523742529));
#6764=CARTESIAN_POINT('Ctrl Pts',(-42.5175701715172,30.1438378387809,2.37833347716718));
#6765=CARTESIAN_POINT('Ctrl Pts',(-42.5202895743756,30.0962405871662,2.3813612172808));
#6766=CARTESIAN_POINT('Ctrl Pts',(-42.5215256234437,30.0485585863193,2.38438895739441));
#6767=CARTESIAN_POINT('Ctrl Pts',(-42.521313086871,30.0008653513074,2.38741669750802));
#6768=CARTESIAN_POINT('Origin',(-40.,30.,5.));
#6769=CARTESIAN_POINT('',(-42.5147865997281,30.0017637212727,3.38741669750802));
#6770=CARTESIAN_POINT('',(-42.5141171500829,29.9986698323151,3.11258330249199));
#6771=CARTESIAN_POINT('',(-42.5175,30.,5.));
#6772=CARTESIAN_POINT('Ctrl Pts',(-42.5141171500829,29.9986698323151,3.11258330249199));
#6773=CARTESIAN_POINT('Ctrl Pts',(-42.5116924647915,30.5047215402099,3.08069209009066));
#6774=CARTESIAN_POINT('Ctrl Pts',(-42.3636222943308,31.0120787091108,3.04880087768933));
#6775=CARTESIAN_POINT('Ctrl Pts',(-42.0796112182407,31.4262069736182,3.01690966528799));
#6776=CARTESIAN_POINT('Ctrl Pts',(-41.608252333057,32.1135148060047,2.9639814255461));
#6777=CARTESIAN_POINT('Ctrl Pts',(-40.7624527895073,32.544029495972,2.9110531858042));
#6778=CARTESIAN_POINT('Ctrl Pts',(-39.9293703407444,32.5206865250762,2.85812494606231));
#6779=CARTESIAN_POINT('Ctrl Pts',(-39.0962878919816,32.4973435541803,2.80519670632041));
#6780=CARTESIAN_POINT('Ctrl Pts',(-38.2759225380058,32.0201429224212,2.75226846657852));
#6781=CARTESIAN_POINT('Ctrl Pts',(-37.8437897476033,31.307519227554,2.69934022683663));
#6782=CARTESIAN_POINT('Ctrl Pts',(-37.4116569572008,30.5948955326869,2.64641198709473));
#6783=CARTESIAN_POINT('Ctrl Pts',(-37.3677567303717,29.6468487747117,2.59348374735284));
#6784=CARTESIAN_POINT('Ctrl Pts',(-37.7321840255849,28.89733962636,2.54055550761094));
#6785=CARTESIAN_POINT('Ctrl Pts',(-38.096611320798,28.1478304780083,2.48762726786905));
#6786=CARTESIAN_POINT('Ctrl Pts',(-38.8693661380534,27.5968589392801,2.43469902812715));
#6787=CARTESIAN_POINT('Ctrl Pts',(-39.6967263578976,27.4966274820302,2.38177078838526));
#6788=CARTESIAN_POINT('Ctrl Pts',(-40.5240865777418,27.3963960247803,2.32884254864336));
#6789=CARTESIAN_POINT('Ctrl Pts',(-41.4060522001749,27.7469046490088,2.27591430890147));
#6790=CARTESIAN_POINT('Ctrl Pts',(-41.9389107152419,28.3877113248286,2.22298606915957));
#6791=CARTESIAN_POINT('Ctrl Pts',(-42.3094064064687,28.833263203212,2.18618514693704));
#6792=CARTESIAN_POINT('Ctrl Pts',(-42.5111297881759,29.4191567463233,2.14938422471451));
#6793=CARTESIAN_POINT('Ctrl Pts',(-42.515808333435,30.0021290957888,2.11258330249199));
#6794=CARTESIAN_POINT('Ctrl Pts',(-42.521313086871,30.0008653513074,2.38741669750802));
#6795=CARTESIAN_POINT('Ctrl Pts',(-42.5178102495169,29.2148281860683,2.4373171971363));
#6796=CARTESIAN_POINT('Ctrl Pts',(-42.1208327469498,28.4257395206662,2.48721769676458));
#6797=CARTESIAN_POINT('Ctrl Pts',(-41.4860274785154,27.9627049430877,2.53711819639287));
#6798=CARTESIAN_POINT('Ctrl Pts',(-40.812705053141,27.4715754892061,2.59004643613476));
#6799=CARTESIAN_POINT('Ctrl Pts',(-39.8718186341432,27.3472675187503,2.64297467587666));
#6800=CARTESIAN_POINT('Ctrl Pts',(-39.0940511926965,27.6466819979924,2.69590291561855));
#6801=CARTESIAN_POINT('Ctrl Pts',(-38.3162837512497,27.9460964772345,2.74883115536045));
#6802=CARTESIAN_POINT('Ctrl Pts',(-37.701635287354,28.6692334061744,2.80175939510234));
#6803=CARTESIAN_POINT('Ctrl Pts',(-37.5314560665151,29.485082818627,2.85468763484424));
#6804=CARTESIAN_POINT('Ctrl Pts',(-37.3612768456762,30.3009322310796,2.90761587458613));
#6805=CARTESIAN_POINT('Ctrl Pts',(-37.6355668678942,31.2094941270447,2.96054411432802));
#6806=CARTESIAN_POINT('Ctrl Pts',(-38.2287721370648,31.7948818078934,3.01347235406992));
#6807=CARTESIAN_POINT('Ctrl Pts',(-38.8219774062353,32.380269488742,3.06640059381181));
#6808=CARTESIAN_POINT('Ctrl Pts',(-39.7340979223584,32.6424829544742,3.11932883355371));
#6809=CARTESIAN_POINT('Ctrl Pts',(-40.547618054905,32.4614961544749,3.1722570732956));
#6810=CARTESIAN_POINT('Ctrl Pts',(-41.3611381874516,32.2805093544756,3.2251853130375));
#6811=CARTESIAN_POINT('Ctrl Pts',(-42.0760579364217,31.656322288745,3.27811355277939));
#6812=CARTESIAN_POINT('Ctrl Pts',(-42.3651286906778,30.8746514323181,3.33104179252129));
#6813=CARTESIAN_POINT('Ctrl Pts',(-42.4677603317142,30.5971271184115,3.34983342751686));
#6814=CARTESIAN_POINT('Ctrl Pts',(-42.5167122997757,30.2997514522924,3.36862506251244));
#6815=CARTESIAN_POINT('Ctrl Pts',(-42.5147865997281,30.0017637212727,3.38741669750802));
#6816=CARTESIAN_POINT('Origin',(-40.,30.,5.));
#6817=CARTESIAN_POINT('',(-42.51493238455,29.9981671625222,4.38741669750802));
#6818=CARTESIAN_POINT('',(-42.52066153614,29.998576517643,4.11258330249199));
#6819=CARTESIAN_POINT('',(-42.5175,30.,5.));
#6820=CARTESIAN_POINT('Ctrl Pts',(-42.52066153614,29.998576517643,4.11258330249199));
#6821=CARTESIAN_POINT('Ctrl Pts',(-42.515579438117,30.7497577154419,4.06492819520869));
#6822=CARTESIAN_POINT('Ctrl Pts',(-42.1578861912069,31.5051392898487,4.01727308792539));
#6823=CARTESIAN_POINT('Ctrl Pts',(-41.5708987560698,31.9725937848838,3.96961798064209));
#6824=CARTESIAN_POINT('Ctrl Pts',(-40.91895999308,32.4917730500686,3.9166897409002));
#6825=CARTESIAN_POINT('Ctrl Pts',(-39.9841758787722,32.6557804875304,3.86376150115831));
#6826=CARTESIAN_POINT('Ctrl Pts',(-39.1944361205037,32.3895430478001,3.81083326141641));
#6827=CARTESIAN_POINT('Ctrl Pts',(-38.4046963622352,32.1233056080699,3.75790502167452));
#6828=CARTESIAN_POINT('Ctrl Pts',(-37.760000960006,31.4268232911476,3.70497678193262));
#6829=CARTESIAN_POINT('Ctrl Pts',(-37.5554539093262,30.6189051241564,3.65204854219073));
#6830=CARTESIAN_POINT('Ctrl Pts',(-37.3509068586463,29.8109869571652,3.59912030244883));
#6831=CARTESIAN_POINT('Ctrl Pts',(-37.5865081595159,28.891632940105,3.54619206270694));
#6832=CARTESIAN_POINT('Ctrl Pts',(-38.1544132623102,28.281669782368,3.49326382296504));
#6833=CARTESIAN_POINT('Ctrl Pts',(-38.7223183651046,27.6717066246309,3.44033558322315));
#6834=CARTESIAN_POINT('Ctrl Pts',(-39.6225272698237,27.371134326217,3.38740734348126));
#6835=CARTESIAN_POINT('Ctrl Pts',(-40.4429767859361,27.5175373709795,3.33447910373936));
#6836=CARTESIAN_POINT('Ctrl Pts',(-41.2634263020485,27.663940415742,3.28155086399747));
#6837=CARTESIAN_POINT('Ctrl Pts',(-42.0041164295541,28.257318803681,3.22862262425557));
#6838=CARTESIAN_POINT('Ctrl Pts',(-42.3260023798981,29.0260584850534,3.17569438451368));
#6839=CARTESIAN_POINT('Ctrl Pts',(-42.453940198555,29.3316042159084,3.15465735717311));
#6840=CARTESIAN_POINT('Ctrl Pts',(-42.5157165929052,29.664852996481,3.13362032983255));
#6841=CARTESIAN_POINT('Ctrl Pts',(-42.5141171500829,29.9986698323151,3.11258330249199));
#6842=CARTESIAN_POINT('Ctrl Pts',(-42.5147865997281,30.0017637212727,3.38741669750802));
#6843=CARTESIAN_POINT('Ctrl Pts',(-42.5112884016521,29.4604436394667,3.42155330225433));
#6844=CARTESIAN_POINT('Ctrl Pts',(-42.3398948378532,28.9171037547851,3.45568990700065));
#6845=CARTESIAN_POINT('Ctrl Pts',(-42.0174030796383,28.4870777730195,3.48982651174697));
#6846=CARTESIAN_POINT('Ctrl Pts',(-41.5173849548006,27.8203296172707,3.54275475148886));
#6847=CARTESIAN_POINT('Ctrl Pts',(-40.6541269455829,27.4259879528961,3.59568299123076));
#6848=CARTESIAN_POINT('Ctrl Pts',(-39.8227782752959,27.4845594199695,3.64861123097265));
#6849=CARTESIAN_POINT('Ctrl Pts',(-38.991429605009,27.5431308870429,3.70153947071455));
#6850=CARTESIAN_POINT('Ctrl Pts',(-38.1919902736528,28.0546154855643,3.75446771045644));
#6851=CARTESIAN_POINT('Ctrl Pts',(-37.7903970322367,28.7848853650609,3.80739595019834));
#6852=CARTESIAN_POINT('Ctrl Pts',(-37.3888037908207,29.5151552445575,3.86032418994023));
#6853=CARTESIAN_POINT('Ctrl Pts',(-37.3850566393447,30.4642104050294,3.91325242968213));
#6854=CARTESIAN_POINT('Ctrl Pts',(-37.7808708053848,31.1976286856571,3.96618066942402));
#6855=CARTESIAN_POINT('Ctrl Pts',(-38.1766849714248,31.9310469662847,4.01910890916591));
#6856=CARTESIAN_POINT('Ctrl Pts',(-38.9720604549807,32.4488283670683,4.07203714890781));
#6857=CARTESIAN_POINT('Ctrl Pts',(-39.8029206979638,32.513962728424,4.1249653886497));
#6858=CARTESIAN_POINT('Ctrl Pts',(-40.6337809409469,32.5790970897796,4.1778936283916));
#6859=CARTESIAN_POINT('Ctrl Pts',(-41.5001259433573,32.1915844117074,4.23082186813349));
#6860=CARTESIAN_POINT('Ctrl Pts',(-42.005393435983,31.5288054219173,4.28375010787539));
#6861=CARTESIAN_POINT('Ctrl Pts',(-42.3352700013614,31.0960935218884,4.31830563775293));
#6862=CARTESIAN_POINT('Ctrl Pts',(-42.5112387594207,30.5460504856982,4.35286116763047));
#6863=CARTESIAN_POINT('Ctrl Pts',(-42.51493238455,29.9981671625222,4.38741669750802));
#6864=CARTESIAN_POINT('Origin',(-40.,30.,5.));
#6865=CARTESIAN_POINT('',(-42.5214025534547,29.9992487949168,5.38741669750802));
#6866=CARTESIAN_POINT('',(-42.5184255606712,30.0022201831731,5.11258330249199));
#6867=CARTESIAN_POINT('',(-42.5175,30.,5.));
#6868=CARTESIAN_POINT('Ctrl Pts',(-42.5184255606712,30.0022201831731,5.11258330249199));
#6869=CARTESIAN_POINT('Ctrl Pts',(-42.5199489469804,30.1679668215771,5.10209254006862));
#6870=CARTESIAN_POINT('Ctrl Pts',(-42.5049858464185,30.3334397470291,5.09160177764525));
#6871=CARTESIAN_POINT('Ctrl Pts',(-42.4725330539849,30.4954083555317,5.08111101522188));
#6872=CARTESIAN_POINT('Ctrl Pts',(-42.3088014671944,31.3125761642691,5.02818277547999));
#6873=CARTESIAN_POINT('Ctrl Pts',(-41.6998823865396,32.0405441122082,4.97525453573809));
#6874=CARTESIAN_POINT('Ctrl Pts',(-40.9245034917662,32.3460908838952,4.9223262959962));
#6875=CARTESIAN_POINT('Ctrl Pts',(-40.1491245969927,32.6516376555822,4.8693980562543));
#6876=CARTESIAN_POINT('Ctrl Pts',(-39.2072858881007,32.534763251017,4.81646981651241));
#6877=CARTESIAN_POINT('Ctrl Pts',(-38.5301062548807,32.0489659635609,4.76354157677051));
#6878=CARTESIAN_POINT('Ctrl Pts',(-37.8529266216607,31.5631686761048,4.71061333702862));
#6879=CARTESIAN_POINT('Ctrl Pts',(-37.4404060641128,30.7084485057578,4.65768509728672));
#6880=CARTESIAN_POINT('Ctrl Pts',(-37.4813724602034,29.8760465508429,4.60475685754483));
#6881=CARTESIAN_POINT('Ctrl Pts',(-37.522338856294,29.043644595928,4.55182861780293));
#6882=CARTESIAN_POINT('Ctrl Pts',(-38.0167922060231,28.2335608564452,4.49890037806104));
#6883=CARTESIAN_POINT('Ctrl Pts',(-38.7384005725339,27.8166044732056,4.44597213831915));
#6884=CARTESIAN_POINT('Ctrl Pts',(-39.4600089390446,27.399648089966,4.39304389857725));
#6885=CARTESIAN_POINT('Ctrl Pts',(-40.408772322337,27.3758190629697,4.34011565883535));
#6886=CARTESIAN_POINT('Ctrl Pts',(-41.1504021201121,27.7560249324566,4.28718741909346));
#6887=CARTESIAN_POINT('Ctrl Pts',(-41.8920319178872,28.1362308019434,4.23425917935157));
#6888=CARTESIAN_POINT('Ctrl Pts',(-42.4265281301451,28.9204715679134,4.18133093960967));
#6889=CARTESIAN_POINT('Ctrl Pts',(-42.5092295304381,29.7497674973523,4.12840269986778));
#6890=CARTESIAN_POINT('Ctrl Pts',(-42.5174689020927,29.8323885575771,4.12312956740918));
#6891=CARTESIAN_POINT('Ctrl Pts',(-42.5212238804001,29.9154568231924,4.11785643495059));
#6892=CARTESIAN_POINT('Ctrl Pts',(-42.52066153614,29.998576517643,4.11258330249199));
#6893=CARTESIAN_POINT('Ctrl Pts',(-42.51493238455,29.9981671625222,4.38741669750802));
#6894=CARTESIAN_POINT('Ctrl Pts',(-42.5168962352879,29.7068649781279,4.40578940737237));
#6895=CARTESIAN_POINT('Ctrl Pts',(-42.4701595306737,29.4161733242344,4.42416211723672));
#6896=CARTESIAN_POINT('Ctrl Pts',(-42.3719616108191,29.1440520062763,4.44253482710107));
#6897=CARTESIAN_POINT('Ctrl Pts',(-42.0890723101885,28.3601228819334,4.49546306684297));
#6898=CARTESIAN_POINT('Ctrl Pts',(-41.3791037260861,27.7303099347556,4.54839130658486));
#6899=CARTESIAN_POINT('Ctrl Pts',(-40.5670381138294,27.5429048393202,4.60131954632675));
#6900=CARTESIAN_POINT('Ctrl Pts',(-39.7549725015727,27.3554997438847,4.65424778606865));
#6901=CARTESIAN_POINT('Ctrl Pts',(-38.8408098611616,27.6105025001917,4.70717602581054));
#6902=CARTESIAN_POINT('Ctrl Pts',(-38.243000590635,28.1911877027572,4.76010426555244));
#6903=CARTESIAN_POINT('Ctrl Pts',(-37.6451913201083,28.7718729053228,4.81303250529433));
#6904=CARTESIAN_POINT('Ctrl Pts',(-37.363735419466,29.678240554147,4.86596074503623));
#6905=CARTESIAN_POINT('Ctrl Pts',(-37.5274670025151,30.4954083442112,4.91888898477812));
#6906=CARTESIAN_POINT('Ctrl Pts',(-37.6911985855641,31.3125761342754,4.97181722452002));
#6907=CARTESIAN_POINT('Ctrl Pts',(-38.3001176523045,32.0405440655797,5.02474546426191));
#6908=CARTESIAN_POINT('Ctrl Pts',(-39.0754965293597,32.3460908302846,5.07767370400381));
#6909=CARTESIAN_POINT('Ctrl Pts',(-39.850875406415,32.6516375949895,5.1306019437457));
#6910=CARTESIAN_POINT('Ctrl Pts',(-40.792714093785,32.534763193095,5.18353018348759));
#6911=CARTESIAN_POINT('Ctrl Pts',(-41.4698937115307,32.0489659167399,5.23645842322949));
#6912=CARTESIAN_POINT('Ctrl Pts',(-42.1136953756329,31.5871134233426,5.286777847989));
#6913=CARTESIAN_POINT('Ctrl Pts',(-42.5182849001928,30.7918099348553,5.33709727274851));
#6914=CARTESIAN_POINT('Ctrl Pts',(-42.5214025534547,29.9992487949168,5.38741669750802));
#6915=CARTESIAN_POINT('Origin',(-40.,30.,5.));
#6916=CARTESIAN_POINT('',(-42.5171492932468,30.0023011681775,6.38741669750801));
#6917=CARTESIAN_POINT('',(-42.51341458009,30.0000546151609,6.11258330249199));
#6918=CARTESIAN_POINT('',(-42.5175,30.,5.));
#6919=CARTESIAN_POINT('Ctrl Pts',(-42.51341458009,30.0000546151609,6.11258330249199));
#6920=CARTESIAN_POINT('Ctrl Pts',(-42.5134952326931,30.4169561760255,6.08632864518665));
#6921=CARTESIAN_POINT('Ctrl Pts',(-42.4154699053225,30.8338220541732,6.06007398788132));
#6922=CARTESIAN_POINT('Ctrl Pts',(-42.2191292453247,31.1976287130241,6.03381933057598));
#6923=CARTESIAN_POINT('Ctrl Pts',(-41.8233150702399,31.9310470104112,5.98089109083409));
#6924=CARTESIAN_POINT('Ctrl Pts',(-41.0279395685088,32.4488284230266,5.9279628510922));
#6925=CARTESIAN_POINT('Ctrl Pts',(-40.1970793065397,32.5139627858706,5.8750346113503));
#6926=CARTESIAN_POINT('Ctrl Pts',(-39.3662190445705,32.5790971487147,5.82210637160841));
#6927=CARTESIAN_POINT('Ctrl Pts',(-38.4998740223633,32.1915844617874,5.76917813186651));
#6928=CARTESIAN_POINT('Ctrl Pts',(-37.9946065181917,31.5288054568521,5.71624989212461));
#6929=CARTESIAN_POINT('Ctrl Pts',(-37.4893390140201,30.8660264519168,5.66332165238272));
#6930=CARTESIAN_POINT('Ctrl Pts',(-37.3451490278841,29.9279811289735,5.61039341264083));
#6931=CARTESIAN_POINT('Ctrl Pts',(-37.6280383349791,29.144051986717,5.55746517289893));
#6932=CARTESIAN_POINT('Ctrl Pts',(-37.910927642074,28.3601228444605,5.50453693315704));
#6933=CARTESIAN_POINT('Ctrl Pts',(-38.6208962423999,27.7303098828908,5.45160869341514));
#6934=CARTESIAN_POINT('Ctrl Pts',(-39.4329618732132,27.542904783173,5.39868045367325));
#6935=CARTESIAN_POINT('Ctrl Pts',(-40.2450275040264,27.3554996834551,5.34575221393135));
#6936=CARTESIAN_POINT('Ctrl Pts',(-41.159190165327,27.6105024455891,5.29282397418946));
#6937=CARTESIAN_POINT('Ctrl Pts',(-41.7569994495142,28.1911876614239,5.23989573444757));
#6938=CARTESIAN_POINT('Ctrl Pts',(-42.2363185816489,28.6567768402132,5.19745825712904));
#6939=CARTESIAN_POINT('Ctrl Pts',(-42.5122631227723,29.3317380080906,5.15502077981052));
#6940=CARTESIAN_POINT('Ctrl Pts',(-42.5184255606712,30.0022201831731,5.11258330249199));
#6941=CARTESIAN_POINT('Ctrl Pts',(-42.5214025534547,29.9992487949168,5.38741669750802));
#6942=CARTESIAN_POINT('Ctrl Pts',(-42.5215641884611,29.9581583932238,5.3900255124904));
#6943=CARTESIAN_POINT('Ctrl Pts',(-42.5206467019638,29.9170753627254,5.39263432747279));
#6944=CARTESIAN_POINT('Ctrl Pts',(-42.5186274822434,29.8760465536754,5.39524314245517));
#6945=CARTESIAN_POINT('Ctrl Pts',(-42.4776610870889,29.0436446177817,5.44817138219707));
#6946=CARTESIAN_POINT('Ctrl Pts',(-41.9832077486585,28.2335608968101,5.50109962193896));
#6947=CARTESIAN_POINT('Ctrl Pts',(-41.2615993986372,27.8166045230985,5.55402786168086));
#6948=CARTESIAN_POINT('Ctrl Pts',(-40.539991048616,27.3996481493868,5.60695610142275));
#6949=CARTESIAN_POINT('Ctrl Pts',(-39.5912276870039,27.375819122935,5.65988434116464));
#6950=CARTESIAN_POINT('Ctrl Pts',(-38.8495979061758,27.7560249837337,5.71281258090654));
#6951=CARTESIAN_POINT('Ctrl Pts',(-38.1079681253477,28.1362308445325,5.76574082064843));
#6952=CARTESIAN_POINT('Ctrl Pts',(-37.5734719253036,28.9204715925817,5.81866906039033));
#6953=CARTESIAN_POINT('Ctrl Pts',(-37.4907705269003,29.7497675030704,5.87159730013222));
#6954=CARTESIAN_POINT('Ctrl Pts',(-37.4080691284971,30.5790634135591,5.92452553987411));
#6955=CARTESIAN_POINT('Ctrl Pts',(-37.7771625317346,31.4534144864871,5.97745377961601));
#6956=CARTESIAN_POINT('Ctrl Pts',(-38.4291012798269,31.9725937398081,6.0303820193579));
#6957=CARTESIAN_POINT('Ctrl Pts',(-39.0810400279192,32.491772993129,6.0833102590998));
#6958=CARTESIAN_POINT('Ctrl Pts',(-40.0158241208662,32.6557804268428,6.13623849884169));
#6959=CARTESIAN_POINT('Ctrl Pts',(-40.8055638610884,32.3895429931965,6.18916673858359));
#6960=CARTESIAN_POINT('Ctrl Pts',(-41.5953036013105,32.1233055595501,6.24209497832548));
#6961=CARTESIAN_POINT('Ctrl Pts',(-42.2399989888077,31.4268232585436,6.29502321806738));
#6962=CARTESIAN_POINT('Ctrl Pts',(-42.4445460348134,30.6189051100139,6.34795145780927));
#6963=CARTESIAN_POINT('Ctrl Pts',(-42.4953852984381,30.4181006274153,6.36110653770885));
#6964=CARTESIAN_POINT('Ctrl Pts',(-42.5190344405339,30.2104122060369,6.37426161760843));
#6965=CARTESIAN_POINT('Ctrl Pts',(-42.5171492932468,30.0023011681775,6.38741669750801));
#6966=CARTESIAN_POINT('Origin',(-40.,30.,5.));
#6967=CARTESIAN_POINT('',(-42.5135601364305,29.999367791574,7.38741669750801));
#6968=CARTESIAN_POINT('',(-42.5182250179402,29.9977519260729,7.11258330249199));
#6969=CARTESIAN_POINT('',(-42.5175,30.,5.));
#6970=CARTESIAN_POINT('Ctrl Pts',(-42.5182250179402,29.9977519260729,7.11258330249199));
#6971=CARTESIAN_POINT('Ctrl Pts',(-42.5120991076497,30.6617513777343,7.07056475030469));
#6972=CARTESIAN_POINT('Ctrl Pts',(-42.2421603820176,31.3301555799156,7.02854619811739));
#6973=CARTESIAN_POINT('Ctrl Pts',(-41.7712279034101,31.7948818489091,6.98652764593008));
#6974=CARTESIAN_POINT('Ctrl Pts',(-41.1780226206846,32.3802695431352,6.93359940618819));
#6975=CARTESIAN_POINT('Ctrl Pts',(-40.2659020837177,32.6424830148576,6.8806711664463));
#6976=CARTESIAN_POINT('Ctrl Pts',(-39.4523819325812,32.4614962107223,6.8277429267044));
#6977=CARTESIAN_POINT('Ctrl Pts',(-38.6388617814446,32.2805094065869,6.77481468696251));
#6978=CARTESIAN_POINT('Ctrl Pts',(-37.9239420161383,31.6563223265937,6.72188644722061));
#6979=CARTESIAN_POINT('Ctrl Pts',(-37.6348712552767,30.8746514523051,6.66895820747871));
#6980=CARTESIAN_POINT('Ctrl Pts',(-37.3458004944151,30.0929805780164,6.61602996773682));
#6981=CARTESIAN_POINT('Ctrl Pts',(-37.4825787379982,29.1538259094324,6.56310172799493));
#6982=CARTESIAN_POINT('Ctrl Pts',(-37.9825968742618,28.4870777384476,6.51017348825303));
#6983=CARTESIAN_POINT('Ctrl Pts',(-38.4826150105254,27.8203295674628,6.45724524851114));
#6984=CARTESIAN_POINT('Ctrl Pts',(-39.3458730394696,27.4259878940772,6.40431700876925));
#6985=CARTESIAN_POINT('Ctrl Pts',(-40.1772217287538,27.4845593624891,6.35138876902735));
#6986=CARTESIAN_POINT('Ctrl Pts',(-41.008570418038,27.5431308309009,6.29846052928545));
#6987=CARTESIAN_POINT('Ctrl Pts',(-41.8080097676621,28.0546154411102,6.24553228954356));
#6988=CARTESIAN_POINT('Ctrl Pts',(-42.209603018255,28.7848853372942,6.19260404980166));
#6989=CARTESIAN_POINT('Ctrl Pts',(-42.4119889416843,29.1529103154872,6.1659304673651));
#6990=CARTESIAN_POINT('Ctrl Pts',(-42.5133326405761,29.5765008805862,6.13925688492855));
#6991=CARTESIAN_POINT('Ctrl Pts',(-42.51341458009,30.0000546151609,6.11258330249199));
#6992=CARTESIAN_POINT('Ctrl Pts',(-42.5171492932468,30.0023011681775,6.38741669750801));
#6993=CARTESIAN_POINT('Ctrl Pts',(-42.5114497258593,29.3730968123762,6.42718985735033));
#6994=CARTESIAN_POINT('Ctrl Pts',(-42.2723414869604,28.7400293237536,6.46696301719264));
#6995=CARTESIAN_POINT('Ctrl Pts',(-41.8455866955162,28.2816698216331,6.50673617703495));
#6996=CARTESIAN_POINT('Ctrl Pts',(-41.277681605699,27.6717066778348,6.55966441677685));
#6997=CARTESIAN_POINT('Ctrl Pts',(-40.3774727215505,27.371134386291,6.61259265651875));
#6998=CARTESIAN_POINT('Ctrl Pts',(-39.5570232241863,27.5175374277073,6.66552089626064));
#6999=CARTESIAN_POINT('Ctrl Pts',(-38.7365737268221,27.6639404691235,6.71844913600254));
#7000=CARTESIAN_POINT('Ctrl Pts',(-37.9958836162423,28.2573188434998,6.77137737574443));
#7001=CARTESIAN_POINT('Ctrl Pts',(-37.6739976732536,29.0260585073073,6.82430561548633));
#7002=CARTESIAN_POINT('Ctrl Pts',(-37.3521117302649,29.7947981711147,6.87723385522822));
#7003=CARTESIAN_POINT('Ctrl Pts',(-37.4490299548673,30.7388991243533,6.93016209497011));
#7004=CARTESIAN_POINT('Ctrl Pts',(-37.9203888292803,31.4262069410312,6.983090334712));
#7005=CARTESIAN_POINT('Ctrl Pts',(-38.3917477036933,32.1135147577091,7.0360185744539));
#7006=CARTESIAN_POINT('Ctrl Pts',(-39.2375472279169,32.5440294378263,7.0889468141958));
#7007=CARTESIAN_POINT('Ctrl Pts',(-40.0706296576422,32.5206864674694,7.14187505393769));
#7008=CARTESIAN_POINT('Ctrl Pts',(-40.9037120873676,32.4973434971125,7.19480329367959));
#7009=CARTESIAN_POINT('Ctrl Pts',(-41.7240774225947,32.0201428762815,7.24773153342148));
#7010=CARTESIAN_POINT('Ctrl Pts',(-42.1562102031238,31.3075191976881,7.30065977316337));
#7011=CARTESIAN_POINT('Ctrl Pts',(-42.3923192640589,30.9181552911899,7.32957874794492));
#7012=CARTESIAN_POINT('Ctrl Pts',(-42.5125284857968,30.4585100695166,7.35849772272647));
#7013=CARTESIAN_POINT('Ctrl Pts',(-42.5135601364305,29.999367791574,7.38741669750801));
#7014=CARTESIAN_POINT('Origin',(-40.,30.,5.));
#7015=CARTESIAN_POINT('',(-42.5194677947045,29.9980220285566,8.38741669750802));
#7016=CARTESIAN_POINT('',(-42.5208028517601,30.0013273486611,8.11258330249199));
#7017=CARTESIAN_POINT('',(-42.5175,30.,5.));
#7018=CARTESIAN_POINT('Ctrl Pts',(-42.5208028517601,30.0013273486611,8.11258330249199));
#7019=CARTESIAN_POINT('Ctrl Pts',(-42.5212922101133,30.0778322922101,8.10772909516461));
#7020=CARTESIAN_POINT('Ctrl Pts',(-42.5181112889522,30.1542959881703,8.10287488783724));
#7021=CARTESIAN_POINT('Ctrl Pts',(-42.5111273223559,30.2304107303999,8.09802068050987));
#7022=CARTESIAN_POINT('Ctrl Pts',(-42.4349770812501,31.0603339398802,8.04509244076797));
#7023=CARTESIAN_POINT('Ctrl Pts',(-41.9066901274328,31.8487707155565,7.99216420102608));
#7024=CARTESIAN_POINT('Ctrl Pts',(-41.1680857014233,32.2348209458145,7.93923596128418));
#7025=CARTESIAN_POINT('Ctrl Pts',(-40.4294812754137,32.6208711760725,7.88630772154229));
#7026=CARTESIAN_POINT('Ctrl Pts',(-39.4805593772119,32.6045348609122,7.83337948180039));
#7027=CARTESIAN_POINT('Ctrl Pts',(-38.7556810423998,32.1932896582907,7.7804512420585));
#7028=CARTESIAN_POINT('Ctrl Pts',(-38.0308027075876,31.7820444556692,7.72752300231661));
#7029=CARTESIAN_POINT('Ctrl Pts',(-37.529967936165,30.9758903655866,7.67459476257471));
#7030=CARTESIAN_POINT('Ctrl Pts',(-37.4824297709596,30.1438378420785,7.62166652283282));
#7031=CARTESIAN_POINT('Ctrl Pts',(-37.4348916057543,29.3117853185706,7.56873828309092));
#7032=CARTESIAN_POINT('Ctrl Pts',(-37.8406500467662,28.4538343616372,7.51581004334903));
#7033=CARTESIAN_POINT('Ctrl Pts',(-38.5139724875241,27.9627048965278,7.46288180360713));
#7034=CARTESIAN_POINT('Ctrl Pts',(-39.187294928282,27.4715754314184,7.40995356386524));
#7035=CARTESIAN_POINT('Ctrl Pts',(-40.1281813687861,27.3472674581329,7.35702532412334));
#7036=CARTESIAN_POINT('Ctrl Pts',(-40.905948828007,27.6466819442195,7.30409708438145));
#7037=CARTESIAN_POINT('Ctrl Pts',(-41.683716287228,27.9460964303061,7.25116884463956));
#7038=CARTESIAN_POINT('Ctrl Pts',(-42.2983647651659,28.6692333757648,7.19824060489766));
#7039=CARTESIAN_POINT('Ctrl Pts',(-42.4685439898928,29.485082806859,7.14531236515577));
#7040=CARTESIAN_POINT('Ctrl Pts',(-42.5036217136015,29.6532475224859,7.13440267760118));
#7041=CARTESIAN_POINT('Ctrl Pts',(-42.519815547927,29.8253512559651,7.12349299004658));
#7042=CARTESIAN_POINT('Ctrl Pts',(-42.5182250179402,29.9977519260729,7.11258330249199));
#7043=CARTESIAN_POINT('Ctrl Pts',(-42.5135601364305,29.999367791574,7.38741669750801));
#7044=CARTESIAN_POINT('Ctrl Pts',(-42.5144166389034,29.6181762490351,7.41142596246836));
#7045=CARTESIAN_POINT('Ctrl Pts',(-42.4331271313634,29.2373313725707,7.43543522742871));
#7046=CARTESIAN_POINT('Ctrl Pts',(-42.2678159225957,28.8973396515338,7.45944449238906));
#7047=CARTESIAN_POINT('Ctrl Pts',(-41.9033886357073,28.1478305203288,7.51237273213095));
#7048=CARTESIAN_POINT('Ctrl Pts',(-41.1306338360994,27.5968589942747,7.56530097187285));
#7049=CARTESIAN_POINT('Ctrl Pts',(-40.303273635167,27.4966275392785,7.61822921161474));
#7050=CARTESIAN_POINT('Ctrl Pts',(-39.4759134342346,27.3963960842823,7.67115745135664));
#7051=CARTESIAN_POINT('Ctrl Pts',(-38.5939478319776,27.746904700344,7.72408569109853));
#7052=CARTESIAN_POINT('Ctrl Pts',(-38.0610893290751,28.3877113615891,7.77701393084042));
#7053=CARTESIAN_POINT('Ctrl Pts',(-37.5282308261726,29.0285180228342,7.82994217058231));
#7054=CARTESIAN_POINT('Ctrl Pts',(-37.3444794226246,29.9596227292627,7.88287041032422));
#7055=CARTESIAN_POINT('Ctrl Pts',(-37.5939457439436,30.7548191971487,7.93579865006611));
#7056=CARTESIAN_POINT('Ctrl Pts',(-37.8434120652626,31.5500156650348,7.98872688980801));
#7057=CARTESIAN_POINT('Ctrl Pts',(-38.5260961114487,32.2093038943785,8.04165512954989));
#7058=CARTESIAN_POINT('Ctrl Pts',(-39.3295050223605,32.4309017309935,8.09458336929179));
#7059=CARTESIAN_POINT('Ctrl Pts',(-40.1329139332723,32.6524995676084,8.14751160903368));
#7060=CARTESIAN_POINT('Ctrl Pts',(-41.0570477089098,32.4364070114946,8.20043984877558));
#7061=CARTESIAN_POINT('Ctrl Pts',(-41.6788915002102,31.8815354756122,8.25336808851748));
#7062=CARTESIAN_POINT('Ctrl Pts',(-42.2038620114768,31.4131040174958,8.29805095818099));
#7063=CARTESIAN_POINT('Ctrl Pts',(-42.5133902258015,30.7032245282214,8.34273382784451));
#7064=CARTESIAN_POINT('Ctrl Pts',(-42.5194677947045,29.9980220285566,8.38741669750802));
#7065=CARTESIAN_POINT('Origin',(-40.,30.,5.));
#7066=CARTESIAN_POINT('',(-42.5197815649842,30.0018165623494,9.38741669750802));
#7067=CARTESIAN_POINT('',(-42.5142224421888,30.0014129136195,9.11258330249199));
#7068=CARTESIAN_POINT('',(-42.5175,30.,5.));
#7069=CARTESIAN_POINT('',(-38.0865340033349,31.635987203375,10.));
#7070=CARTESIAN_POINT('Ctrl Pts',(-42.5197815649842,30.0018165623494,9.38741669750802));
#7071=CARTESIAN_POINT('Ctrl Pts',(-42.513858141005,29.2855376666819,9.43282641244632));
#7072=CARTESIAN_POINT('Ctrl Pts',(-42.1929705189018,28.5647530629107,9.47823612738464));
#7073=CARTESIAN_POINT('Ctrl Pts',(-41.6529744178988,28.0958628304862,9.52364584232295));
#7074=CARTESIAN_POINT('Ctrl Pts',(-41.0235707069879,27.5493380467894,9.57657408206484));
#7075=CARTESIAN_POINT('Ctrl Pts',(-40.0964959908271,27.3450257192792,9.62950232180674));
#7076=CARTESIAN_POINT('Ctrl Pts',(-39.2962220007402,27.5780866216694,9.68243056154863));
#7077=CARTESIAN_POINT('Ctrl Pts',(-38.4959480106534,27.8111475240597,9.73535880129053));
#7078=CARTESIAN_POINT('Ctrl Pts',(-37.8224747466407,28.4815816563505,9.78828704103242));
#7079=CARTESIAN_POINT('Ctrl Pts',(-37.5841061119589,29.2787069994738,9.84121528077432));
#7080=CARTESIAN_POINT('Ctrl Pts',(-37.3457374772771,30.0758323425971,9.89414352051621));
#7081=CARTESIAN_POINT('Ctrl Pts',(-37.5424734719262,30.999648896553,9.94707176025811));
#7082=CARTESIAN_POINT('Ctrl Pts',(-38.0865340033349,31.635987203375,10.));
#7083=CARTESIAN_POINT('',(-41.9171062441644,31.638757234455,9.99999999999999));
#7084=CARTESIAN_POINT('Origin',(-40.,30.,10.));
#7085=CARTESIAN_POINT('Ctrl Pts',(-41.9171091880766,31.6387594746126,9.99999999999999));
#7086=CARTESIAN_POINT('Ctrl Pts',(-41.3863009439606,32.2578634975499,9.94821753066412));
#7087=CARTESIAN_POINT('Ctrl Pts',(-40.5267000509608,32.5973561981228,9.89643506132826));
#7088=CARTESIAN_POINT('Ctrl Pts',(-39.7163628878231,32.5055165856408,9.84465259199239));
#7089=CARTESIAN_POINT('Ctrl Pts',(-38.8880957118387,32.4116448740444,9.7917243522505));
#7090=CARTESIAN_POINT('Ctrl Pts',(-38.111296463077,31.8671418326788,9.7387961125086));
#7091=CARTESIAN_POINT('Ctrl Pts',(-37.7410325214101,31.1206210243586,9.6858678727667));
#7092=CARTESIAN_POINT('Ctrl Pts',(-37.3707685797432,30.3741002160383,9.6329396330248));
#7093=CARTESIAN_POINT('Ctrl Pts',(-37.4070399451711,29.4255616407633,9.58001139328291));
#7094=CARTESIAN_POINT('Ctrl Pts',(-37.8334967847582,28.7095042189904,9.52708315354102));
#7095=CARTESIAN_POINT('Ctrl Pts',(-38.2599536243453,27.9934467972176,9.47415491379912));
#7096=CARTESIAN_POINT('Ctrl Pts',(-39.0765959380917,27.509870528947,9.42122667405723));
#7097=CARTESIAN_POINT('Ctrl Pts',(-39.9094857441256,27.4799717114424,9.36829843431534));
#7098=CARTESIAN_POINT('Ctrl Pts',(-40.7423755501596,27.4500728939378,9.31537019457344));
#7099=CARTESIAN_POINT('Ctrl Pts',(-41.5915128484811,27.8738515271992,9.26244195483155));
#7100=CARTESIAN_POINT('Ctrl Pts',(-42.0682755018096,28.5574049250838,9.20951371508965));
#7101=CARTESIAN_POINT('Ctrl Pts',(-42.3593161064952,28.9746813054093,9.1772035775571));
#7102=CARTESIAN_POINT('Ctrl Pts',(-42.5115907928592,29.4887631053692,9.14489344002455));
#7103=CARTESIAN_POINT('Ctrl Pts',(-42.5142224421888,30.0014129136195,9.11258330249199));
#7104=CARTESIAN_POINT('Origin',(-40.,-30.,5.));
#7105=CARTESIAN_POINT('',(-42.5134504848964,-29.9993943075263,0.38741669750801));
#7106=CARTESIAN_POINT('',(-42.5156173960267,-30.0035024211729,0.112583302491982));
#7107=CARTESIAN_POINT('',(-42.5175,-30.,5.));
#7108=CARTESIAN_POINT('',(-41.9134659966651,-28.364012796625,0.));
#7109=CARTESIAN_POINT('Ctrl Pts',(-42.5156173960267,-30.0035024211729,0.112583302491982));
#7110=CARTESIAN_POINT('Ctrl Pts',(-42.5103683909667,-29.4109031495499,0.0750555349946548));
#7111=CARTESIAN_POINT('Ctrl Pts',(-42.2992218280841,-28.8151964396956,0.0375277674973275));
#7112=CARTESIAN_POINT('Ctrl Pts',(-41.9134659966651,-28.364012796625,0.));
#7113=CARTESIAN_POINT('',(-38.0828936690615,-28.3612428482559,1.02151810828812E-14));
#7114=CARTESIAN_POINT('Origin',(-40.,-30.,0.));
#7115=CARTESIAN_POINT('Ctrl Pts',(-38.0828907224,-28.3612406061267,6.83481049534862E-15));
#7116=CARTESIAN_POINT('Ctrl Pts',(-38.6136989387411,-27.7421367124245,0.051782469335876));
#7117=CARTESIAN_POINT('Ctrl Pts',(-39.4732999017946,-27.4026436690207,0.103564938671745));
#7118=CARTESIAN_POINT('Ctrl Pts',(-40.283637116215,-27.4944832126233,0.155347408007614));
#7119=CARTESIAN_POINT('Ctrl Pts',(-41.1119043446168,-27.5883548538164,0.208275647749507));
#7120=CARTESIAN_POINT('Ctrl Pts',(-41.888703626185,-28.1328581109876,0.261203887491401));
#7121=CARTESIAN_POINT('Ctrl Pts',(-42.2589675775206,-28.8793789907236,0.314132127233294));
#7122=CARTESIAN_POINT('Ctrl Pts',(-42.4298570352352,-29.223923869723,0.338560317324866));
#7123=CARTESIAN_POINT('Ctrl Pts',(-42.514148869307,-29.6115012842663,0.362988507416438));
#7124=CARTESIAN_POINT('Ctrl Pts',(-42.5134504848964,-29.9993943075263,0.38741669750801));
#7125=CARTESIAN_POINT('Origin',(-40.,-30.,5.));
#7126=CARTESIAN_POINT('',(-42.517348422246,-30.0023034643409,1.38741669750801));
#7127=CARTESIAN_POINT('',(-42.5216691698492,-29.9998787127942,1.11258330249199));
#7128=CARTESIAN_POINT('',(-42.5175,-30.,5.));
#7129=CARTESIAN_POINT('Ctrl Pts',(-42.5216691698492,-29.9998787127942,1.11258330249199));
#7130=CARTESIAN_POINT('Ctrl Pts',(-42.5216727213969,-29.9941563074997,1.11221987985459));
#7131=CARTESIAN_POINT('Ctrl Pts',(-42.5216549338522,-29.9884339268551,1.11185645721719));
#7132=CARTESIAN_POINT('Ctrl Pts',(-42.5216157407844,-29.9827116948348,1.11149303457979));
#7133=CARTESIAN_POINT('Ctrl Pts',(-42.5159077306748,-29.1493357928889,1.0585647948379));
#7134=CARTESIAN_POINT('Ctrl Pts',(-42.0561778285,-28.3191122866127,1.005636555096));
#7135=CARTESIAN_POINT('Ctrl Pts',(-41.352855734795,-27.8719685956743,0.952708315354107));
#7136=CARTESIAN_POINT('Ctrl Pts',(-40.6495336410899,-27.4248249047359,0.899780075612213));
#7137=CARTESIAN_POINT('Ctrl Pts',(-39.7026193558544,-27.3607610291354,0.846851835870318));
#7138=CARTESIAN_POINT('Ctrl Pts',(-38.9455707745702,-27.709302480843,0.793923596128424));
#7139=CARTESIAN_POINT('Ctrl Pts',(-38.188522193286,-28.0578439325505,0.740995356386529));
#7140=CARTESIAN_POINT('Ctrl Pts',(-37.621339315953,-28.818990711566,0.688067116644635));
#7141=CARTESIAN_POINT('Ctrl Pts',(-37.5036141315071,-29.6439329244633,0.63513887690274));
#7142=CARTESIAN_POINT('Ctrl Pts',(-37.3858889470612,-30.4688751373606,0.582210637160846));
#7143=CARTESIAN_POINT('Ctrl Pts',(-37.7176214555024,-31.3576127841396,0.529282397418952));
#7144=CARTESIAN_POINT('Ctrl Pts',(-38.3470253385022,-31.904137509153,0.476354157677058));
#7145=CARTESIAN_POINT('Ctrl Pts',(-38.9764292215021,-32.4506622341664,0.423425917935163));
#7146=CARTESIAN_POINT('Ctrl Pts',(-39.9035044790606,-32.6549740374143,0.370497678193268));
#7147=CARTESIAN_POINT('Ctrl Pts',(-40.7037782325491,-32.4219133590322,0.317569438451373));
#7148=CARTESIAN_POINT('Ctrl Pts',(-41.5040519860376,-32.1888526806501,0.264641198709479));
#7149=CARTESIAN_POINT('Ctrl Pts',(-42.177524235456,-31.5184195206382,0.211712958967585));
#7150=CARTESIAN_POINT('Ctrl Pts',(-42.415892870965,-30.7212941263374,0.158784719225691));
#7151=CARTESIAN_POINT('Ctrl Pts',(-42.4852507331013,-30.4893554189435,0.143384246981121));
#7152=CARTESIAN_POINT('Ctrl Pts',(-42.5177714585284,-30.2466905787268,0.127983774736552));
#7153=CARTESIAN_POINT('Ctrl Pts',(-42.5156173960267,-30.0035024211729,0.112583302491982));
#7154=CARTESIAN_POINT('Ctrl Pts',(-42.5134504848964,-29.9993943075263,0.38741669750801));
#7155=CARTESIAN_POINT('Ctrl Pts',(-42.5126356889454,-30.4519440208077,0.415916747158333));
#7156=CARTESIAN_POINT('Ctrl Pts',(-42.3961357474936,-30.9049233275291,0.444416796808655));
#7157=CARTESIAN_POINT('Ctrl Pts',(-42.1665032932827,-31.2904957986896,0.472916846458978));
#7158=CARTESIAN_POINT('Ctrl Pts',(-41.7400464366065,-32.0065532246186,0.525845086200871));
#7159=CARTESIAN_POINT('Ctrl Pts',(-40.9234041021512,-32.4901295741756,0.578773325942766));
#7160=CARTESIAN_POINT('Ctrl Pts',(-40.0905142646775,-32.5200284066574,0.631701565684659));
#7161=CARTESIAN_POINT('Ctrl Pts',(-39.2576244272039,-32.5499272391393,0.684629805426554));
#7162=CARTESIAN_POINT('Ctrl Pts',(-38.4084870867119,-32.126148554546,0.737558045168449));
#7163=CARTESIAN_POINT('Ctrl Pts',(-37.9317244130836,-31.4425951218629,0.790486284910343));
#7164=CARTESIAN_POINT('Ctrl Pts',(-37.4549617394553,-30.7590416891798,0.843414524652238));
#7165=CARTESIAN_POINT('Ctrl Pts',(-37.3505737326908,-29.8157135084069,0.896342764394131));
#7166=CARTESIAN_POINT('Ctrl Pts',(-37.6663749029378,-29.0444505300205,0.949271004136026));
#7167=CARTESIAN_POINT('Ctrl Pts',(-37.9821760731849,-28.2731875516341,1.00219924387792));
#7168=CARTESIAN_POINT('Ctrl Pts',(-38.7181664204435,-27.6739897756341,1.05512748361982));
#7169=CARTESIAN_POINT('Ctrl Pts',(-39.537436538438,-27.5211153732406,1.10805572336171));
#7170=CARTESIAN_POINT('Ctrl Pts',(-40.3567066564326,-27.368240970847,1.16098396310361));
#7171=CARTESIAN_POINT('Ctrl Pts',(-41.2592565451631,-27.6616899420598,1.2139122028455));
#7172=CARTESIAN_POINT('Ctrl Pts',(-41.8319594110142,-28.2671482889205,1.26684044258739));
#7173=CARTESIAN_POINT('Ctrl Pts',(-42.2668524352508,-28.7269148226958,1.30703252756093));
#7174=CARTESIAN_POINT('Ctrl Pts',(-42.5115418566941,-29.3665990250785,1.34722461253447));
#7175=CARTESIAN_POINT('Ctrl Pts',(-42.517348422246,-30.0023034643409,1.38741669750801));
#7176=CARTESIAN_POINT('Origin',(-40.,-30.,5.));
#7177=CARTESIAN_POINT('',(-42.5213132441747,-29.9991346486057,2.38741669750801));
#7178=CARTESIAN_POINT('',(-42.5158084819528,-29.9978709045252,2.11258330249198));
#7179=CARTESIAN_POINT('',(-42.5175,-30.,5.));
#7180=CARTESIAN_POINT('Ctrl Pts',(-42.5158084819528,-29.9978709045252,2.11258330249198));
#7181=CARTESIAN_POINT('Ctrl Pts',(-42.5178587672328,-29.7423941346425,2.09645598497262));
#7182=CARTESIAN_POINT('Ctrl Pts',(-42.4820672379611,-29.4874783703648,2.08032866745326));
#7183=CARTESIAN_POINT('Ctrl Pts',(-42.4060544530648,-29.2451807415716,2.06420134993389));
#7184=CARTESIAN_POINT('Ctrl Pts',(-42.1565881113989,-28.4499842080957,2.011273110192));
#7185=CARTESIAN_POINT('Ctrl Pts',(-41.4739040096323,-27.7906959227911,1.9583448704501));
#7186=CARTESIAN_POINT('Ctrl Pts',(-40.6704950327292,-27.5690980688551,1.90541663070821));
#7187=CARTESIAN_POINT('Ctrl Pts',(-39.867086055826,-27.3475002149192,1.85248839096631));
#7188=CARTESIAN_POINT('Ctrl Pts',(-38.9429522037861,-27.5635927923519,1.79956015122442));
#7189=CARTESIAN_POINT('Ctrl Pts',(-38.321108361921,-28.1184643721705,1.74663191148252));
#7190=CARTESIAN_POINT('Ctrl Pts',(-37.6992645200558,-28.673335951989,1.69370367174063));
#7191=CARTESIAN_POINT('Ctrl Pts',(-37.3797106883653,-29.5669865341932,1.64077543199874));
#7192=CARTESIAN_POINT('Ctrl Pts',(-37.508719499589,-30.3903486277475,1.58784719225684));
#7193=CARTESIAN_POINT('Ctrl Pts',(-37.6377283108126,-31.2137107213018,1.53491895251495));
#7194=CARTESIAN_POINT('Ctrl Pts',(-38.2152997649503,-31.9667843262062,1.48199071277305));
#7195=CARTESIAN_POINT('Ctrl Pts',(-38.9770562866683,-32.3048688388086,1.42906247303116));
#7196=CARTESIAN_POINT('Ctrl Pts',(-39.7388128083864,-32.642953351411,1.37613423328926));
#7197=CARTESIAN_POINT('Ctrl Pts',(-40.6847543976847,-32.5660487717114,1.32320599354737));
#7198=CARTESIAN_POINT('Ctrl Pts',(-41.3818821333116,-32.1093323330538,1.27027775380548));
#7199=CARTESIAN_POINT('Ctrl Pts',(-42.0742231614735,-31.6557518591192,1.21771293670098));
#7200=CARTESIAN_POINT('Ctrl Pts',(-42.521155480172,-30.8275574448016,1.16514811959648));
#7201=CARTESIAN_POINT('Ctrl Pts',(-42.5216691698492,-29.9998787127942,1.11258330249199));
#7202=CARTESIAN_POINT('Ctrl Pts',(-42.517348422246,-30.0023034643409,1.38741669750801));
#7203=CARTESIAN_POINT('Ctrl Pts',(-42.5191884192899,-30.2037468612362,1.40015285227637));
#7204=CARTESIAN_POINT('Ctrl Pts',(-42.4970411605304,-30.4047906329863,1.41288900704472));
#7205=CARTESIAN_POINT('Ctrl Pts',(-42.4493576963842,-30.5995832549246,1.42562516181308));
#7206=CARTESIAN_POINT('Ctrl Pts',(-42.2511972729315,-31.4090921515597,1.47855340155497));
#7207=CARTESIAN_POINT('Ctrl Pts',(-41.6120205830545,-32.1106422223213,1.53148164129687));
#7208=CARTESIAN_POINT('Ctrl Pts',(-40.8244074737101,-32.3831071850833,1.58440988103876));
#7209=CARTESIAN_POINT('Ctrl Pts',(-40.0367943643657,-32.6555721478454,1.63733812078065));
#7210=CARTESIAN_POINT('Ctrl Pts',(-39.100744835554,-32.4989520026077,1.69026636052255));
#7211=CARTESIAN_POINT('Ctrl Pts',(-38.4447268280219,-31.9849370913482,1.74319460026444));
#7212=CARTESIAN_POINT('Ctrl Pts',(-37.7887088204899,-31.4709221800887,1.79612284000634));
#7213=CARTESIAN_POINT('Ctrl Pts',(-37.4127223342376,-30.5995125028073,1.84905107974823));
#7214=CARTESIAN_POINT('Ctrl Pts',(-37.4888725784047,-29.7695892606159,1.90197931949013));
#7215=CARTESIAN_POINT('Ctrl Pts',(-37.5650228225718,-28.9396660184245,1.95490755923202));
#7216=CARTESIAN_POINT('Ctrl Pts',(-38.0933097971584,-28.1512292113232,2.00783579897392));
#7217=CARTESIAN_POINT('Ctrl Pts',(-38.8319142523488,-27.7651789657407,2.06076403871581));
#7218=CARTESIAN_POINT('Ctrl Pts',(-39.5705187075392,-27.3791287201582,2.11369227845771));
#7219=CARTESIAN_POINT('Ctrl Pts',(-40.5194406433335,-27.3954650360944,2.1666205181996));
#7220=CARTESIAN_POINT('Ctrl Pts',(-41.2443190068267,-27.8067102550096,2.2195487579415));
#7221=CARTESIAN_POINT('Ctrl Pts',(-41.96919737032,-28.2179554739248,2.27247699768339));
#7222=CARTESIAN_POINT('Ctrl Pts',(-42.4700321615123,-29.0241095958189,2.32540523742529));
#7223=CARTESIAN_POINT('Ctrl Pts',(-42.5175703285892,-29.8561621522147,2.37833347716718));
#7224=CARTESIAN_POINT('Ctrl Pts',(-42.5202897316166,-29.9037594067979,2.38136121728079));
#7225=CARTESIAN_POINT('Ctrl Pts',(-42.5215257807612,-29.9514414106188,2.3843889573944));
#7226=CARTESIAN_POINT('Ctrl Pts',(-42.5213132441747,-29.9991346486057,2.38741669750801));
#7227=CARTESIAN_POINT('Origin',(-40.,-30.,5.));
#7228=CARTESIAN_POINT('',(-42.5147867566421,-29.9982362786167,3.38741669750801));
#7229=CARTESIAN_POINT('',(-42.5141172985733,-30.0013301677674,3.11258330249199));
#7230=CARTESIAN_POINT('',(-42.5175,-30.,5.));
#7231=CARTESIAN_POINT('Ctrl Pts',(-42.5141172985733,-30.0013301677674,3.11258330249199));
#7232=CARTESIAN_POINT('Ctrl Pts',(-42.5116926131382,-29.4952784299888,3.08069209009066));
#7233=CARTESIAN_POINT('Ctrl Pts',(-42.3636224339317,-28.9879212311263,3.04880087768933));
#7234=CARTESIAN_POINT('Ctrl Pts',(-42.0796113410677,-28.5737929421548,3.01690966528799));
#7235=CARTESIAN_POINT('Ctrl Pts',(-41.608252428045,-27.8864850691663,2.9639814255461));
#7236=CARTESIAN_POINT('Ctrl Pts',(-40.762452834543,-27.4559703537395,2.9110531858042));
#7237=CARTESIAN_POINT('Ctrl Pts',(-39.9293703365743,-27.4793133260285,2.85812494606231));
#7238=CARTESIAN_POINT('Ctrl Pts',(-39.0962878386057,-27.5026562983174,2.80519670632041));
#7239=CARTESIAN_POINT('Ctrl Pts',(-38.2759224361703,-27.979856958322,2.75226846657852));
#7240=CARTESIAN_POINT('Ctrl Pts',(-37.8437896202483,-28.6924806952517,2.69934022683663));
#7241=CARTESIAN_POINT('Ctrl Pts',(-37.4116568043264,-29.4051044321814,2.64641198709473));
#7242=CARTESIAN_POINT('Ctrl Pts',(-37.3677565749178,-30.3531512460361,2.59348374735284));
#7243=CARTESIAN_POINT('Ctrl Pts',(-37.7321838916479,-31.1026604387066,2.54055550761094));
#7244=CARTESIAN_POINT('Ctrl Pts',(-38.0966112083779,-31.8521696313771,2.48762726786905));
#7245=CARTESIAN_POINT('Ctrl Pts',(-38.8693660712466,-32.4031412028634,2.43469902812715));
#7246=CARTESIAN_POINT('Ctrl Pts',(-39.6967263399719,-32.5033726659385,2.38177078838526));
#7247=CARTESIAN_POINT('Ctrl Pts',(-40.5240866086972,-32.6036041290136,2.32884254864336));
#7248=CARTESIAN_POINT('Ctrl Pts',(-41.4060522832791,-32.2530954836775,2.27591430890147));
#7249=CARTESIAN_POINT('Ctrl Pts',(-41.9389108297875,-31.612288770186,2.22298606915957));
#7250=CARTESIAN_POINT('Ctrl Pts',(-42.3094065428755,-31.1667368656095,2.18618514693704));
#7251=CARTESIAN_POINT('Ctrl Pts',(-42.5111299364331,-30.5808432882975,2.14938422471451));
#7252=CARTESIAN_POINT('Ctrl Pts',(-42.5158084819528,-29.9978709045252,2.11258330249198));
#7253=CARTESIAN_POINT('Ctrl Pts',(-42.5213132441747,-29.9991346486057,2.38741669750801));
#7254=CARTESIAN_POINT('Ctrl Pts',(-42.5178104065942,-30.7851718628753,2.43731719713629));
#7255=CARTESIAN_POINT('Ctrl Pts',(-42.1208328792847,-31.5742605775652,2.48721769676458));
#7256=CARTESIAN_POINT('Ctrl Pts',(-41.4860275712473,-32.0372951840482,2.53711819639286));
#7257=CARTESIAN_POINT('Ctrl Pts',(-40.8127051038668,-32.5284246685882,2.59004643613476));
#7258=CARTESIAN_POINT('Ctrl Pts',(-39.8718186261444,-32.6527326467706,2.64297467587665));
#7259=CARTESIAN_POINT('Ctrl Pts',(-39.0940511361637,-32.3533181488389,2.69590291561855));
#7260=CARTESIAN_POINT('Ctrl Pts',(-38.3162836461829,-32.0539036509073,2.74883115536044));
#7261=CARTESIAN_POINT('Ctrl Pts',(-37.7016351439439,-31.3307666768615,2.80175939510233));
#7262=CARTESIAN_POINT('Ctrl Pts',(-37.5314559124885,-30.5149172135064,2.85468763484423));
#7263=CARTESIAN_POINT('Ctrl Pts',(-37.361276681033,-29.6990677501512,2.90761587458612));
#7264=CARTESIAN_POINT('Ctrl Pts',(-37.6355667203612,-28.7905057974866,2.96054411432802));
#7265=CARTESIAN_POINT('Ctrl Pts',(-38.2287720265447,-28.2051180801097,3.01347235406991));
#7266=CARTESIAN_POINT('Ctrl Pts',(-38.8219773327282,-27.6197303627328,3.06640059381181));
#7267=CARTESIAN_POINT('Ctrl Pts',(-39.7340979057671,-27.3575168806436,3.1193288335537));
#7268=CARTESIAN_POINT('Ctrl Pts',(-40.5476180890752,-27.5385036919369,3.1722570732956));
#7269=CARTESIAN_POINT('Ctrl Pts',(-41.3611382723834,-27.7194905032302,3.22518531303749));
#7270=CARTESIAN_POINT('Ctrl Pts',(-42.0760580659608,-28.3436776079059,3.27811355277939));
#7271=CARTESIAN_POINT('Ctrl Pts',(-42.3651288382537,-29.1253485131059,3.33104179252128));
#7272=CARTESIAN_POINT('Ctrl Pts',(-42.4677604856938,-29.4028728443289,3.34983342751686));
#7273=CARTESIAN_POINT('Ctrl Pts',(-42.5167124568098,-29.7002485290033,3.36862506251243));
#7274=CARTESIAN_POINT('Ctrl Pts',(-42.5147867566421,-29.9982362786167,3.38741669750801));
#7275=CARTESIAN_POINT('Origin',(-40.,-30.,5.));
#7276=CARTESIAN_POINT('',(-42.5149325414735,-30.0018328375922,4.38741669750801));
#7277=CARTESIAN_POINT('',(-42.5206616850174,-30.0014234824409,4.11258330249199));
#7278=CARTESIAN_POINT('',(-42.5175,-30.,5.));
#7279=CARTESIAN_POINT('Ctrl Pts',(-42.5206616850174,-30.0014234824409,4.11258330249199));
#7280=CARTESIAN_POINT('Ctrl Pts',(-42.5155795866941,-29.2502422402753,4.06492819520869));
#7281=CARTESIAN_POINT('Ctrl Pts',(-42.1578863186577,-28.4948606212539,4.01727308792539));
#7282=CARTESIAN_POINT('Ctrl Pts',(-41.5708988488514,-28.0274060986095,3.9696179806421));
#7283=CARTESIAN_POINT('Ctrl Pts',(-40.9189600473564,-27.5082268027603,3.9166897409002));
#7284=CARTESIAN_POINT('Ctrl Pts',(-39.9841758778376,-27.3442193556112,3.8637615011583));
#7285=CARTESIAN_POINT('Ctrl Pts',(-39.1944360729249,-27.6104568110664,3.81083326141641));
#7286=CARTESIAN_POINT('Ctrl Pts',(-38.4046962680121,-27.8766942665217,3.75790502167452));
#7287=CARTESIAN_POINT('Ctrl Pts',(-37.7600008277053,-28.5731766245815,3.70497678193262));
#7288=CARTESIAN_POINT('Ctrl Pts',(-37.5554537649444,-29.38109483929,3.65204854219073));
#7289=CARTESIAN_POINT('Ctrl Pts',(-37.3509067021835,-30.1890130539986,3.59912030244883));
#7290=CARTESIAN_POINT('Ctrl Pts',(-37.5865080169685,-31.1083671253559,3.54619206270694));
#7291=CARTESIAN_POINT('Ctrl Pts',(-38.1544131533048,-31.7183303191202,3.49326382296504));
#7292=CARTESIAN_POINT('Ctrl Pts',(-38.7223182896412,-32.3282935128845,3.44033558322315));
#7293=CARTESIAN_POINT('Ctrl Pts',(-39.6225272475288,-32.6288658290557,3.38740734348126));
#7294=CARTESIAN_POINT('Ctrl Pts',(-40.4429768120994,-32.4824627756441,3.33447910373936));
#7295=CARTESIAN_POINT('Ctrl Pts',(-41.26342637667,-32.3360597222325,3.28155086399747));
#7296=CARTESIAN_POINT('Ctrl Pts',(-42.0041165479235,-31.742681299238,3.22862262425557));
#7297=CARTESIAN_POINT('Ctrl Pts',(-42.3260025172786,-30.9739415724657,3.17569438451368));
#7298=CARTESIAN_POINT('Ctrl Pts',(-42.4539403434918,-30.6683958235659,3.15465735717311));
#7299=CARTESIAN_POINT('Ctrl Pts',(-42.5157167414903,-30.3351470233143,3.13362032983255));
#7300=CARTESIAN_POINT('Ctrl Pts',(-42.5141172985733,-30.0013301677674,3.11258330249199));
#7301=CARTESIAN_POINT('Ctrl Pts',(-42.5147867566421,-29.9982362786167,3.38741669750801));
#7302=CARTESIAN_POINT('Ctrl Pts',(-42.511288558348,-30.5395563941995,3.42155330225433));
#7303=CARTESIAN_POINT('Ctrl Pts',(-42.339894983855,-31.0828963127842,3.45568990700064));
#7304=CARTESIAN_POINT('Ctrl Pts',(-42.0174032055179,-31.5129223213822,3.48982651174696));
#7305=CARTESIAN_POINT('Ctrl Pts',(-41.5173850494808,-32.1796705187342,3.54275475148886));
#7306=CARTESIAN_POINT('Ctrl Pts',(-40.6541269863983,-32.5740122077138,3.59568299123075));
#7307=CARTESIAN_POINT('Ctrl Pts',(-39.8227782642378,-32.5154407369856,3.64861123097265));
#7308=CARTESIAN_POINT('Ctrl Pts',(-38.9914295420773,-32.4568692662574,3.70153947071454));
#7309=CARTESIAN_POINT('Ctrl Pts',(-38.1919901608389,-31.9453846358214,3.75446771045644));
#7310=CARTESIAN_POINT('Ctrl Pts',(-37.7903968943648,-31.2151147107584,3.80739595019833));
#7311=CARTESIAN_POINT('Ctrl Pts',(-37.3888036278907,-30.4848447856954,3.86032418994022));
#7312=CARTESIAN_POINT('Ctrl Pts',(-37.3850564761809,-29.5357895660055,3.91325242968212));
#7313=CARTESIAN_POINT('Ctrl Pts',(-37.7808706669184,-28.8023712396148,3.96618066942401));
#7314=CARTESIAN_POINT('Ctrl Pts',(-38.1766848576559,-28.0689529132242,4.01910890916591));
#7315=CARTESIAN_POINT('Ctrl Pts',(-38.9720603908406,-27.5511714801328,4.0720371489078));
#7316=CARTESIAN_POINT('Ctrl Pts',(-39.8029206856667,-27.486037114713,4.1249653886497));
#7317=CARTESIAN_POINT('Ctrl Pts',(-40.6337809804928,-27.4209027492932,4.17789362839159));
#7318=CARTESIAN_POINT('Ctrl Pts',(-41.5001260369602,-27.8084154515449,4.23082186813349));
#7319=CARTESIAN_POINT('Ctrl Pts',(-42.005393561113,-28.4711944826902,4.28375010787538));
#7320=CARTESIAN_POINT('Ctrl Pts',(-42.3352701470746,-28.9039064097189,4.31830563775292));
#7321=CARTESIAN_POINT('Ctrl Pts',(-42.5112389161138,-29.45394948023,4.35286116763047));
#7322=CARTESIAN_POINT('Ctrl Pts',(-42.5149325414735,-30.0018328375922,4.38741669750801));
#7323=CARTESIAN_POINT('Origin',(-40.,-30.,5.));
#7324=CARTESIAN_POINT('',(-42.521402710782,-30.0007512051302,5.38741669750801));
#7325=CARTESIAN_POINT('',(-42.5184257094164,-29.9977798166958,5.11258330249199));
#7326=CARTESIAN_POINT('',(-42.5175,-30.,5.));
#7327=CARTESIAN_POINT('Ctrl Pts',(-42.5184257094164,-29.9977798166958,5.11258330249199));
#7328=CARTESIAN_POINT('Ctrl Pts',(-42.5199490958157,-29.8320331685022,5.10209254006862));
#7329=CARTESIAN_POINT('Ctrl Pts',(-42.50498599437,-29.666560233277,5.09160177764525));
#7330=CARTESIAN_POINT('Ctrl Pts',(-42.4725332000196,-29.504591615208,5.08111101522188));
#7331=CARTESIAN_POINT('Ctrl Pts',(-42.3088016035587,-28.6874237582064,5.02818277547999));
#7332=CARTESIAN_POINT('Ctrl Pts',(-41.6998824869394,-27.9594557672715,4.97525453573809));
#7333=CARTESIAN_POINT('Ctrl Pts',(-40.9245035463699,-27.6539089775381,4.9223262959962));
#7334=CARTESIAN_POINT('Ctrl Pts',(-40.1491246058004,-27.3483621878047,4.8693980562543));
#7335=CARTESIAN_POINT('Ctrl Pts',(-39.2072858412808,-27.4652365992728,4.81646981651241));
#7336=CARTESIAN_POINT('Ctrl Pts',(-38.5301061680647,-27.9510339154214,4.76354157677051));
#7337=CARTESIAN_POINT('Ctrl Pts',(-37.8529264948486,-28.4368312315701,4.71061333702862));
#7338=CARTESIAN_POINT('Ctrl Pts',(-37.440405912936,-29.2915514523993,4.65768509728673));
#7339=CARTESIAN_POINT('Ctrl Pts',(-37.4813723114462,-30.1239534564781,4.60475685754483));
#7340=CARTESIAN_POINT('Ctrl Pts',(-37.5223387099564,-30.956355460557,4.55182861780294));
#7341=CARTESIAN_POINT('Ctrl Pts',(-38.0167920888894,-31.7664392478856,4.49890037806104));
#7342=CARTESIAN_POINT('Ctrl Pts',(-38.7384004980203,-32.1833956557518,4.44597213831915));
#7343=CARTESIAN_POINT('Ctrl Pts',(-39.4600089071513,-32.600352063618,4.39304389857725));
#7344=CARTESIAN_POINT('Ctrl Pts',(-40.4087723464802,-32.6241810920218,4.34011565883536));
#7345=CARTESIAN_POINT('Ctrl Pts',(-41.1504021880581,-32.2439752000789,4.28718741909346));
#7346=CARTESIAN_POINT('Ctrl Pts',(-41.8920320296359,-31.863769308136,4.23425917935157));
#7347=CARTESIAN_POINT('Ctrl Pts',(-42.4265282734626,-31.0795284958463,4.18133093960967));
#7348=CARTESIAN_POINT('Ctrl Pts',(-42.5092296786403,-30.250232517427,4.12840269986778));
#7349=CARTESIAN_POINT('Ctrl Pts',(-42.5174690507815,-30.1676114523224,4.12312956740918));
#7350=CARTESIAN_POINT('Ctrl Pts',(-42.5212240293106,-30.0845431818009,4.11785643495058));
#7351=CARTESIAN_POINT('Ctrl Pts',(-42.5206616850174,-30.0014234824409,4.11258330249199));
#7352=CARTESIAN_POINT('Ctrl Pts',(-42.5149325414735,-30.0018328375922,4.38741669750801));
#7353=CARTESIAN_POINT('Ctrl Pts',(-42.516896392334,-30.2931350401628,4.40578940737236));
#7354=CARTESIAN_POINT('Ctrl Pts',(-42.4701596848035,-30.5838267121945,4.42416211723671));
#7355=CARTESIAN_POINT('Ctrl Pts',(-42.3719617588218,-30.8559480471321,4.44253482710106));
#7356=CARTESIAN_POINT('Ctrl Pts',(-42.0890724405397,-31.6398772203896,4.49546306684296));
#7357=CARTESIAN_POINT('Ctrl Pts',(-41.3791038121377,-32.2696902068656,4.54839130658486));
#7358=CARTESIAN_POINT('Ctrl Pts',(-40.5670381492107,-32.4570953139945,4.60131954632675));
#7359=CARTESIAN_POINT('Ctrl Pts',(-39.7549724862838,-32.6445004211234,4.65424778606864));
#7360=CARTESIAN_POINT('Ctrl Pts',(-38.840809788832,-32.3894976489052,4.70717602581054));
#7361=CARTESIAN_POINT('Ctrl Pts',(-38.243000481004,-31.8088124101068,4.76010426555243));
#7362=CARTESIAN_POINT('Ctrl Pts',(-37.645191173176,-31.2281271713084,4.81303250529432));
#7363=CARTESIAN_POINT('Ctrl Pts',(-37.3637352549718,-30.3217594659298,4.86596074503622));
#7364=CARTESIAN_POINT('Ctrl Pts',(-37.5274668482371,-29.504591624877,4.91888898477811));
#7365=CARTESIAN_POINT('Ctrl Pts',(-37.6911984415025,-28.6874237838241,4.97181722452001));
#7366=CARTESIAN_POINT('Ctrl Pts',(-38.3001175462374,-27.959455807097,5.0247454642619));
#7367=CARTESIAN_POINT('Ctrl Pts',(-39.0754964716737,-27.653909023327,5.0776737040038));
#7368=CARTESIAN_POINT('Ctrl Pts',(-39.85087539711,-27.348362239557,5.1306019437457));
#7369=CARTESIAN_POINT('Ctrl Pts',(-40.7927141432477,-27.465236648744,5.18353018348759));
#7370=CARTESIAN_POINT('Ctrl Pts',(-41.4698938032473,-27.9510339554113,5.23645842322948));
#7371=CARTESIAN_POINT('Ctrl Pts',(-42.1136955075206,-28.4128864776267,5.28677784798899));
#7372=CARTESIAN_POINT('Ctrl Pts',(-42.5182850573256,-29.2081900157384,5.3370972727485));
#7373=CARTESIAN_POINT('Ctrl Pts',(-42.521402710782,-30.0007512051302,5.38741669750801));
#7374=CARTESIAN_POINT('Origin',(-40.,-30.,5.));
#7375=CARTESIAN_POINT('',(-42.5171494503087,-29.9976988316789,6.38741669750801));
#7376=CARTESIAN_POINT('',(-42.5134147285392,-29.9999453848359,6.11258330249199));
#7377=CARTESIAN_POINT('',(-42.5175,-30.,5.));
#7378=CARTESIAN_POINT('Ctrl Pts',(-42.5134147285392,-29.9999453848359,6.11258330249199));
#7379=CARTESIAN_POINT('Ctrl Pts',(-42.5134953811471,-29.5830437993479,6.08632864518665));
#7380=CARTESIAN_POINT('Ctrl Pts',(-42.4154700479868,-29.1661778965789,6.06007398788132));
#7381=CARTESIAN_POINT('Ctrl Pts',(-42.2191293763926,-28.8023712162405,6.03381933057598));
#7382=CARTESIAN_POINT('Ctrl Pts',(-41.82331517793,-28.0689528755357,5.98089109083409));
#7383=CARTESIAN_POINT('Ctrl Pts',(-41.0279396292218,-27.5511714323388,5.92796285109219));
#7384=CARTESIAN_POINT('Ctrl Pts',(-40.1970793181797,-27.4860370656477,5.8750346113503));
#7385=CARTESIAN_POINT('Ctrl Pts',(-39.3662190071376,-27.4209026989567,5.8221063716084));
#7386=CARTESIAN_POINT('Ctrl Pts',(-38.4998739337617,-27.8084154087715,5.76917813186651));
#7387=CARTESIAN_POINT('Ctrl Pts',(-37.9946063997475,-28.4711944528524,5.71624989212461));
#7388=CARTESIAN_POINT('Ctrl Pts',(-37.4893388657334,-29.1339734969332,5.66332165238272));
#7389=CARTESIAN_POINT('Ctrl Pts',(-37.3451488710812,-30.0720188752802,5.61039341264082));
#7390=CARTESIAN_POINT('Ctrl Pts',(-37.6280381948844,-30.8559480638377,5.55746517289893));
#7391=CARTESIAN_POINT('Ctrl Pts',(-37.9109275186876,-31.6398772523952,5.50453693315704));
#7392=CARTESIAN_POINT('Ctrl Pts',(-38.6208961609462,-32.2696902511634,5.45160869341514));
#7393=CARTESIAN_POINT('Ctrl Pts',(-39.4329618397223,-32.4570953619499,5.39868045367325));
#7394=CARTESIAN_POINT('Ctrl Pts',(-40.2450275184985,-32.6445004727364,5.34575221393135));
#7395=CARTESIAN_POINT('Ctrl Pts',(-41.1591902337921,-32.3894976955413,5.29282397418946));
#7396=CARTESIAN_POINT('Ctrl Pts',(-41.7569995532876,-31.8088124454096,5.23989573444756));
#7397=CARTESIAN_POINT('Ctrl Pts',(-42.2363187137321,-31.3432232391213,5.19745825712904));
#7398=CARTESIAN_POINT('Ctrl Pts',(-42.5122632711536,-30.6682620313788,5.15502077981051));
#7399=CARTESIAN_POINT('Ctrl Pts',(-42.5184257094164,-29.9977798166958,5.11258330249199));
#7400=CARTESIAN_POINT('Ctrl Pts',(-42.521402710782,-30.0007512051302,5.38741669750801));
#7401=CARTESIAN_POINT('Ctrl Pts',(-42.5215643457984,-30.041841609387,5.39002551249039));
#7402=CARTESIAN_POINT('Ctrl Pts',(-42.5206468592439,-30.0829246424488,5.39263432747278));
#7403=CARTESIAN_POINT('Ctrl Pts',(-42.5186276393975,-30.1239534540589,5.39524314245516));
#7404=CARTESIAN_POINT('Ctrl Pts',(-42.4776612416868,-30.9563554418917,5.44817138219706));
#7405=CARTESIAN_POINT('Ctrl Pts',(-41.9832078724042,-31.7664392134098,5.50109962193896));
#7406=CARTESIAN_POINT('Ctrl Pts',(-41.2615994773569,-32.1833956131383,5.55402786168085));
#7407=CARTESIAN_POINT('Ctrl Pts',(-40.5399910823097,-32.6003520128667,5.60695610142275));
#7408=CARTESIAN_POINT('Ctrl Pts',(-39.5912276614978,-32.6241810408054,5.65988434116464));
#7409=CARTESIAN_POINT('Ctrl Pts',(-38.8495978343945,-32.243975156283,5.71281258090653));
#7410=CARTESIAN_POINT('Ctrl Pts',(-38.1079680072911,-31.8637692717606,5.76574082064843));
#7411=CARTESIAN_POINT('Ctrl Pts',(-37.5734717738962,-31.0795284747771,5.81866906039032));
#7412=CARTESIAN_POINT('Ctrl Pts',(-37.4907703703327,-30.2502325125432,5.87159730013222));
#7413=CARTESIAN_POINT('Ctrl Pts',(-37.4080689667691,-29.4209365503093,5.92452553987411));
#7414=CARTESIAN_POINT('Ctrl Pts',(-37.7771623930368,-28.546585422825,5.97745377961601));
#7415=CARTESIAN_POINT('Ctrl Pts',(-38.429101181808,-28.0274061371088,6.0303820193579));
#7416=CARTESIAN_POINT('Ctrl Pts',(-39.0810399705791,-27.5082268513926,6.08331025909979));
#7417=CARTESIAN_POINT('Ctrl Pts',(-40.0158241218535,-27.3442194074445,6.13623849884169));
#7418=CARTESIAN_POINT('Ctrl Pts',(-40.8055639113529,-27.6104568577035,6.18916673858358));
#7419=CARTESIAN_POINT('Ctrl Pts',(-41.5953037008522,-27.8766943079625,6.24209497832548));
#7420=CARTESIAN_POINT('Ctrl Pts',(-42.2399991285764,-28.5731766524286,6.29502321806738));
#7421=CARTESIAN_POINT('Ctrl Pts',(-42.4445461873451,-29.3810948513691,6.34795145780927));
#7422=CARTESIAN_POINT('Ctrl Pts',(-42.495385454142,-29.5818993464971,6.36110653770885));
#7423=CARTESIAN_POINT('Ctrl Pts',(-42.5190345977134,-29.7895877808343,6.37426161760843));
#7424=CARTESIAN_POINT('Ctrl Pts',(-42.5171494503087,-29.9976988316789,6.38741669750801));
#7425=CARTESIAN_POINT('Origin',(-40.,-30.,5.));
#7426=CARTESIAN_POINT('',(-42.5135602932616,-30.0006322084125,7.38741669750801));
#7427=CARTESIAN_POINT('',(-42.5182251666708,-30.0022480740648,7.11258330249199));
#7428=CARTESIAN_POINT('',(-42.5175,-30.,5.));
#7429=CARTESIAN_POINT('Ctrl Pts',(-42.5182251666708,-30.0022480740648,7.11258330249199));
#7430=CARTESIAN_POINT('Ctrl Pts',(-42.5120992560187,-29.3382485831854,7.07056475030469));
#7431=CARTESIAN_POINT('Ctrl Pts',(-42.2421605144463,-28.6698443415211,7.02854619811738));
#7432=CARTESIAN_POINT('Ctrl Pts',(-41.771228008025,-28.2051180450781,6.98652764593008));
#7433=CARTESIAN_POINT('Ctrl Pts',(-41.1780226902642,-27.6197303162755,6.93359940618819));
#7434=CARTESIAN_POINT('Ctrl Pts',(-40.2659020994226,-27.35751682907,6.88067116644629));
#7435=CARTESIAN_POINT('Ctrl Pts',(-39.4523819002367,-27.538503643896,6.8277429267044));
#7436=CARTESIAN_POINT('Ctrl Pts',(-38.6388617010508,-27.7194904587219,6.77481468696251));
#7437=CARTESIAN_POINT('Ctrl Pts',(-37.9239418935206,-28.3436775755792,6.72188644722061));
#7438=CARTESIAN_POINT('Ctrl Pts',(-37.6348711155859,-29.125348496035,6.66895820747872));
#7439=CARTESIAN_POINT('Ctrl Pts',(-37.3458003376513,-29.9070194164908,6.61602996773682));
#7440=CARTESIAN_POINT('Ctrl Pts',(-37.4825785893123,-30.8461741405451,6.56310172799493));
#7441=CARTESIAN_POINT('Ctrl Pts',(-37.9825967551082,-31.5129223509102,6.51017348825303));
#7442=CARTESIAN_POINT('Ctrl Pts',(-38.4826149209041,-32.1796705612752,6.45724524851114));
#7443=CARTESIAN_POINT('Ctrl Pts',(-39.345873000835,-32.5740122579511,6.40431700876924));
#7444=CARTESIAN_POINT('Ctrl Pts',(-40.1772217392211,-32.5154407860797,6.35138876902735));
#7445=CARTESIAN_POINT('Ctrl Pts',(-41.0085704776071,-32.4568693142083,6.29846052928545));
#7446=CARTESIAN_POINT('Ctrl Pts',(-41.8080098744483,-31.9453846737896,6.24553228954356));
#7447=CARTESIAN_POINT('Ctrl Pts',(-42.2096031487603,-31.2151147344739,6.19260404980166));
#7448=CARTESIAN_POINT('Ctrl Pts',(-42.4119890841431,-30.8470897345444,6.16593046736511));
#7449=CARTESIAN_POINT('Ctrl Pts',(-42.5133327890205,-30.4234991444269,6.13925688492855));
#7450=CARTESIAN_POINT('Ctrl Pts',(-42.5134147285392,-29.9999453848359,6.11258330249199));
#7451=CARTESIAN_POINT('Ctrl Pts',(-42.5171494503087,-29.9976988316789,6.38741669750801));
#7452=CARTESIAN_POINT('Ctrl Pts',(-42.5114498825654,-30.6269032267395,6.42718985735033));
#7453=CARTESIAN_POINT('Ctrl Pts',(-42.2723416287469,-31.2599707548622,6.46696301719264));
#7454=CARTESIAN_POINT('Ctrl Pts',(-41.8455868106747,-31.7183302855837,6.50673617703495));
#7455=CARTESIAN_POINT('Ctrl Pts',(-41.2776816854222,-32.3282934674429,6.55966441677685));
#7456=CARTESIAN_POINT('Ctrl Pts',(-40.3774727451039,-32.6288657777464,6.61259265651874));
#7457=CARTESIAN_POINT('Ctrl Pts',(-39.5570231965462,-32.4824627271928,6.66552089626064));
#7458=CARTESIAN_POINT('Ctrl Pts',(-38.7365736479884,-32.3360596766392,6.71844913600253));
#7459=CARTESIAN_POINT('Ctrl Pts',(-37.9958834911912,-31.7426812652287,6.77137737574443));
#7460=CARTESIAN_POINT('Ctrl Pts',(-37.6739975281183,-30.9739415534587,6.82430561548632));
#7461=CARTESIAN_POINT('Ctrl Pts',(-37.3521115650454,-30.2052018416886,6.87723385522821));
#7462=CARTESIAN_POINT('Ctrl Pts',(-37.4490297956967,-29.261100829559,6.9301620949701));
#7463=CARTESIAN_POINT('Ctrl Pts',(-37.9203886995201,-28.5737929699874,6.983090334712));
#7464=CARTESIAN_POINT('Ctrl Pts',(-38.3917476033435,-27.8864851104157,7.0360185744539));
#7465=CARTESIAN_POINT('Ctrl Pts',(-39.237547180339,-27.4559704034018,7.08894681419579));
#7466=CARTESIAN_POINT('Ctrl Pts',(-40.0706296620477,-27.4793133752305,7.14187505393769));
#7467=CARTESIAN_POINT('Ctrl Pts',(-40.9037121437564,-27.5026563470591,7.19480329367958));
#7468=CARTESIAN_POINT('Ctrl Pts',(-41.7240775301785,-27.9798569977301,7.24773153342147));
#7469=CARTESIAN_POINT('Ctrl Pts',(-42.1562103376676,-28.6924807207603,7.30065977316337));
#7470=CARTESIAN_POINT('Ctrl Pts',(-42.392319413333,-29.0818446515379,7.32957874794491));
#7471=CARTESIAN_POINT('Ctrl Pts',(-42.5125286425665,-29.5414899018482,7.35849772272646));
#7472=CARTESIAN_POINT('Ctrl Pts',(-42.5135602932616,-30.0006322084125,7.38741669750801));
#7473=CARTESIAN_POINT('Origin',(-40.,-30.,5.));
#7474=CARTESIAN_POINT('',(-42.51946795121,-30.0019779683886,8.38741669750802));
#7475=CARTESIAN_POINT('',(-42.5208030005754,-29.9986726513939,8.11258330249199));
#7476=CARTESIAN_POINT('',(-42.5175,-30.,5.));
#7477=CARTESIAN_POINT('Ctrl Pts',(-42.5208030005754,-29.9986726513939,8.11258330249199));
#7478=CARTESIAN_POINT('Ctrl Pts',(-42.5212923589469,-29.922167703349,8.10772909516461));
#7479=CARTESIAN_POINT('Ctrl Pts',(-42.5181114375889,-29.8457040028919,8.10287488783724));
#7480=CARTESIAN_POINT('Ctrl Pts',(-42.5111274705733,-29.7695892561818,8.09802068050987));
#7481=CARTESIAN_POINT('Ctrl Pts',(-42.4349772248954,-28.9396659978463,8.04509244076797));
#7482=CARTESIAN_POINT('Ctrl Pts',(-41.9066902400584,-28.151229175236,7.99216420102608));
#7483=CARTESIAN_POINT('Ctrl Pts',(-41.1680857704662,-27.7651789220903,7.93923596128419));
#7484=CARTESIAN_POINT('Ctrl Pts',(-40.4294813008741,-27.3791286689446,7.88630772154229));
#7485=CARTESIAN_POINT('Ctrl Pts',(-39.4805593465267,-27.3954649852637,7.83337948180039));
#7486=CARTESIAN_POINT('Ctrl Pts',(-38.7556809688784,-27.8067102122203,7.7804512420585));
#7487=CARTESIAN_POINT('Ctrl Pts',(-38.0308025912301,-28.217955439177,7.7275230023166));
#7488=CARTESIAN_POINT('Ctrl Pts',(-37.5299677902808,-29.0241095767712,7.67459476257471));
#7489=CARTESIAN_POINT('Ctrl Pts',(-37.4824296222801,-29.8561621493983,7.62166652283282));
#7490=CARTESIAN_POINT('Ctrl Pts',(-37.4348914542795,-30.6882147220254,7.56873828309093));
#7491=CARTESIAN_POINT('Ctrl Pts',(-37.8406499192275,-31.5461657296854,7.51581004334903));
#7492=CARTESIAN_POINT('Ctrl Pts',(-38.513972399747,-32.0372952238151,7.46288180360714));
#7493=CARTESIAN_POINT('Ctrl Pts',(-39.1872948802665,-32.5284247179447,7.40995356386524));
#7494=CARTESIAN_POINT('Ctrl Pts',(-40.1281813763575,-32.652732698544,7.35702532412334));
#7495=CARTESIAN_POINT('Ctrl Pts',(-40.9059488815193,-32.3533181947664,7.30409708438145));
#7496=CARTESIAN_POINT('Ctrl Pts',(-41.683716386681,-32.0539036909888,7.25116884463955));
#7497=CARTESIAN_POINT('Ctrl Pts',(-42.2983649009134,-31.3307667028344,7.19824060489766));
#7498=CARTESIAN_POINT('Ctrl Pts',(-42.4685441356896,-30.5149172235574,7.14531236515577));
#7499=CARTESIAN_POINT('Ctrl Pts',(-42.5036218614697,-30.3467524979989,7.13440267760118));
#7500=CARTESIAN_POINT('Ctrl Pts',(-42.5198156967515,-30.174648754355,7.12349299004658));
#7501=CARTESIAN_POINT('Ctrl Pts',(-42.5182251666708,-30.0022480740648,7.11258330249199));
#7502=CARTESIAN_POINT('Ctrl Pts',(-42.5135602932616,-30.0006322084125,7.38741669750801));
#7503=CARTESIAN_POINT('Ctrl Pts',(-42.5144167957854,-30.3818237747137,7.41142596246836));
#7504=CARTESIAN_POINT('Ctrl Pts',(-42.4331272831723,-30.76266867493,7.43543522742871));
#7505=CARTESIAN_POINT('Ctrl Pts',(-42.2678160640931,-31.1026604172056,7.45944449238905));
#7506=CARTESIAN_POINT('Ctrl Pts',(-41.9033887544732,-31.8521695952311,7.51237273213095));
#7507=CARTESIAN_POINT('Ctrl Pts',(-41.1306339066773,-32.4031411558927,7.56530097187284));
#7508=CARTESIAN_POINT('Ctrl Pts',(-40.3032736541046,-32.5033726170428,7.61822921161474));
#7509=CARTESIAN_POINT('Ctrl Pts',(-39.4759134015319,-32.6036040781929,7.67115745135663));
#7510=CARTESIAN_POINT('Ctrl Pts',(-38.5939477441824,-32.2530954398316,7.72408569109853));
#7511=CARTESIAN_POINT('Ctrl Pts',(-38.0610892080637,-31.6122887387886,7.77701393084043));
#7512=CARTESIAN_POINT('Ctrl Pts',(-37.5282306719451,-30.9714820377456,7.82994217058232));
#7513=CARTESIAN_POINT('Ctrl Pts',(-37.3444792570573,-30.0403772740209,7.88287041032421));
#7514=CARTESIAN_POINT('Ctrl Pts',(-37.5939455938752,-29.2451807561725,7.93579865006611));
#7515=CARTESIAN_POINT('Ctrl Pts',(-37.8434119306932,-28.4499842383242,7.988726889808));
#7516=CARTESIAN_POINT('Ctrl Pts',(-38.5260960192167,-27.7906959663523,8.04165512954989));
#7517=CARTESIAN_POINT('Ctrl Pts',(-39.3295049803966,-27.5690981165436,8.09458336929179));
#7518=CARTESIAN_POINT('Ctrl Pts',(-40.1329139415765,-27.3475002667349,8.14751160903368));
#7519=CARTESIAN_POINT('Ctrl Pts',(-41.0570477754128,-27.5635928390895,8.20043984877558));
#7520=CARTESIAN_POINT('Ctrl Pts',(-41.67889160523,-28.1184644084391,8.25336808851747));
#7521=CARTESIAN_POINT('Ctrl Pts',(-42.2038621490131,-28.586895894809,8.29805095818099));
#7522=CARTESIAN_POINT('Ctrl Pts',(-42.513390381827,-29.2967754246142,8.3427338278445));
#7523=CARTESIAN_POINT('Ctrl Pts',(-42.51946795121,-30.0019779683886,8.38741669750802));
#7524=CARTESIAN_POINT('Origin',(-40.,-30.,5.));
#7525=CARTESIAN_POINT('',(-42.5197817068771,-29.9981833838556,9.38741669750801));
#7526=CARTESIAN_POINT('',(-42.5142225916618,-29.9985870806183,9.11258330249199));
#7527=CARTESIAN_POINT('',(-42.5175,-30.,5.));
#7528=CARTESIAN_POINT('',(-38.0865340033349,-28.364012796625,10.));
#7529=CARTESIAN_POINT('Ctrl Pts',(-42.5197817068771,-29.9981833838556,9.38741669750801));
#7530=CARTESIAN_POINT('Ctrl Pts',(-42.5138583444366,-30.7144624076937,9.43282641244632));
#7531=CARTESIAN_POINT('Ctrl Pts',(-42.1929708169802,-31.4352472342186,9.47823612738463));
#7532=CARTESIAN_POINT('Ctrl Pts',(-41.6529746034879,-31.9041374282717,9.52364584232294));
#7533=CARTESIAN_POINT('Ctrl Pts',(-41.0235707614628,-32.450662167244,9.57657408206484));
#7534=CARTESIAN_POINT('Ctrl Pts',(-40.096495632782,-32.654974095277,9.62950232180673));
#7535=CARTESIAN_POINT('Ctrl Pts',(-39.2962218229396,-32.4219133635354,9.68243056154862));
#7536=CARTESIAN_POINT('Ctrl Pts',(-38.4959480130971,-32.1888526317938,9.73535880129052));
#7537=CARTESIAN_POINT('Ctrl Pts',(-37.8224755220932,-31.5184192402776,9.78828704103242));
#7538=CARTESIAN_POINT('Ctrl Pts',(-37.5841068868004,-30.7212938581909,9.84121528077432));
#7539=CARTESIAN_POINT('Ctrl Pts',(-37.3457382515077,-29.9241684761042,9.89414352051621));
#7540=CARTESIAN_POINT('Ctrl Pts',(-37.5424734719262,-29.0003511034471,9.9470717602581));
#7541=CARTESIAN_POINT('Ctrl Pts',(-38.0865340033349,-28.364012796625,10.));
#7542=CARTESIAN_POINT('',(-41.9171063737423,-28.3612428889485,9.99999999999999));
#7543=CARTESIAN_POINT('Origin',(-40.,-30.,10.));
#7544=CARTESIAN_POINT('Ctrl Pts',(-41.9171093217586,-28.3612406458477,9.99999999999999));
#7545=CARTESIAN_POINT('Ctrl Pts',(-41.3863011191192,-27.7421368159147,9.94821753066412));
#7546=CARTESIAN_POINT('Ctrl Pts',(-40.5267001215146,-27.402643603469,9.89643506132826));
#7547=CARTESIAN_POINT('Ctrl Pts',(-39.7163628817935,-27.4944831131097,9.84465259199239));
#7548=CARTESIAN_POINT('Ctrl Pts',(-38.8880956275312,-27.5883547195893,9.79172435225049));
#7549=CARTESIAN_POINT('Ctrl Pts',(-38.1112963297669,-28.1328580831711,9.73879611250859));
#7550=CARTESIAN_POINT('Ctrl Pts',(-37.741032373656,-28.8793789981345,9.6858678727667));
#7551=CARTESIAN_POINT('Ctrl Pts',(-37.3707684175451,-29.6258999130979,9.6329396330248));
#7552=CARTESIAN_POINT('Ctrl Pts',(-37.4070398030878,-30.574438379443,9.58001139328291));
#7553=CARTESIAN_POINT('Ctrl Pts',(-37.8334966681989,-31.2904958074349,9.52708315354102));
#7554=CARTESIAN_POINT('Ctrl Pts',(-38.2599535333099,-32.0065532354269,9.47415491379913));
#7555=CARTESIAN_POINT('Ctrl Pts',(-39.0765958779895,-32.4901296250657,9.42122667405723));
#7556=CARTESIAN_POINT('Ctrl Pts',(-39.9094857309799,-32.5200284649321,9.36829843431533));
#7557=CARTESIAN_POINT('Ctrl Pts',(-40.7423755839703,-32.5499273047984,9.31537019457344));
#7558=CARTESIAN_POINT('Ctrl Pts',(-41.5915129452714,-32.1261485948923,9.26244195483154));
#7559=CARTESIAN_POINT('Ctrl Pts',(-42.0682756289179,-31.4425951450394,9.20951371508965));
#7560=CARTESIAN_POINT('Ctrl Pts',(-42.3593162521113,-31.0253187329899,9.1772035775571));
#7561=CARTESIAN_POINT('Ctrl Pts',(-42.5115909448116,-30.5112369105017,9.14489344002454));
#7562=CARTESIAN_POINT('Ctrl Pts',(-42.5142225916618,-29.9985870806183,9.11258330249199));
#7563=CARTESIAN_POINT('Origin',(40.,-30.,5.));
#7564=CARTESIAN_POINT('',(37.4865493719845,-29.9993943699827,0.387416697508021));
#7565=CARTESIAN_POINT('',(37.4843806918116,-30.0035003569228,0.112583302491982));
#7566=CARTESIAN_POINT('',(37.4825,-30.,5.));
#7567=CARTESIAN_POINT('',(38.0865340033349,-28.364012796625,0.));
#7568=CARTESIAN_POINT('Ctrl Pts',(37.4843806918116,-30.0035003569228,0.112583302491982));
#7569=CARTESIAN_POINT('Ctrl Pts',(37.4896304006503,-29.4109018718323,0.0750555349946546));
#7570=CARTESIAN_POINT('Ctrl Pts',(37.700778171916,-28.8151964396956,0.0375277674973273));
#7571=CARTESIAN_POINT('Ctrl Pts',(38.0865340033349,-28.364012796625,-6.93889390390723E-17));
#7572=CARTESIAN_POINT('',(41.9171064557029,-28.361242966669,2.14205110652297E-15));
#7573=CARTESIAN_POINT('Origin',(40.,-30.,0.));
#7574=CARTESIAN_POINT('Ctrl Pts',(41.9171094063105,-28.36124072171,6.72491220257403E-16));
#7575=CARTESIAN_POINT('Ctrl Pts',(41.3863012299091,-27.7421370139191,0.0517824693358735));
#7576=CARTESIAN_POINT('Ctrl Pts',(40.526700166155,-27.4026434779206,0.103564938671746));
#7577=CARTESIAN_POINT('Ctrl Pts',(39.7163628779809,-27.4944829225585,0.155347408007619));
#7578=CARTESIAN_POINT('Ctrl Pts',(38.8880955741935,-27.5883544625971,0.208275647749513));
#7579=CARTESIAN_POINT('Ctrl Pts',(38.1112962453924,-28.132858029856,0.261203887491408));
#7580=CARTESIAN_POINT('Ctrl Pts',(37.7410322801268,-28.8793790122715,0.314132127233303));
#7581=CARTESIAN_POINT('Ctrl Pts',(37.5701428159829,-29.223923938661,0.338560317324876));
#7582=CARTESIAN_POINT('Ctrl Pts',(37.4858509825759,-29.6115013564135,0.362988507416448));
#7583=CARTESIAN_POINT('Ctrl Pts',(37.4865493719845,-29.9993943699827,0.387416697508021));
#7584=CARTESIAN_POINT('Origin',(40.,-30.,5.));
#7585=CARTESIAN_POINT('',(37.4826514345854,-30.0023034644279,1.38741669750802));
#7586=CARTESIAN_POINT('',(37.4783313032867,-29.9998786620396,1.11258330249198));
#7587=CARTESIAN_POINT('',(37.4825,-30.,5.));
#7588=CARTESIAN_POINT('Ctrl Pts',(37.4783313032867,-29.9998786620396,1.11258330249198));
#7589=CARTESIAN_POINT('Ctrl Pts',(37.4783277518435,-29.994156258084,1.11221987985458));
#7590=CARTESIAN_POINT('Ctrl Pts',(37.4783455394907,-29.9884338787842,1.11185645721719));
#7591=CARTESIAN_POINT('Ctrl Pts',(37.478384732659,-29.9827116481148,1.11149303457979));
#7592=CARTESIAN_POINT('Ctrl Pts',(37.4840927574081,-29.1493359429073,1.05856479483789));
#7593=CARTESIAN_POINT('Ctrl Pts',(37.9438226319757,-28.3191127610073,1.005636555096));
#7594=CARTESIAN_POINT('Ctrl Pts',(38.6471445572473,-27.8719690967068,0.952708315354104));
#7595=CARTESIAN_POINT('Ctrl Pts',(39.3504664825189,-27.4248254324063,0.89978007561221));
#7596=CARTESIAN_POINT('Ctrl Pts',(40.2973804584944,-27.3607612857053,0.846851835870315));
#7597=CARTESIAN_POINT('Ctrl Pts',(41.0544289594598,-27.7093027682094,0.793923596128421));
#7598=CARTESIAN_POINT('Ctrl Pts',(41.8114774604251,-28.0578442507135,0.740995356386527));
#7599=CARTESIAN_POINT('Ctrl Pts',(42.3786604863801,-28.8189913624227,0.688067116644633));
#7600=CARTESIAN_POINT('Ctrl Pts',(42.4963855115501,-29.6439332601599,0.635138876902738));
#7601=CARTESIAN_POINT('Ctrl Pts',(42.61411053672,-30.4688751578969,0.582210637160844));
#7602=CARTESIAN_POINT('Ctrl Pts',(42.2823775611047,-31.3576118416619,0.529282397418949));
#7603=CARTESIAN_POINT('Ctrl Pts',(41.6529740852769,-31.9041367057679,0.476354157677056));
#7604=CARTESIAN_POINT('Ctrl Pts',(41.023570609449,-32.4506615698739,0.42342591793516));
#7605=CARTESIAN_POINT('Ctrl Pts',(40.0964966334085,-32.6549746143208,0.370497678193266));
#7606=CARTESIAN_POINT('Ctrl Pts',(39.2962223204593,-32.4219134063263,0.317569438451371));
#7607=CARTESIAN_POINT('Ctrl Pts',(38.4959480075102,-32.1888521983318,0.264641198709478));
#7608=CARTESIAN_POINT('Ctrl Pts',(37.8224733576524,-31.5184167378959,0.211712958967584));
#7609=CARTESIAN_POINT('Ctrl Pts',(37.5841047237564,-30.7212914641747,0.158784719225691));
#7610=CARTESIAN_POINT('Ctrl Pts',(37.5147468620895,-30.4893527918657,0.143384246981121));
#7611=CARTESIAN_POINT('Ctrl Pts',(37.4822263404964,-30.2466881917031,0.127983774736552));
#7612=CARTESIAN_POINT('Ctrl Pts',(37.4843806918116,-30.0035003569228,0.112583302491982));
#7613=CARTESIAN_POINT('Ctrl Pts',(37.4865493719845,-29.9993943699827,0.387416697508021));
#7614=CARTESIAN_POINT('Ctrl Pts',(37.4873641737667,-30.4519440719579,0.415916747158343));
#7615=CARTESIAN_POINT('Ctrl Pts',(37.603864126948,-30.9049233498139,0.444416796808666));
#7616=CARTESIAN_POINT('Ctrl Pts',(37.8334965944027,-31.2904958242251,0.472916846458989));
#7617=CARTESIAN_POINT('Ctrl Pts',(38.2599534756744,-32.0065532561908,0.525845086200882));
#7618=CARTESIAN_POINT('Ctrl Pts',(39.0765958399479,-32.4901297225502,0.578773325942776));
#7619=CARTESIAN_POINT('Ctrl Pts',(39.9094857226646,-32.5200285765499,0.63170156568467));
#7620=CARTESIAN_POINT('Ctrl Pts',(40.7423756053813,-32.5499274305496,0.684629805426564));
#7621=CARTESIAN_POINT('Ctrl Pts',(41.5915130065413,-32.1261486721896,0.737558045168459));
#7622=CARTESIAN_POINT('Ctrl Pts',(42.0682757093793,-31.442595189452,0.790486284910354));
#7623=CARTESIAN_POINT('Ctrl Pts',(42.5450384122174,-30.7590417067144,0.843414524652249));
#7624=CARTESIAN_POINT('Ctrl Pts',(42.6494264167334,-29.8157134995992,0.896342764394142));
#7625=CARTESIAN_POINT('Ctrl Pts',(42.3336252269733,-29.0444504835271,0.949271004136037));
#7626=CARTESIAN_POINT('Ctrl Pts',(42.0178240372131,-28.273187467455,1.00219924387793));
#7627=CARTESIAN_POINT('Ctrl Pts',(41.2818336531767,-27.6739896424261,1.05512748361983));
#7628=CARTESIAN_POINT('Ctrl Pts',(40.462563489583,-27.5211152279163,1.10805572336172));
#7629=CARTESIAN_POINT('Ctrl Pts',(39.6432933259892,-27.3682408134066,1.16098396310362));
#7630=CARTESIAN_POINT('Ctrl Pts',(38.7407433828381,-27.6616898094161,1.21391220284551));
#7631=CARTESIAN_POINT('Ctrl Pts',(38.1680404837585,-28.2671481925974,1.26684044258741));
#7632=CARTESIAN_POINT('Ctrl Pts',(37.7331474342891,-28.7269147539535,1.30703252756094));
#7633=CARTESIAN_POINT('Ctrl Pts',(37.4884579998333,-29.3665989905621,1.34722461253448));
#7634=CARTESIAN_POINT('Ctrl Pts',(37.4826514345854,-30.0023034644279,1.38741669750802));
#7635=CARTESIAN_POINT('Origin',(40.,-30.,5.));
#7636=CARTESIAN_POINT('',(37.4786866123615,-29.9991346485264,2.38741669750802));
#7637=CARTESIAN_POINT('',(37.4841920048104,-29.9978709034909,2.11258330249198));
#7638=CARTESIAN_POINT('',(37.4825,-30.,5.));
#7639=CARTESIAN_POINT('Ctrl Pts',(37.4841920048104,-29.9978709034909,2.11258330249198));
#7640=CARTESIAN_POINT('Ctrl Pts',(37.4821417199046,-29.7423941828823,2.09645598497262));
#7641=CARTESIAN_POINT('Ctrl Pts',(37.5179332422556,-29.4874784679461,2.08032866745325));
#7642=CARTESIAN_POINT('Ctrl Pts',(37.5939460125011,-29.2451808863826,2.06420134993389));
#7643=CARTESIAN_POINT('Ctrl Pts',(37.8434123060845,-28.4499845079103,2.011273110192));
#7644=CARTESIAN_POINT('Ctrl Pts',(38.5260962765078,-27.7906963548654,1.9583448704501));
#7645=CARTESIAN_POINT('Ctrl Pts',(39.3295050974595,-27.5690985418568,1.90541663070821));
#7646=CARTESIAN_POINT('Ctrl Pts',(40.1329139184113,-27.3475007288482,1.85248839096631));
#7647=CARTESIAN_POINT('Ctrl Pts',(41.0570475898915,-27.563593255876,1.79956015122442));
#7648=CARTESIAN_POINT('Ctrl Pts',(41.6788913122662,-28.1184647318748,1.74663191148252));
#7649=CARTESIAN_POINT('Ctrl Pts',(42.300735034641,-28.6733362078736,1.69370367174063));
#7650=CARTESIAN_POINT('Ctrl Pts',(42.6202888079102,-29.5669866328433,1.64077543199873));
#7651=CARTESIAN_POINT('Ctrl Pts',(42.4912800198408,-30.3903485605237,1.58784719225684));
#7652=CARTESIAN_POINT('Ctrl Pts',(42.3622712317715,-31.2137104882041,1.53491895251494));
#7653=CARTESIAN_POINT('Ctrl Pts',(41.7846998823636,-31.9667839185952,1.48199071277305));
#7654=CARTESIAN_POINT('Ctrl Pts',(41.0229435118419,-32.3048683773518,1.42906247303116));
#7655=CARTESIAN_POINT('Ctrl Pts',(40.2611871413201,-32.6429528361084,1.37613423328926));
#7656=CARTESIAN_POINT('Ctrl Pts',(39.3152457496845,-32.5660483232304,1.32320599354737));
#7657=CARTESIAN_POINT('Ctrl Pts',(38.6181181413319,-32.1093319525339,1.27027775380547));
#7658=CARTESIAN_POINT('Ctrl Pts',(37.9257772395706,-31.6557515460937,1.21771293670098));
#7659=CARTESIAN_POINT('Ctrl Pts',(37.4788449778475,-30.8275572003943,1.16514811959648));
#7660=CARTESIAN_POINT('Ctrl Pts',(37.4783313032867,-29.9998786620396,1.11258330249198));
#7661=CARTESIAN_POINT('Ctrl Pts',(37.4826514345854,-30.0023034644279,1.38741669750802));
#7662=CARTESIAN_POINT('Ctrl Pts',(37.4808114376377,-30.2037468722884,1.40015285227638));
#7663=CARTESIAN_POINT('Ctrl Pts',(37.5029586978307,-30.4047906550415,1.41288900704473));
#7664=CARTESIAN_POINT('Ctrl Pts',(37.5506421647824,-30.5995832878214,1.42562516181309));
#7665=CARTESIAN_POINT('Ctrl Pts',(37.748802599894,-31.4090922295111,1.47855340155498));
#7666=CARTESIAN_POINT('Ctrl Pts',(38.3879793251253,-32.1106423425376,1.53148164129688));
#7667=CARTESIAN_POINT('Ctrl Pts',(39.1755924790674,-32.3831073213503,1.58440988103877));
#7668=CARTESIAN_POINT('Ctrl Pts',(39.9632056330096,-32.6555723001631,1.63733812078066));
#7669=CARTESIAN_POINT('Ctrl Pts',(40.8992552156624,-32.4989521447621,1.69026636052256));
#7670=CARTESIAN_POINT('Ctrl Pts',(41.5552732606538,-31.9849372039589,1.74319460026445));
#7671=CARTESIAN_POINT('Ctrl Pts',(42.2112913056452,-31.4709222631558,1.79612284000635));
#7672=CARTESIAN_POINT('Ctrl Pts',(42.587277812975,-30.5995125369504,1.84905107974824));
#7673=CARTESIAN_POINT('Ctrl Pts',(42.5111275644027,-29.7695892476869,1.90197931949014));
#7674=CARTESIAN_POINT('Ctrl Pts',(42.4349773158305,-28.9396659584235,1.95490755923203));
#7675=CARTESIAN_POINT('Ctrl Pts',(41.9066903113561,-28.151229106102,2.00783579897393));
#7676=CARTESIAN_POINT('Ctrl Pts',(41.1680858141738,-27.7651788384674,2.06076403871582));
#7677=CARTESIAN_POINT('Ctrl Pts',(40.4294813169916,-27.3791285708329,2.11369227845772));
#7678=CARTESIAN_POINT('Ctrl Pts',(39.4805593271014,-27.3954648878851,2.16662051819961));
#7679=CARTESIAN_POINT('Ctrl Pts',(38.7556809223357,-27.8067101302471,2.21954875794151));
#7680=CARTESIAN_POINT('Ctrl Pts',(38.0308025175699,-28.217955372609,2.2724769976834));
#7681=CARTESIAN_POINT('Ctrl Pts',(37.5299676979286,-29.0241095402806,2.3254052374253));
#7682=CARTESIAN_POINT('Ctrl Pts',(37.4824295281584,-29.8561621440027,2.37833347716719));
#7683=CARTESIAN_POINT('Ctrl Pts',(37.4797101249769,-29.9037594012931,2.3813612172808));
#7684=CARTESIAN_POINT('Ctrl Pts',(37.4784740757625,-29.9514414078264,2.38438895739441));
#7685=CARTESIAN_POINT('Ctrl Pts',(37.4786866123615,-29.9991346485264,2.38741669750802));
#7686=CARTESIAN_POINT('Origin',(40.,-30.,5.));
#7687=CARTESIAN_POINT('',(37.4852131002495,-29.9982362785157,3.38741669750802));
#7688=CARTESIAN_POINT('',(37.4858831881014,-30.0013301674969,3.11258330249199));
#7689=CARTESIAN_POINT('',(37.4825,-30.,5.));
#7690=CARTESIAN_POINT('Ctrl Pts',(37.4858831881014,-30.0013301674969,3.11258330249199));
#7691=CARTESIAN_POINT('Ctrl Pts',(37.4883078730657,-29.4952785276618,3.08069209009065));
#7692=CARTESIAN_POINT('Ctrl Pts',(37.636378023608,-28.987921426998,3.04880087768932));
#7693=CARTESIAN_POINT('Ctrl Pts',(37.9203890614956,-28.5737932182074,3.01690966528799));
#7694=CARTESIAN_POINT('Ctrl Pts',(38.3917478832765,-27.8864854782912,2.96398142554609));
#7695=CARTESIAN_POINT('Ctrl Pts',(39.2375473130611,-27.4559708463078,2.9110531858042));
#7696=CARTESIAN_POINT('Ctrl Pts',(40.0706296497584,-27.4793138140309,2.85812494606231));
#7697=CARTESIAN_POINT('Ctrl Pts',(40.9037119864556,-27.502656781754,2.80519670632041));
#7698=CARTESIAN_POINT('Ctrl Pts',(41.7240772300655,-27.9798573491834,2.75226846657852));
#7699=CARTESIAN_POINT('Ctrl Pts',(42.1562099623478,-28.6924809482542,2.69934022683662));
#7700=CARTESIAN_POINT('Ctrl Pts',(42.5883426946301,-29.4051045473249,2.64641198709473));
#7701=CARTESIAN_POINT('Ctrl Pts',(42.6322429155848,-30.353151178037,2.59348374735284));
#7702=CARTESIAN_POINT('Ctrl Pts',(42.2678156693759,-31.1026602254528,2.54055550761094));
#7703=CARTESIAN_POINT('Ctrl Pts',(41.903388423167,-31.8521692728685,2.48762726786905));
#7704=CARTESIAN_POINT('Ctrl Pts',(41.1306337097946,-32.4031407369879,2.43469902812715));
#7705=CARTESIAN_POINT('Ctrl Pts',(40.3032736012765,-32.503372180972,2.38177078838526));
#7706=CARTESIAN_POINT('Ctrl Pts',(39.4759134927584,-32.6036036249562,2.32884254864336));
#7707=CARTESIAN_POINT('Ctrl Pts',(38.5939479890946,-32.2530950488052,2.27591430890147));
#7708=CARTESIAN_POINT('Ctrl Pts',(38.0610895456344,-31.6122884587799,2.22298606915957));
#7709=CARTESIAN_POINT('Ctrl Pts',(37.6905939041957,-31.1667366400493,2.18618514693704));
#7710=CARTESIAN_POINT('Ctrl Pts',(37.4888705494763,-30.5808431748248,2.14938422471451));
#7711=CARTESIAN_POINT('Ctrl Pts',(37.4841920048104,-29.9978709034909,2.11258330249198));
#7712=CARTESIAN_POINT('Ctrl Pts',(37.4786866123615,-29.9991346485264,2.38741669750802));
#7713=CARTESIAN_POINT('Ctrl Pts',(37.4821894501486,-30.7851719075128,2.43731719713631));
#7714=CARTESIAN_POINT('Ctrl Pts',(37.8791670000235,-31.5742606671538,2.48721769676459));
#7715=CARTESIAN_POINT('Ctrl Pts',(38.5139723441797,-32.0372952999983,2.53711819639287));
#7716=CARTESIAN_POINT('Ctrl Pts',(39.1872948498703,-32.5284248124992,2.59004643613477));
#7717=CARTESIAN_POINT('Ctrl Pts',(40.1281813811507,-32.6527327977285,2.64297467587666));
#7718=CARTESIAN_POINT('Ctrl Pts',(40.9059489153952,-32.3533182827517,2.69590291561856));
#7719=CARTESIAN_POINT('Ctrl Pts',(41.6837164496398,-32.0539037677748,2.74883115536045));
#7720=CARTESIAN_POINT('Ctrl Pts',(42.2983649868485,-31.3307667525918,2.80175939510234));
#7721=CARTESIAN_POINT('Ctrl Pts',(42.4685442279864,-30.5149172428125,2.85468763484424));
#7722=CARTESIAN_POINT('Ctrl Pts',(42.6387234691244,-29.6990677330333,2.90761587458613));
#7723=CARTESIAN_POINT('Ctrl Pts',(42.3644334141915,-28.7905057286578,2.96054411432803));
#7724=CARTESIAN_POINT('Ctrl Pts',(41.7712280742516,-28.2051179779666,3.01347235406992));
#7725=CARTESIAN_POINT('Ctrl Pts',(41.1780227343116,-27.6197302272753,3.06640059381182));
#7726=CARTESIAN_POINT('Ctrl Pts',(40.2659021093645,-27.3575167302683,3.11932883355372));
#7727=CARTESIAN_POINT('Ctrl Pts',(39.4523818797609,-27.5385035518619,3.17225707329561));
#7728=CARTESIAN_POINT('Ctrl Pts',(38.6388616501573,-27.7194903734554,3.2251853130375));
#7729=CARTESIAN_POINT('Ctrl Pts',(37.9239418158972,-28.3436775136496,3.2781135527794));
#7730=CARTESIAN_POINT('Ctrl Pts',(37.6348710271545,-29.1253484633316,3.33104179252129));
#7731=CARTESIAN_POINT('Ctrl Pts',(37.532239373874,-29.4028728103475,3.34983342751687));
#7732=CARTESIAN_POINT('Ctrl Pts',(37.4832873999723,-29.7002485119447,3.36862506251244));
#7733=CARTESIAN_POINT('Ctrl Pts',(37.4852131002495,-29.9982362785157,3.38741669750802));
#7734=CARTESIAN_POINT('Origin',(40.,-30.,5.));
#7735=CARTESIAN_POINT('',(37.4850673154095,-30.0018328376965,4.38741669750802));
#7736=CARTESIAN_POINT('',(37.4793388029256,-30.0014234821656,4.11258330249199));
#7737=CARTESIAN_POINT('',(37.4825,-30.,5.));
#7738=CARTESIAN_POINT('Ctrl Pts',(37.4793388029256,-30.0014234821656,4.11258330249199));
#7739=CARTESIAN_POINT('Ctrl Pts',(37.4844209002651,-29.2502423854113,4.06492819520869));
#7740=CARTESIAN_POINT('Ctrl Pts',(37.8421140990601,-28.4948609126137,4.01727308792539));
#7741=CARTESIAN_POINT('Ctrl Pts',(38.4291014552389,-28.0274064804584,3.96961798064209));
#7742=CARTESIAN_POINT('Ctrl Pts',(39.0810401305334,-27.5082272851111,3.9166897409002));
#7743=CARTESIAN_POINT('Ctrl Pts',(40.0158241190993,-27.3442198697122,3.86376150115831));
#7744=CARTESIAN_POINT('Ctrl Pts',(40.8055637711363,-27.610457273629,3.81083326141641));
#7745=CARTESIAN_POINT('Ctrl Pts',(41.5953034231733,-27.8766946775457,3.75790502167452));
#7746=CARTESIAN_POINT('Ctrl Pts',(42.2399987386814,-28.5731769007781,3.70497678193262));
#7747=CARTESIAN_POINT('Ctrl Pts',(42.4445457618467,-29.3810949590939,3.65204854219072));
#7748=CARTESIAN_POINT('Ctrl Pts',(42.6490927850121,-30.1890130174097,3.59912030244883));
#7749=CARTESIAN_POINT('Ctrl Pts',(42.4134915158347,-31.1083669108089,3.54619206270694));
#7750=CARTESIAN_POINT('Ctrl Pts',(41.8455864894317,-31.7183299864945,3.49326382296504));
#7751=CARTESIAN_POINT('Ctrl Pts',(41.2776814630286,-32.3282930621801,3.44033558322315));
#7752=CARTESIAN_POINT('Ctrl Pts',(40.3774726793999,-32.628865320152,3.38740734348125));
#7753=CARTESIAN_POINT('Ctrl Pts',(39.5570232736503,-32.4824622950877,3.33447910373936));
#7754=CARTESIAN_POINT('Ctrl Pts',(38.7365738679008,-32.3360592700233,3.28155086399746));
#7755=CARTESIAN_POINT('Ctrl Pts',(37.9958838400304,-31.7426809619227,3.22862262425557));
#7756=CARTESIAN_POINT('Ctrl Pts',(37.6739979329839,-30.9739413839478,3.17569438451368));
#7757=CARTESIAN_POINT('Ctrl Pts',(37.5460601315361,-30.6683956941894,3.15465735717311));
#7758=CARTESIAN_POINT('Ctrl Pts',(37.484283745495,-30.3351469584353,3.13362032983255));
#7759=CARTESIAN_POINT('Ctrl Pts',(37.4858831881014,-30.0013301674969,3.11258330249199));
#7760=CARTESIAN_POINT('Ctrl Pts',(37.4852131002495,-29.9982362785157,3.38741669750802));
#7761=CARTESIAN_POINT('Ctrl Pts',(37.4887112987426,-30.5395564249036,3.42155330225434));
#7762=CARTESIAN_POINT('Ctrl Pts',(37.6601048829887,-31.0828963744086,3.45568990700066));
#7763=CARTESIAN_POINT('Ctrl Pts',(37.9825966796778,-31.5129224074782,3.48982651174697));
#7764=CARTESIAN_POINT('Ctrl Pts',(38.4826148641692,-32.179670642773,3.54275475148887));
#7765=CARTESIAN_POINT('Ctrl Pts',(39.3458729763774,-32.5740123541928,3.59568299123076));
#7766=CARTESIAN_POINT('Ctrl Pts',(40.1772217458474,-32.5154408801314,3.64861123097266));
#7767=CARTESIAN_POINT('Ctrl Pts',(41.0085705153174,-32.4568694060699,3.70153947071455));
#7768=CARTESIAN_POINT('Ctrl Pts',(41.8080099420493,-31.9453847465272,3.75446771045645));
#7769=CARTESIAN_POINT('Ctrl Pts',(42.2096032313768,-31.2151147799068,3.80739595019834));
#7770=CARTESIAN_POINT('Ctrl Pts',(42.6111965207043,-30.4848448132865,3.86032418994024));
#7771=CARTESIAN_POINT('Ctrl Pts',(42.6149436726274,-29.5357895395886,3.91325242968213));
#7772=CARTESIAN_POINT('Ctrl Pts',(42.2191294593654,-28.8023711714614,3.96618066942403));
#7773=CARTESIAN_POINT('Ctrl Pts',(41.8233152461034,-28.0689528033342,4.01910890916592));
#7774=CARTESIAN_POINT('Ctrl Pts',(41.0279396676562,-27.5511713407776,4.07203714890781));
#7775=CARTESIAN_POINT('Ctrl Pts',(40.1970793255485,-27.4860369716512,4.12496538864971));
#7776=CARTESIAN_POINT('Ctrl Pts',(39.3662189834407,-27.4209026025248,4.1778936283916));
#7777=CARTESIAN_POINT('Ctrl Pts',(38.4998738776723,-27.8084153268287,4.2308218681335));
#7778=CARTESIAN_POINT('Ctrl Pts',(37.9946063247663,-28.4711943956907,4.2837501078754));
#7779=CARTESIAN_POINT('Ctrl Pts',(37.6647297200325,-28.9039063473437,4.31830563775294));
#7780=CARTESIAN_POINT('Ctrl Pts',(37.4887609409795,-29.4539494491559,4.35286116763048));
#7781=CARTESIAN_POINT('Ctrl Pts',(37.4850673154095,-30.0018328376965,4.38741669750802));
#7782=CARTESIAN_POINT('Origin',(40.,-30.,5.));
#7783=CARTESIAN_POINT('',(37.4785971457328,-30.0007512051729,5.38741669750803));
#7784=CARTESIAN_POINT('',(37.4815747780937,-29.9977798171256,5.11258330249199));
#7785=CARTESIAN_POINT('',(37.4825,-30.,5.));
#7786=CARTESIAN_POINT('Ctrl Pts',(37.4815747780937,-29.9977798171256,5.11258330249199));
#7787=CARTESIAN_POINT('Ctrl Pts',(37.4800513919894,-29.8320332010168,5.10209254006862));
#7788=CARTESIAN_POINT('Ctrl Pts',(37.4950144905386,-29.6665602978234,5.09160177764525));
#7789=CARTESIAN_POINT('Ctrl Pts',(37.5274672786068,-29.5045917111079,5.08111101522188));
#7790=CARTESIAN_POINT('Ctrl Pts',(37.691198843373,-28.6874240122915,5.02818277547998));
#7791=CARTESIAN_POINT('Ctrl Pts',(38.3001178421193,-27.9594561622746,4.97525453573809));
#7792=CARTESIAN_POINT('Ctrl Pts',(39.075496632593,-27.6539094316881,4.92232629599619));
#7793=CARTESIAN_POINT('Ctrl Pts',(39.8508754230667,-27.3483627011017,4.8693980562543));
#7794=CARTESIAN_POINT('Ctrl Pts',(40.7927140052677,-27.4652370899456,4.81646981651241));
#7795=CARTESIAN_POINT('Ctrl Pts',(41.4698935473972,-27.9510343120548,4.76354157677051));
#7796=CARTESIAN_POINT('Ctrl Pts',(42.1470730895267,-28.4368315341641,4.71061333702862));
#7797=CARTESIAN_POINT('Ctrl Pts',(42.5595935915846,-29.2915515895388,4.65768509728672));
#7798=CARTESIAN_POINT('Ctrl Pts',(42.5186272010046,-30.1239534324835,4.60475685754483));
#7799=CARTESIAN_POINT('Ctrl Pts',(42.4776608104246,-30.9563552754283,4.55182861780293));
#7800=CARTESIAN_POINT('Ctrl Pts',(41.9832075272066,-31.7664389059432,4.49890037806104));
#7801=CARTESIAN_POINT('Ctrl Pts',(41.2615992577626,-32.183395233096,4.44597213831914));
#7802=CARTESIAN_POINT('Ctrl Pts',(40.5399909883187,-32.6003515602488,4.39304389857725));
#7803=CARTESIAN_POINT('Ctrl Pts',(39.5912277326488,-32.6241805840396,4.34011565883535));
#7804=CARTESIAN_POINT('Ctrl Pts',(38.8495980346337,-32.243974765696,4.28718741909346));
#7805=CARTESIAN_POINT('Ctrl Pts',(38.1079683366186,-31.8637689473525,4.23425917935157));
#7806=CARTESIAN_POINT('Ctrl Pts',(37.5734721962583,-31.0795282868747,4.18133093960967));
#7807=CARTESIAN_POINT('Ctrl Pts',(37.4907708070897,-30.250232468988,4.12840269986778));
#7808=CARTESIAN_POINT('Ctrl Pts',(37.4825314365435,-30.1676114198769,4.12312956740918));
#7809=CARTESIAN_POINT('Ctrl Pts',(37.4787764587412,-30.0845431654355,4.11785643495059));
#7810=CARTESIAN_POINT('Ctrl Pts',(37.4793388029256,-30.0014234821656,4.11258330249199));
#7811=CARTESIAN_POINT('Ctrl Pts',(37.4850673154095,-30.0018328376965,4.38741669750802));
#7812=CARTESIAN_POINT('Ctrl Pts',(37.4831034644373,-30.2931350568442,4.40578940737237));
#7813=CARTESIAN_POINT('Ctrl Pts',(37.5298401746273,-30.5838267454182,4.42416211723672));
#7814=CARTESIAN_POINT('Ctrl Pts',(37.6280381061972,-30.8559480958414,4.44253482710107));
#7815=CARTESIAN_POINT('Ctrl Pts',(37.9109274405776,-31.6398773137099,4.49546306684297));
#7816=CARTESIAN_POINT('Ctrl Pts',(38.6208961093818,-32.2696903360266,4.54839130658486));
#7817=CARTESIAN_POINT('Ctrl Pts',(39.4329618185209,-32.4570954538202,4.60131954632676));
#7818=CARTESIAN_POINT('Ctrl Pts',(40.24502752766,-32.6445005716137,4.65424778606865));
#7819=CARTESIAN_POINT('Ctrl Pts',(41.1591902771339,-32.389497784884,4.70717602581055));
#7820=CARTESIAN_POINT('Ctrl Pts',(41.7569996189814,-31.8088125130406,4.76010426555244));
#7821=CARTESIAN_POINT('Ctrl Pts',(42.3548089608288,-31.2281272411973,4.81303250529434));
#7822=CARTESIAN_POINT('Ctrl Pts',(42.6362648950499,-30.3217594842401,4.86596074503623));
#7823=CARTESIAN_POINT('Ctrl Pts',(42.4725332924671,-29.5045915966848,4.91888898477813));
#7824=CARTESIAN_POINT('Ctrl Pts',(42.3088016898843,-28.6874237091295,4.97181722452002));
#7825=CARTESIAN_POINT('Ctrl Pts',(41.6998825504976,-27.959455690976,5.02474546426192));
#7826=CARTESIAN_POINT('Ctrl Pts',(40.9245035809369,-27.6539088898183,5.07767370400381));
#7827=CARTESIAN_POINT('Ctrl Pts',(40.1491246113762,-27.3483620886605,5.1306019437457));
#7828=CARTESIAN_POINT('Ctrl Pts',(39.2072858116414,-27.4652365044985,5.1835301834876));
#7829=CARTESIAN_POINT('Ctrl Pts',(38.5301061131057,-27.951033838811,5.23645842322949));
#7830=CARTESIAN_POINT('Ctrl Pts',(37.8863043721956,-28.4128863873091,5.286777847989));
#7831=CARTESIAN_POINT('Ctrl Pts',(37.4817147993667,-29.208189970679,5.33709727274851));
#7832=CARTESIAN_POINT('Ctrl Pts',(37.4785971457328,-30.0007512051729,5.38741669750803));
#7833=CARTESIAN_POINT('Origin',(40.,-30.,5.));
#7834=CARTESIAN_POINT('',(37.4828504064482,-29.9976988315479,6.38741669750802));
#7835=CARTESIAN_POINT('',(37.4865857580008,-29.9999453848463,6.11258330249199));
#7836=CARTESIAN_POINT('',(37.4825,-30.,5.));
#7837=CARTESIAN_POINT('Ctrl Pts',(37.4865857580008,-29.9999453848463,6.11258330249199));
#7838=CARTESIAN_POINT('Ctrl Pts',(37.4865051054086,-29.5830438800611,6.08632864518665));
#7839=CARTESIAN_POINT('Ctrl Pts',(37.5845304195934,-29.1661780579881,6.06007398788132));
#7840=CARTESIAN_POINT('Ctrl Pts',(37.7808710531806,-28.8023714480745,6.03381933057598));
#7841=CARTESIAN_POINT('Ctrl Pts',(38.1766851750226,-28.0689532493429,5.98089109083409));
#7842=CARTESIAN_POINT('Ctrl Pts',(38.972060569764,-27.5511719063765,5.92796285109219));
#7843=CARTESIAN_POINT('Ctrl Pts',(39.8029207199703,-27.4860375522939,5.8750346113503));
#7844=CARTESIAN_POINT('Ctrl Pts',(40.6337808701766,-27.4209031982113,5.8221063716084));
#7845=CARTESIAN_POINT('Ctrl Pts',(41.5001257758479,-27.8084158330126,5.76917813186651));
#7846=CARTESIAN_POINT('Ctrl Pts',(42.0053932120537,-28.4711947487945,5.71624989212461));
#7847=CARTESIAN_POINT('Ctrl Pts',(42.5106606482595,-29.1339736645764,5.66332165238272));
#7848=CARTESIAN_POINT('Ctrl Pts',(42.6548506149998,-30.0720188613389,5.61039341264082));
#7849=CARTESIAN_POINT('Ctrl Pts',(42.3719613459576,-30.8559478981455,5.55746517289893));
#7850=CARTESIAN_POINT('Ctrl Pts',(42.0890720769154,-31.6398769349521,5.50453693315703));
#7851=CARTESIAN_POINT('Ctrl Pts',(41.3791035720906,-32.2696898118028,5.45160869341514));
#7852=CARTESIAN_POINT('Ctrl Pts',(40.5670380505119,-32.4570948863119,5.39868045367324));
#7853=CARTESIAN_POINT('Ctrl Pts',(39.7549725289333,-32.6444999608211,5.34575221393135));
#7854=CARTESIAN_POINT('Ctrl Pts',(38.8408099906009,-32.3894972329887,5.29282397418945));
#7855=CARTESIAN_POINT('Ctrl Pts',(38.2430007868277,-31.8088120952645,5.23989573444756));
#7856=CARTESIAN_POINT('Ctrl Pts',(37.7636817191685,-31.3432229791037,5.19745825712904));
#7857=CARTESIAN_POINT('Ctrl Pts',(37.4877372151636,-30.6682619020185,5.15502077981051));
#7858=CARTESIAN_POINT('Ctrl Pts',(37.4815747780937,-29.9977798171256,5.11258330249199));
#7859=CARTESIAN_POINT('Ctrl Pts',(37.4785971457328,-30.0007512051729,5.38741669750803));
#7860=CARTESIAN_POINT('Ctrl Pts',(37.4784355107072,-30.0418416117681,5.39002551249041));
#7861=CARTESIAN_POINT('Ctrl Pts',(37.4793529973139,-30.0829246471678,5.39263432747279));
#7862=CARTESIAN_POINT('Ctrl Pts',(37.4813722172753,-30.1239534611127,5.39524314245518));
#7863=CARTESIAN_POINT('Ctrl Pts',(37.5223386173172,-30.956355496315,5.44817138219707));
#7864=CARTESIAN_POINT('Ctrl Pts',(38.0167920147376,-31.7664393139323,5.50109962193897));
#7865=CARTESIAN_POINT('Ctrl Pts',(38.7384004508494,-32.1833957373885,5.55402786168086));
#7866=CARTESIAN_POINT('Ctrl Pts',(39.4600088869611,-32.6003521608446,5.60695610142275));
#7867=CARTESIAN_POINT('Ctrl Pts',(40.4087723617641,-32.6241811901395,5.65988434116465));
#7868=CARTESIAN_POINT('Ctrl Pts',(41.1504022310713,-32.2439752839807,5.71281258090654));
#7869=CARTESIAN_POINT('Ctrl Pts',(41.8920321003785,-31.8637693778219,5.76574082064844));
#7870=CARTESIAN_POINT('Ctrl Pts',(42.42652836419,-31.0795285362096,5.81866906039033));
#7871=CARTESIAN_POINT('Ctrl Pts',(42.5092297724598,-30.2502325267831,5.87159730013223));
#7872=CARTESIAN_POINT('Ctrl Pts',(42.5919311807296,-29.4209365173566,5.92452553987412));
#7873=CARTESIAN_POINT('Ctrl Pts',(42.2228377334579,-28.5465853401159,5.97745377961602));
#7874=CARTESIAN_POINT('Ctrl Pts',(41.570898907587,-28.0274060248547,6.03038201935791));
#7875=CARTESIAN_POINT('Ctrl Pts',(40.9189600817161,-27.5082267095935,6.08331025909981));
#7876=CARTESIAN_POINT('Ctrl Pts',(39.984175877246,-27.3442192563117,6.1362384988417));
#7877=CARTESIAN_POINT('Ctrl Pts',(39.194436042805,-27.6104567217217,6.18916673858359));
#7878=CARTESIAN_POINT('Ctrl Pts',(38.404696208364,-27.8766941871318,6.24209497832549));
#7879=CARTESIAN_POINT('Ctrl Pts',(37.7600007439522,-28.5731765712337,6.29502321806739));
#7880=CARTESIAN_POINT('Ctrl Pts',(37.5554536735433,-29.3810948161497,6.34795145780928));
#7881=CARTESIAN_POINT('Ctrl Pts',(37.5046144038534,-29.5818993227048,6.36110653770886));
#7882=CARTESIAN_POINT('Ctrl Pts',(37.4809652589362,-29.7895877688607,6.37426161760844));
#7883=CARTESIAN_POINT('Ctrl Pts',(37.4828504064482,-29.9976988315479,6.38741669750802));
#7884=CARTESIAN_POINT('Origin',(40.,-30.,5.));
#7885=CARTESIAN_POINT('',(37.4864395637057,-30.0006322084003,7.38741669750802));
#7886=CARTESIAN_POINT('',(37.4817753207913,-30.0022480736136,7.11258330249199));
#7887=CARTESIAN_POINT('',(37.4825,-30.,5.));
#7888=CARTESIAN_POINT('Ctrl Pts',(37.4817753207913,-30.0022480736136,7.11258330249199));
#7889=CARTESIAN_POINT('Ctrl Pts',(37.4879012302583,-29.3382487112704,7.07056475030469));
#7890=CARTESIAN_POINT('Ctrl Pts',(37.7578399195865,-28.6698445990111,7.02854619811738));
#7891=CARTESIAN_POINT('Ctrl Pts',(38.2287723348486,-28.2051183925334,6.98652764593008));
#7892=CARTESIAN_POINT('Ctrl Pts',(38.8219775377818,-27.6197307770547,6.93359940618819));
#7893=CARTESIAN_POINT('Ctrl Pts',(39.7340979520498,-27.3575173405945,6.88067116644629));
#7894=CARTESIAN_POINT('Ctrl Pts',(40.5476179937548,-27.5385041203823,6.82774292670439));
#7895=CARTESIAN_POINT('Ctrl Pts',(41.3611380354598,-27.7194909001701,6.7748146869625));
#7896=CARTESIAN_POINT('Ctrl Pts',(42.0760577046018,-28.3436778962059,6.72188644722061));
#7897=CARTESIAN_POINT('Ctrl Pts',(42.3651284265798,-29.1253486653496,6.66895820747872));
#7898=CARTESIAN_POINT('Ctrl Pts',(42.6541991485579,-29.9070194344933,6.61602996773682));
#7899=CARTESIAN_POINT('Ctrl Pts',(42.517420923372,-30.8461739767449,6.56310172799492));
#7900=CARTESIAN_POINT('Ctrl Pts',(42.0174028543677,-31.5129220580417,6.51017348825303));
#7901=CARTESIAN_POINT('Ctrl Pts',(41.5173847853634,-32.1796701393386,6.45724524851113));
#7902=CARTESIAN_POINT('Ctrl Pts',(40.6541268725408,-32.5740117596807,6.40431700876924));
#7903=CARTESIAN_POINT('Ctrl Pts',(39.8227782950853,-32.5154402991479,6.35138876902734));
#7904=CARTESIAN_POINT('Ctrl Pts',(38.9914297176298,-32.4568688386151,6.29846052928545));
#7905=CARTESIAN_POINT('Ctrl Pts',(38.1919904755415,-31.9453842972072,6.24553228954355));
#7906=CARTESIAN_POINT('Ctrl Pts',(37.7903972789686,-31.215114499255,6.19260404980166));
#7907=CARTESIAN_POINT('Ctrl Pts',(37.5880113827631,-30.8470895705667,6.1659304673651));
#7908=CARTESIAN_POINT('Ctrl Pts',(37.4866676975036,-30.4234990624467,6.13925688492854));
#7909=CARTESIAN_POINT('Ctrl Pts',(37.4865857580008,-29.9999453848463,6.11258330249199));
#7910=CARTESIAN_POINT('Ctrl Pts',(37.4828504064482,-29.9976988315479,6.38741669750802));
#7911=CARTESIAN_POINT('Ctrl Pts',(37.4885499745158,-30.6269032624138,6.42718985735033));
#7912=CARTESIAN_POINT('Ctrl Pts',(37.7276582419413,-31.2599708265612,6.46696301719264));
#7913=CARTESIAN_POINT('Ctrl Pts',(38.1544130842988,-31.7183303833674,6.50673617703496));
#7914=CARTESIAN_POINT('Ctrl Pts',(38.7223182418689,-32.3282935999387,6.55966441677685));
#7915=CARTESIAN_POINT('Ctrl Pts',(39.6225272334149,-32.6288659273512,6.61259265651875));
#7916=CARTESIAN_POINT('Ctrl Pts',(40.4429768286621,-32.4824628684643,6.66552089626065));
#7917=CARTESIAN_POINT('Ctrl Pts',(41.2634264239092,-32.3360598095774,6.71844913600254));
#7918=CARTESIAN_POINT('Ctrl Pts',(42.0041166228575,-31.742681364391,6.77137737574443));
#7919=CARTESIAN_POINT('Ctrl Pts',(42.3260026042476,-30.9739416088782,6.82430561548633));
#7920=CARTESIAN_POINT('Ctrl Pts',(42.6478885856377,-30.2052018533655,6.87723385522822));
#7921=CARTESIAN_POINT('Ctrl Pts',(42.5509703494696,-29.2611007875262,6.93016209497012));
#7922=CARTESIAN_POINT('Ctrl Pts',(42.0796114188234,-28.5737928888347,6.98309033471202));
#7923=CARTESIAN_POINT('Ctrl Pts',(41.6082524881772,-27.8864849901432,7.03601857445391));
#7924=CARTESIAN_POINT('Ctrl Pts',(40.762452863053,-27.4559702585993,7.0889468141958));
#7925=CARTESIAN_POINT('Ctrl Pts',(39.9293703339345,-27.4793132317701,7.1418750539377));
#7926=CARTESIAN_POINT('Ctrl Pts',(39.096287804816,-27.5026562049409,7.19480329367959));
#7927=CARTESIAN_POINT('Ctrl Pts',(38.2759223717032,-27.9798568828263,7.24773153342148));
#7928=CARTESIAN_POINT('Ctrl Pts',(37.8437895396261,-28.6924806463837,7.30065977316338));
#7929=CARTESIAN_POINT('Ctrl Pts',(37.6076804505263,-29.0818445993046,7.32957874794493));
#7930=CARTESIAN_POINT('Ctrl Pts',(37.4874712144567,-29.5414898757325,7.35849772272648));
#7931=CARTESIAN_POINT('Ctrl Pts',(37.4864395637057,-30.0006322084003,7.38741669750802));
#7932=CARTESIAN_POINT('Origin',(40.,-30.,5.));
#7933=CARTESIAN_POINT('',(37.4805319060517,-30.0019779656107,8.38741669750802));
#7934=CARTESIAN_POINT('',(37.4791974871636,-29.9986726512116,8.11258330249198));
#7935=CARTESIAN_POINT('',(37.4825,-30.,5.));
#7936=CARTESIAN_POINT('Ctrl Pts',(37.4791974871636,-29.9986726512116,8.11258330249198));
#7937=CARTESIAN_POINT('Ctrl Pts',(37.478708128852,-29.9221677179019,8.10772909516461));
#7938=CARTESIAN_POINT('Ctrl Pts',(37.4818890495647,-29.8457040321827,8.10287488783723));
#7939=CARTESIAN_POINT('Ctrl Pts',(37.4888730152059,-29.7695893001576,8.09802068050986));
#7940=CARTESIAN_POINT('Ctrl Pts',(37.565023245898,-28.9396662019417,8.04509244076796));
#7941=CARTESIAN_POINT('Ctrl Pts',(38.0933101290704,-28.1512295331621,7.99216420102607));
#7942=CARTESIAN_POINT('Ctrl Pts',(38.8319144558216,-27.7651793550315,7.93923596128418));
#7943=CARTESIAN_POINT('Ctrl Pts',(39.5705187825728,-27.379129176901,7.88630772154229));
#7944=CARTESIAN_POINT('Ctrl Pts',(40.5194405529029,-27.3954654894196,7.83337948180039));
#7945=CARTESIAN_POINT('Ctrl Pts',(41.2443187901563,-27.8067106366176,7.7804512420585));
#7946=CARTESIAN_POINT('Ctrl Pts',(41.9691970274096,-28.2179557838156,7.72752300231661));
#7947=CARTESIAN_POINT('Ctrl Pts',(42.4700317315862,-29.024109765693,7.67459476257471));
#7948=CARTESIAN_POINT('Ctrl Pts',(42.5175698904255,-29.8561621773333,7.62166652283281));
#7949=CARTESIAN_POINT('Ctrl Pts',(42.5651080492647,-30.6882145889737,7.56873828309092));
#7950=CARTESIAN_POINT('Ctrl Pts',(42.1593496627666,-31.546165430377,7.51581004334902));
#7951=CARTESIAN_POINT('Ctrl Pts',(41.4860273125649,-32.0372948293931,7.46288180360713));
#7952=CARTESIAN_POINT('Ctrl Pts',(40.8127049623631,-32.5284242284091,7.40995356386524));
#7953=CARTESIAN_POINT('Ctrl Pts',(39.8718186484578,-32.652732185038,7.35702532412334));
#7954=CARTESIAN_POINT('Ctrl Pts',(39.0940512938662,-32.3533177392424,7.30409708438145));
#7955=CARTESIAN_POINT('Ctrl Pts',(38.3162839392746,-32.0539032934467,7.25116884463955));
#7956=CARTESIAN_POINT('Ctrl Pts',(37.7016355439968,-31.3307664452267,7.19824060489766));
#7957=CARTESIAN_POINT('Ctrl Pts',(37.531456342157,-30.514917123868,7.14531236515576));
#7958=CARTESIAN_POINT('Ctrl Pts',(37.4963786231659,-30.34675243086,7.13440267760117));
#7959=CARTESIAN_POINT('Ctrl Pts',(37.4801847910183,-30.1746487205307,7.12349299004658));
#7960=CARTESIAN_POINT('Ctrl Pts',(37.4817753207913,-30.0022480736136,7.11258330249199));
#7961=CARTESIAN_POINT('Ctrl Pts',(37.4864395637057,-30.0006322084003,7.38741669750802));
#7962=CARTESIAN_POINT('Ctrl Pts',(37.4855830611354,-30.3818237963733,7.41142596246837));
#7963=CARTESIAN_POINT('Ctrl Pts',(37.5668725783754,-30.7626687182516,7.43543522742872));
#7964=CARTESIAN_POINT('Ctrl Pts',(37.7321838068588,-31.1026604798972,7.45944449238906));
#7965=CARTESIAN_POINT('Ctrl Pts',(38.0966111372102,-31.8521697006237,7.51237273213096));
#7966=CARTESIAN_POINT('Ctrl Pts',(38.8693660289545,-32.4031412928472,7.56530097187285));
#7967=CARTESIAN_POINT('Ctrl Pts',(39.696726328624,-32.5033727596101,7.61822921161475));
#7968=CARTESIAN_POINT('Ctrl Pts',(40.5240866282935,-32.603604226373,7.67115745135664));
#7969=CARTESIAN_POINT('Ctrl Pts',(41.4060523358881,-32.2530955676754,7.72408569109853));
#7970=CARTESIAN_POINT('Ctrl Pts',(41.9389109023006,-31.6122888303354,7.77701393084043));
#7971=CARTESIAN_POINT('Ctrl Pts',(42.4717694687131,-30.9714820929955,7.82994217058232));
#7972=CARTESIAN_POINT('Ctrl Pts',(42.6555208939435,-30.0403772770133,7.88287041032422));
#7973=CARTESIAN_POINT('Ctrl Pts',(42.40605454299,-29.2451807135995,7.93579865006611));
#7974=CARTESIAN_POINT('Ctrl Pts',(42.1565881920366,-28.4499841501856,7.98872688980801));
#7975=CARTESIAN_POINT('Ctrl Pts',(41.4739040648993,-27.7906958393402,8.0416551295499));
#7976=CARTESIAN_POINT('Ctrl Pts',(40.6704950578746,-27.569097977497,8.09458336929179));
#7977=CARTESIAN_POINT('Ctrl Pts',(39.8670860508498,-27.3475001156537,8.14751160903369));
#7978=CARTESIAN_POINT('Ctrl Pts',(38.9429521639374,-27.5635927028126,8.20043984877559));
#7979=CARTESIAN_POINT('Ctrl Pts',(38.3211082989912,-28.1184643026878,8.25336808851748));
#7980=CARTESIAN_POINT('Ctrl Pts',(37.7961377255517,-28.5868958148278,8.298050958181));
#7981=CARTESIAN_POINT('Ctrl Pts',(37.4866094758723,-29.2967753816077,8.34273382784451));
#7982=CARTESIAN_POINT('Ctrl Pts',(37.4805319060517,-30.0019779656107,8.38741669750802));
#7983=CARTESIAN_POINT('Origin',(40.,-30.,5.));
#7984=CARTESIAN_POINT('',(37.4802181636634,-29.9981833349058,9.38741669750803));
#7985=CARTESIAN_POINT('',(37.4857778982365,-29.998587099551,9.11258330249199));
#7986=CARTESIAN_POINT('',(37.4825,-30.,5.));
#7987=CARTESIAN_POINT('',(41.9134659966651,-28.3640127966251,10.));
#7988=CARTESIAN_POINT('Ctrl Pts',(37.4802181636634,-29.9981833349058,9.38741669750803));
#7989=CARTESIAN_POINT('Ctrl Pts',(37.4861414700995,-30.7144624754953,9.43282641244634));
#7990=CARTESIAN_POINT('Ctrl Pts',(37.8070289114727,-31.4352475048581,9.47823612738464));
#7991=CARTESIAN_POINT('Ctrl Pts',(38.3470252274242,-31.904137664027,9.52364584232294));
#7992=CARTESIAN_POINT('Ctrl Pts',(38.9764291888727,-32.4506623623392,9.57657408206484));
#7993=CARTESIAN_POINT('Ctrl Pts',(39.9035046931223,-32.6549739267535,9.62950232180674));
#7994=CARTESIAN_POINT('Ctrl Pts',(40.7037783386841,-32.421913350571,9.68243056154863));
#7995=CARTESIAN_POINT('Ctrl Pts',(41.5040519842458,-32.1888527743885,9.73535880129053));
#7996=CARTESIAN_POINT('Ctrl Pts',(42.1775237711198,-31.5184200576092,9.78828704103242));
#7997=CARTESIAN_POINT('Ctrl Pts',(42.4158924070768,-30.7212946398739,9.84121528077432));
#7998=CARTESIAN_POINT('Ctrl Pts',(42.6542610430338,-29.9241692221385,9.89414352051621));
#7999=CARTESIAN_POINT('Ctrl Pts',(42.4575265280738,-29.0003511034471,9.94707176025811));
#8000=CARTESIAN_POINT('Ctrl Pts',(41.9134659966651,-28.364012796625,10.));
#8001=CARTESIAN_POINT('',(38.0828940514472,-28.3612424815972,10.));
#8002=CARTESIAN_POINT('Origin',(40.,-30.,10.));
#8003=CARTESIAN_POINT('Ctrl Pts',(38.0828911169303,-28.3612402481786,10.));
#8004=CARTESIAN_POINT('Ctrl Pts',(38.6136994556452,-27.7421357853924,9.94821753066413));
#8005=CARTESIAN_POINT('Ctrl Pts',(39.4733001098964,-27.4026442541442,9.89643506132826));
#8006=CARTESIAN_POINT('Ctrl Pts',(40.2836370984124,-27.4944841015763,9.84465259199238));
#8007=CARTESIAN_POINT('Ctrl Pts',(41.1119040959113,-27.5883560533215,9.79172435225049));
#8008=CARTESIAN_POINT('Ctrl Pts',(41.8887032331835,-28.1328583586548,9.7387961125086));
#8009=CARTESIAN_POINT('Ctrl Pts',(42.2589671420342,-28.8793789236736,9.6858678727667));
#8010=CARTESIAN_POINT('Ctrl Pts',(42.629231050885,-29.6258994886923,9.6329396330248));
#8011=CARTESIAN_POINT('Ctrl Pts',(42.5929597313141,-30.5744383133966,9.58001139328291));
#8012=CARTESIAN_POINT('Ctrl Pts',(42.1665029498384,-31.2904957212721,9.52708315354101));
#8013=CARTESIAN_POINT('Ctrl Pts',(41.7400461683628,-32.0065531291476,9.47415491379912));
#8014=CARTESIAN_POINT('Ctrl Pts',(40.9234039249823,-32.4901291201944,9.42122667405723));
#8015=CARTESIAN_POINT('Ctrl Pts',(40.0905142258871,-32.5200278866053,9.36829843431534));
#8016=CARTESIAN_POINT('Ctrl Pts',(39.2576245267919,-32.5499266530163,9.31537019457344));
#8017=CARTESIAN_POINT('Ctrl Pts',(38.408487371982,-32.1261481947915,9.26244195483155));
#8018=CARTESIAN_POINT('Ctrl Pts',(37.9317247877119,-31.4425949153635,9.20951371508965));
#8019=CARTESIAN_POINT('Ctrl Pts',(37.640684225183,-31.02531860735,9.17720357755709));
#8020=CARTESIAN_POINT('Ctrl Pts',(37.4884095532307,-30.5112368586177,9.14489344002454));
#8021=CARTESIAN_POINT('Ctrl Pts',(37.4857778982365,-29.998587099551,9.11258330249199));
#8022=CARTESIAN_POINT('Origin',(40.,30.,12.2084234471775));
#8023=CARTESIAN_POINT('',(36.9214104210795,30.0001481134795,0.791576552822544));
#8024=CARTESIAN_POINT('',(36.9314435342158,30.0007393170824,0.708423447177453));
#8025=CARTESIAN_POINT('',(36.9265,30.0000000000001,12.2084234471775));
#8026=CARTESIAN_POINT('',(40.7937992825328,27.0307770462543,0.));
#8027=CARTESIAN_POINT('Ctrl Pts',(36.9314435342158,30.0007393170824,0.708423447177453));
#8028=CARTESIAN_POINT('Ctrl Pts',(36.9305908971901,30.4743000521285,0.68399525708588));
#8029=CARTESIAN_POINT('Ctrl Pts',(37.2564683870193,31.9726985654157,0.606638827252413));
#8030=CARTESIAN_POINT('Ctrl Pts',(39.5908855572201,33.609027296031,0.47635415767705));
#8031=CARTESIAN_POINT('Ctrl Pts',(42.8129709591412,32.3023681766822,0.317569438451369));
#8032=CARTESIAN_POINT('Ctrl Pts',(43.4548287867864,28.8815849473274,0.158784719225683));
#8033=CARTESIAN_POINT('Ctrl Pts',(41.7812379463276,27.2947612990625,0.0529282397418946));
#8034=CARTESIAN_POINT('Ctrl Pts',(40.7937992825328,27.0307770462543,0.));
#8035=CARTESIAN_POINT('',(39.2062007174671,27.0307770462543,0.));
#8036=CARTESIAN_POINT('Origin',(40.,30.,0.));
#8037=CARTESIAN_POINT('Ctrl Pts',(36.9214104210795,30.0001481134795,0.791576552822544));
#8038=CARTESIAN_POINT('Ctrl Pts',(36.9214060852395,30.0071343339544,0.791213130185148));
#8039=CARTESIAN_POINT('Ctrl Pts',(36.9245904926899,31.0315771191332,0.737921467805857));
#8040=CARTESIAN_POINT('Ctrl Pts',(38.0509704657541,33.0656996094815,0.631701565684668));
#8041=CARTESIAN_POINT('Ctrl Pts',(41.5191020833988,33.300338163167,0.472916846458987));
#8042=CARTESIAN_POINT('Ctrl Pts',(43.5964449208384,30.5125900673602,0.314132127233303));
#8043=CARTESIAN_POINT('Ctrl Pts',(42.3902201567819,27.281023587038,0.15649317841364));
#8044=CARTESIAN_POINT('Ctrl Pts',(40.1666400375141,26.7696589897829,0.0517824693358737));
#8045=CARTESIAN_POINT('Ctrl Pts',(39.2044526546617,27.0254683880106,-4.06575814682064E-18));
#8046=CARTESIAN_POINT('Origin',(40.,30.,12.2084234471775));
#8047=CARTESIAN_POINT('',(36.9285654760686,30.0025993155776,1.79157655282254));
#8048=CARTESIAN_POINT('',(36.9266847216198,29.9971878060927,1.70842344717745));
#8049=CARTESIAN_POINT('',(36.9265,30.0000000000001,12.2084234471775));
#8050=CARTESIAN_POINT('Ctrl Pts',(36.9266847216198,29.9971878060927,1.70842344717745));
#8051=CARTESIAN_POINT('Ctrl Pts',(36.9337736898222,30.7732902078871,1.66823136220391));
#8052=CARTESIAN_POINT('Ctrl Pts',(37.6258961169519,32.5826850742956,1.57511103748848));
#8053=CARTESIAN_POINT('Ctrl Pts',(40.6663949910499,33.5712523754168,1.42906247303115));
#8054=CARTESIAN_POINT('Ctrl Pts',(43.3620055739433,31.3766529896116,1.27027775380547));
#8055=CARTESIAN_POINT('Ctrl Pts',(42.9796780358998,27.9216547954996,1.11149303457979));
#8056=CARTESIAN_POINT('Ctrl Pts',(39.8696594013047,26.3695385472464,0.952708315354102));
#8057=CARTESIAN_POINT('Ctrl Pts',(37.3388060344315,27.8681888840249,0.81835178621999));
#8058=CARTESIAN_POINT('Ctrl Pts',(36.9324382946739,29.448242205726,0.736923496827775));
#8059=CARTESIAN_POINT('Ctrl Pts',(36.9314435342158,30.0007393170824,0.708423447177453));
#8060=CARTESIAN_POINT('Ctrl Pts',(36.9285654760686,30.0025993155776,1.79157655282254));
#8061=CARTESIAN_POINT('Ctrl Pts',(36.9260623773303,30.3144991191654,1.77544923530318));
#8062=CARTESIAN_POINT('Ctrl Pts',(37.1131652421759,31.6470901191891,1.70639367804192));
#8063=CARTESIAN_POINT('Ctrl Pts',(39.0340361139851,33.5021320828999,1.58440988103877));
#8064=CARTESIAN_POINT('Ctrl Pts',(42.4187332816925,32.7106797239938,1.42562516181309));
#8065=CARTESIAN_POINT('Ctrl Pts',(43.5891188868934,29.4376293695436,1.2668404425874));
#8066=CARTESIAN_POINT('Ctrl Pts',(41.4737278337939,26.6794509596774,1.10805572336172));
#8067=CARTESIAN_POINT('Ctrl Pts',(38.0170881375389,26.9604739257629,0.949634426773431));
#8068=CARTESIAN_POINT('Ctrl Pts',(36.9220375494226,28.9896733556398,0.844141369927042));
#8069=CARTESIAN_POINT('Ctrl Pts',(36.9214104210795,30.0001481134795,0.791576552822544));
#8070=CARTESIAN_POINT('Origin',(40.,30.,12.2084234471775));
#8071=CARTESIAN_POINT('',(36.9306301640296,29.9983760595424,2.79157655282254));
#8072=CARTESIAN_POINT('',(36.9218442521368,30.001056467914,2.70842344717745));
#8073=CARTESIAN_POINT('',(36.9265,30.0000000000001,12.2084234471775));
#8074=CARTESIAN_POINT('Ctrl Pts',(36.9218442521368,30.001056467914,2.70842344717745));
#8075=CARTESIAN_POINT('Ctrl Pts',(36.9215847759613,30.0592829556301,2.70539570706384));
#8076=CARTESIAN_POINT('Ctrl Pts',(36.9494734222224,31.1351192558441,2.64943972720834));
#8077=CARTESIAN_POINT('Ctrl Pts',(38.2073434453337,33.1598130705237,2.54055550761094));
#8078=CARTESIAN_POINT('Ctrl Pts',(41.6828293076519,33.2196458493402,2.38177078838525));
#8079=CARTESIAN_POINT('Ctrl Pts',(43.6177133488499,30.3319467933355,2.22298606915957));
#8080=CARTESIAN_POINT('Ctrl Pts',(42.2406393602062,27.1403544247083,2.06420134993389));
#8081=CARTESIAN_POINT('Ctrl Pts',(38.8122994891743,26.5667233512227,1.9054166307082));
#8082=CARTESIAN_POINT('Ctrl Pts',(37.0638424029061,28.4858017899762,1.78682399645606));
#8083=CARTESIAN_POINT('Ctrl Pts',(36.9244383540519,29.7512547993364,1.72115960194581));
#8084=CARTESIAN_POINT('Ctrl Pts',(36.9266847216198,29.9971878060927,1.70842344717745));
#8085=CARTESIAN_POINT('Ctrl Pts',(36.9306301640296,29.9983760595424,2.79157655282254));
#8086=CARTESIAN_POINT('Ctrl Pts',(36.9335903506277,30.61619128252,2.75968534042121));
#8087=CARTESIAN_POINT('Ctrl Pts',(37.4143806753803,32.2636022177905,2.67486588827799));
#8088=CARTESIAN_POINT('Ctrl Pts',(40.1017542133218,33.6314839980979,2.53711819639287));
#8089=CARTESIAN_POINT('Ctrl Pts',(43.1063930447263,31.883707179614,2.37833347716719));
#8090=CARTESIAN_POINT('Ctrl Pts',(43.2671803398556,28.4114273111418,2.21954875794151));
#8091=CARTESIAN_POINT('Ctrl Pts',(40.4369180427711,26.3934599853152,2.06076403871582));
#8092=CARTESIAN_POINT('Ctrl Pts',(37.5347521985174,27.5468316477252,1.9181066370095));
#8093=CARTESIAN_POINT('Ctrl Pts',(36.9342772965169,29.2908752238756,1.82837747504508));
#8094=CARTESIAN_POINT('Ctrl Pts',(36.9285654760686,30.0025993155776,1.79157655282254));
#8095=CARTESIAN_POINT('Origin',(40.,30.,12.2084234471775));
#8096=CARTESIAN_POINT('',(36.9226404245075,29.9982621359517,3.79157655282254));
#8097=CARTESIAN_POINT('',(36.9298121415154,30.0021532465789,3.70842344717745));
#8098=CARTESIAN_POINT('',(36.9265,30.0000000000001,12.2084234471775));
#8099=CARTESIAN_POINT('Ctrl Pts',(36.9298121415154,30.0021532465789,3.70842344717745));
#8100=CARTESIAN_POINT('Ctrl Pts',(36.9274611424663,30.3659528285612,3.68963181218188));
#8101=CARTESIAN_POINT('Ctrl Pts',(37.1555525490304,31.7515729915281,3.61791193744441));
#8102=CARTESIAN_POINT('Ctrl Pts',(39.2110614856976,33.5462109122232,3.49326382296504));
#8103=CARTESIAN_POINT('Ctrl Pts',(42.551760057577,32.5858376556528,3.33447910373935));
#8104=CARTESIAN_POINT('Ctrl Pts',(43.5563644593613,29.2581727531378,3.17569438451367));
#8105=CARTESIAN_POINT('Ctrl Pts',(41.3051759276346,26.6096384170271,3.01690966528799));
#8106=CARTESIAN_POINT('Ctrl Pts',(37.9248305372375,27.0562426682318,2.86115268617592));
#8107=CARTESIAN_POINT('Ctrl Pts',(36.9261207059647,29.0414196696403,2.75832394680574));
#8108=CARTESIAN_POINT('Ctrl Pts',(36.9218442521368,30.001056467914,2.70842344717745));
#8109=CARTESIAN_POINT('Ctrl Pts',(36.9226404245075,29.9982621359517,3.79157655282254));
#8110=CARTESIAN_POINT('Ctrl Pts',(36.9288449239179,30.91534466323,3.74392144553925));
#8111=CARTESIAN_POINT('Ctrl Pts',(37.8505480972411,32.8618102457237,3.64333809851406));
#8112=CARTESIAN_POINT('Ctrl Pts',(41.1605538126502,33.4425492067914,3.48982651174697));
#8113=CARTESIAN_POINT('Ctrl Pts',(43.5217905842841,30.8916396581577,3.33104179252129));
#8114=CARTESIAN_POINT('Ctrl Pts',(42.6588862528215,27.5244487277861,3.17225707329561));
#8115=CARTESIAN_POINT('Ctrl Pts',(39.3618154801332,26.4235841007334,3.01347235406992));
#8116=CARTESIAN_POINT('Ctrl Pts',(37.1938507363835,28.1603743953028,2.88657884724557));
#8117=CARTESIAN_POINT('Ctrl Pts',(36.9286774779537,29.5908344592533,2.81261358016311));
#8118=CARTESIAN_POINT('Ctrl Pts',(36.9306301640296,29.9983760595424,2.79157655282254));
#8119=CARTESIAN_POINT('Origin',(40.,30.,12.2084234471775));
#8120=CARTESIAN_POINT('',(36.9253702239752,30.0027105193813,4.79157655282255));
#8121=CARTESIAN_POINT('',(36.9296341594976,29.9977623726118,4.70842344717745));
#8122=CARTESIAN_POINT('',(36.9265,30.0000000000001,12.2084234471775));
#8123=CARTESIAN_POINT('Ctrl Pts',(36.9296341594976,29.9977623726118,4.70842344717745));
#8124=CARTESIAN_POINT('Ctrl Pts',(36.9341435373618,30.6666480454017,4.67386791729991));
#8125=CARTESIAN_POINT('Ctrl Pts',(37.4780313316422,32.3667321797224,4.58638414768047));
#8126=CARTESIAN_POINT('Ctrl Pts',(40.2839268182445,33.6217980846202,4.44597213831914));
#8127=CARTESIAN_POINT('Ctrl Pts',(43.1970393894843,31.7253912441272,4.28718741909346));
#8128=CARTESIAN_POINT('Ctrl Pts',(43.1833152122909,28.2494172218816,4.12840269986777));
#8129=CARTESIAN_POINT('Ctrl Pts',(40.255318543719,26.3760728144276,3.96961798064209));
#8130=CARTESIAN_POINT('Ctrl Pts',(37.4677628071963,27.6494457306752,3.82962489641198));
#8131=CARTESIAN_POINT('Ctrl Pts',(36.9340829314343,29.3412803347791,3.74256005192377));
#8132=CARTESIAN_POINT('Ctrl Pts',(36.9298121415154,30.0021532465789,3.70842344717745));
#8133=CARTESIAN_POINT('Ctrl Pts',(36.9253702239752,30.0027105193813,4.79157655282255));
#8134=CARTESIAN_POINT('Ctrl Pts',(36.9235103917928,30.2050629564242,4.78108579039918));
#8135=CARTESIAN_POINT('Ctrl Pts',(37.0339430833948,31.4263085444825,4.71766678823391));
#8136=CARTESIAN_POINT('Ctrl Pts',(38.6680931462871,33.3799488650141,4.60131954632676));
#8137=CARTESIAN_POINT('Ctrl Pts',(42.1176356506926,32.9518891320487,4.44253482710108));
#8138=CARTESIAN_POINT('Ctrl Pts',(43.6285176985082,29.8214236615297,4.28375010787539));
#8139=CARTESIAN_POINT('Ctrl Pts',(41.8175517334939,26.8544418788833,4.1249653886497));
#8140=CARTESIAN_POINT('Ctrl Pts',(38.3426471809504,26.7671665941811,3.96618066942403));
#8141=CARTESIAN_POINT('Ctrl Pts',(36.9725521563655,28.7774415912537,3.85505105748164));
#8142=CARTESIAN_POINT('Ctrl Pts',(36.9219538843002,29.8967851292364,3.79684968528114));
#8143=CARTESIAN_POINT('Ctrl Pts',(36.9226404245075,29.9982621359517,3.79157655282254));
#8144=CARTESIAN_POINT('Origin',(40.,30.,12.2084234471775));
#8145=CARTESIAN_POINT('',(36.9314878993762,30.0000666771347,5.79157655282255));
#8146=CARTESIAN_POINT('',(36.9217350264198,29.9990828880962,5.70842344717746));
#8147=CARTESIAN_POINT('',(36.9265,30.0000000000001,12.2084234471775));
#8148=CARTESIAN_POINT('Ctrl Pts',(36.9217350264198,29.9990828880962,5.70842344717746));
#8149=CARTESIAN_POINT('Ctrl Pts',(36.925541226593,30.966684508532,5.65810402241795));
#8150=CARTESIAN_POINT('Ctrl Pts',(37.9390395048434,32.9589227335458,5.55485635791654));
#8151=CARTESIAN_POINT('Ctrl Pts',(41.3319071366153,33.3799495829286,5.39868045367324));
#8152=CARTESIAN_POINT('Ctrl Pts',(43.562111392168,30.7137213976436,5.23989573444756));
#8153=CARTESIAN_POINT('Ctrl Pts',(42.5312615113734,27.3940930629228,5.08111101522188));
#8154=CARTESIAN_POINT('Ctrl Pts',(39.1830835312918,26.4601294816251,4.92232629599619));
#8155=CARTESIAN_POINT('Ctrl Pts',(37.1486704266839,28.2648568201031,4.79809710664805));
#8156=CARTESIAN_POINT('Ctrl Pts',(36.9272365840166,29.6421248685093,4.7267961570418));
#8157=CARTESIAN_POINT('Ctrl Pts',(36.9296341594976,29.9977623726118,4.70842344717745));
#8158=CARTESIAN_POINT('Ctrl Pts',(36.9314878993762,30.0000666771347,5.79157655282255));
#8159=CARTESIAN_POINT('Ctrl Pts',(36.9313894343278,30.5090425915801,5.76532189551722));
#8160=CARTESIAN_POINT('Ctrl Pts',(37.2923228112074,32.0439602821561,5.68613899846999));
#8161=CARTESIAN_POINT('Ctrl Pts',(39.7160732420625,33.6217973153363,5.55402786168086));
#8162=CARTESIAN_POINT('Ctrl Pts',(42.8891154512744,32.2025081398842,5.39524314245518));
#8163=CARTESIAN_POINT('Ctrl Pts',(43.4172201906419,28.7668591460577,5.23645842322949));
#8164=CARTESIAN_POINT('Ctrl Pts',(40.8169162951919,26.4601302335076,5.07767370400381));
#8165=CARTESIAN_POINT('Ctrl Pts',(37.6899500625198,27.3323875025768,4.92937974720149));
#8166=CARTESIAN_POINT('Ctrl Pts',(36.9328936605827,29.1841497121866,4.83401403014107));
#8167=CARTESIAN_POINT('Ctrl Pts',(36.9253702239752,30.0027105193813,4.79157655282255));
#8168=CARTESIAN_POINT('Origin',(40.,30.,12.2084234471775));
#8169=CARTESIAN_POINT('',(36.9256150573553,29.9972554300884,6.79157655282254));
#8170=CARTESIAN_POINT('',(36.926927637137,30.0028093909042,6.70842344717746));
#8171=CARTESIAN_POINT('',(36.9265,30.0000000000001,12.2084234471775));
#8172=CARTESIAN_POINT('Ctrl Pts',(36.926927637137,30.0028093909042,6.70842344717746));
#8173=CARTESIAN_POINT('Ctrl Pts',(36.9246261470968,30.2568826318381,6.69526836727787));
#8174=CARTESIAN_POINT('Ctrl Pts',(37.0696627317,31.5306040707075,6.6291850476364));
#8175=CARTESIAN_POINT('Ctrl Pts',(38.8394459408439,33.4425499380084,6.51017348825303));
#8176=CARTESIAN_POINT('Ctrl Pts',(42.2631512836135,32.8418624302693,6.35138876902734));
#8177=CARTESIAN_POINT('Ctrl Pts',(43.6149790117272,29.6394968119162,6.19260404980166));
#8178=CARTESIAN_POINT('Ctrl Pts',(41.657353171078,26.7671659075135,6.03381933057598));
#8179=CARTESIAN_POINT('Ctrl Pts',(38.1824478804507,26.8544412107546,5.87503461135029));
#8180=CARTESIAN_POINT('Ctrl Pts',(36.9453830083193,28.8811766715375,5.76656931688412));
#8181=CARTESIAN_POINT('Ctrl Pts',(36.9215376936385,29.9489174973662,5.71103226215984));
#8182=CARTESIAN_POINT('Ctrl Pts',(36.9217350264198,29.9990828880962,5.70842344717746));
#8183=CARTESIAN_POINT('Ctrl Pts',(36.9256150573553,29.9972554300884,6.79157655282254));
#8184=CARTESIAN_POINT('Ctrl Pts',(36.9330938990886,30.8079017788323,6.74955800063525));
#8185=CARTESIAN_POINT('Ctrl Pts',(37.6777711979151,32.6518218559865,6.65461120870606));
#8186=CARTESIAN_POINT('Ctrl Pts',(40.7889383467181,33.5462101590121,6.50673617703496));
#8187=CARTESIAN_POINT('Ctrl Pts',(43.4073761900399,31.2600863855708,6.34795145780928));
#8188=CARTESIAN_POINT('Ctrl Pts',(42.9064174160314,27.8203743447495,6.1891667385836));
#8189=CARTESIAN_POINT('Ctrl Pts',(39.7446815105131,26.3760735841615,6.03038201935791));
#8190=CARTESIAN_POINT('Ctrl Pts',(37.3008223075735,27.9396648339668,5.89785195743756));
#8191=CARTESIAN_POINT('Ctrl Pts',(36.9315879355548,29.4829694301855,5.81825013525911));
#8192=CARTESIAN_POINT('Ctrl Pts',(36.9314878993762,30.0000666771347,5.79157655282255));
#8193=CARTESIAN_POINT('Origin',(40.,30.,12.2084234471775));
#8194=CARTESIAN_POINT('',(36.9224678986813,30.0016204990256,7.79157655282255));
#8195=CARTESIAN_POINT('',(36.9313094744419,29.9992281658451,7.70842344717746));
#8196=CARTESIAN_POINT('',(36.9265,30.0000000000001,12.2084234471775));
#8197=CARTESIAN_POINT('Ctrl Pts',(36.9313094744419,29.9992281658452,7.70842344717746));
#8198=CARTESIAN_POINT('Ctrl Pts',(36.9325689694722,30.5597739580728,7.67950447239591));
#8199=CARTESIAN_POINT('Ctrl Pts',(37.347926997611,32.1479826672757,7.59765725787247));
#8200=CARTESIAN_POINT('Ctrl Pts',(39.8982457650928,33.6314847697161,7.46288180360713));
#8201=CARTESIAN_POINT('Ctrl Pts',(42.9960395463676,32.0546977641436,7.30409708438144));
#8202=CARTESIAN_POINT('Ctrl Pts',(43.3510086198694,28.5968688366528,7.14531236515576));
#8203=CARTESIAN_POINT('Ctrl Pts',(40.6381846554167,26.4235833410482,6.98652764593007));
#8204=CARTESIAN_POINT('Ctrl Pts',(37.6142706932541,27.4332431712104,6.84089800660398));
#8205=CARTESIAN_POINT('Ctrl Pts',(36.933885978093,29.2346425914276,6.74819660701977));
#8206=CARTESIAN_POINT('Ctrl Pts',(36.926927637137,30.0028093909042,6.70842344717746));
#8207=CARTESIAN_POINT('Ctrl Pts',(36.9224678986813,30.0016204990256,7.79157655282255));
#8208=CARTESIAN_POINT('Ctrl Pts',(36.9218704635921,30.0950218610504,7.78672234549518));
#8209=CARTESIAN_POINT('Ctrl Pts',(36.9680973053051,31.2062330488769,7.72893989842591));
#8210=CARTESIAN_POINT('Ctrl Pts',(38.3171710506372,33.2196451638042,7.61822921161474));
#8211=CARTESIAN_POINT('Ctrl Pts',(41.7926561734374,33.159812400248,7.45944449238906));
#8212=CARTESIAN_POINT('Ctrl Pts',(43.6269944901785,30.207223201086,7.30065977316338));
#8213=CARTESIAN_POINT('Ctrl Pts',(42.1408791121553,27.0649247751536,7.14187505393769));
#8214=CARTESIAN_POINT('Ctrl Pts',(38.6948243496615,26.6096391370258,6.98309033471202));
#8215=CARTESIAN_POINT('Ctrl Pts',(37.0393590026679,28.5573022279082,6.86632416767362));
#8216=CARTESIAN_POINT('Ctrl Pts',(36.9236732525493,29.7867793922029,6.80248624037714));
#8217=CARTESIAN_POINT('Ctrl Pts',(36.9256150573553,29.9972554300884,6.79157655282254));
#8218=CARTESIAN_POINT('Origin',(40.,30.,12.2084234471775));
#8219=CARTESIAN_POINT('',(36.9305016190506,30.0017249535699,8.79157655282255));
#8220=CARTESIAN_POINT('',(36.9240970871575,29.9975851957844,8.70842344717746));
#8221=CARTESIAN_POINT('',(36.9265,30.0000000000001,12.2084234471775));
#8222=CARTESIAN_POINT('Ctrl Pts',(36.9240970871575,29.9975851957844,8.70842344717746));
#8223=CARTESIAN_POINT('Ctrl Pts',(36.9315169131983,30.8585346510502,8.66374057751394));
#8224=CARTESIAN_POINT('Ctrl Pts',(37.7570267321285,32.7517788120336,8.56612946810854));
#8225=CARTESIAN_POINT('Ctrl Pts',(40.9659640933653,33.5021328388261,8.41559011896122));
#8226=CARTESIAN_POINT('Ctrl Pts',(43.4663372079312,31.0874483526599,8.25680539973555));
#8227=CARTESIAN_POINT('Ctrl Pts',(42.7933361741705,27.6772190016871,8.09802068050986));
#8228=CARTESIAN_POINT('Ctrl Pts',(39.5630818641794,26.3934592174139,7.93923596128418));
#8229=CARTESIAN_POINT('Ctrl Pts',(37.2482860828349,28.0439006852296,7.80937021684004));
#8230=CARTESIAN_POINT('Ctrl Pts',(36.930263809783,29.5338488586718,7.7324327121378));
#8231=CARTESIAN_POINT('Ctrl Pts',(36.9313094744419,29.9992281658452,7.70842344717746));
#8232=CARTESIAN_POINT('Ctrl Pts',(36.9305016190507,30.0017249535699,8.79157655282255));
#8233=CARTESIAN_POINT('Ctrl Pts',(36.9284513914002,30.4011123899437,8.77095845061321));
#8234=CARTESIAN_POINT('Ctrl Pts',(37.1865084098534,31.8232183849388,8.69741210866198));
#8235=CARTESIAN_POINT('Ctrl Pts',(39.3336051768584,33.5712515449036,8.57093752696884));
#8236=CARTESIAN_POINT('Ctrl Pts',(42.63924979695,32.4964766410994,8.41215280774317));
#8237=CARTESIAN_POINT('Ctrl Pts',(43.5287243142158,29.1361944846783,8.25336808851748));
#8238=CARTESIAN_POINT('Ctrl Pts',(41.1877002535156,26.5667240916348,8.0945833692918));
#8239=CARTESIAN_POINT('Ctrl Pts',(37.864168867224,27.12281855603,7.94065285739348));
#8240=CARTESIAN_POINT('Ctrl Pts',(36.9283846451053,29.0766126032515,7.83965058523707));
#8241=CARTESIAN_POINT('Ctrl Pts',(36.9224678986813,30.0016204990256,7.79157655282255));
#8242=CARTESIAN_POINT('Origin',(40.,30.,12.2084234471775));
#8243=CARTESIAN_POINT('',(36.9295987310864,29.9965353802945,9.79157655282255));
#8244=CARTESIAN_POINT('',(36.9237140680981,30.0022179367619,9.70842344717746));
#8245=CARTESIAN_POINT('',(36.9265,30.0000000000001,12.2084234471775));
#8246=CARTESIAN_POINT('',(39.2062007174671,27.0307770462543,10.));
#8247=CARTESIAN_POINT('Ctrl Pts',(39.2062007174671,27.0307770462543,10.));
#8248=CARTESIAN_POINT('Ctrl Pts',(38.2187620536724,27.2947612990625,9.94707176025811));
#8249=CARTESIAN_POINT('Ctrl Pts',(37.1203696025755,28.3362007046644,9.87759727786562));
#8250=CARTESIAN_POINT('Ctrl Pts',(36.9271780976658,29.6764519122675,9.80812279547314));
#8251=CARTESIAN_POINT('Ctrl Pts',(36.9295987310864,29.9965353802945,9.79157655282255));
#8252=CARTESIAN_POINT('',(40.7955467101491,27.0254727950732,10.));
#8253=CARTESIAN_POINT('Origin',(40.,30.,10.));
#8254=CARTESIAN_POINT('Ctrl Pts',(40.7955481281091,27.0254684909089,10.));
#8255=CARTESIAN_POINT('Ctrl Pts',(39.8333613752542,26.7696596878221,9.94821753066413));
#8256=CARTESIAN_POINT('Ctrl Pts',(37.7694374933144,27.2443038752448,9.85102534638994));
#8257=CARTESIAN_POINT('Ctrl Pts',(36.9309454989351,29.1277455385835,9.75383316211576));
#8258=CARTESIAN_POINT('Ctrl Pts',(36.9237140680981,30.0022179367619,9.70842344717746));
#8259=CARTESIAN_POINT('Origin',(-40.,30.,12.2084234471774));
#8260=CARTESIAN_POINT('',(-43.0785897715144,30.0001480928245,0.791576552822542));
#8261=CARTESIAN_POINT('',(-43.0685559416288,30.0007395458647,0.708423447177451));
#8262=CARTESIAN_POINT('',(-43.0735,30.0000000000001,12.2084234471774));
#8263=CARTESIAN_POINT('',(-39.2062007174671,27.0307770462543,0.));
#8264=CARTESIAN_POINT('Ctrl Pts',(-43.0685559416287,30.0007395458647,0.708423447177451));
#8265=CARTESIAN_POINT('Ctrl Pts',(-43.0694085603479,30.4743003164273,0.683995257085879));
#8266=CARTESIAN_POINT('Ctrl Pts',(-42.7435310628009,31.9726987925452,0.606638827252412));
#8267=CARTESIAN_POINT('Ctrl Pts',(-40.4091143183855,33.6090247272076,0.476354157677051));
#8268=CARTESIAN_POINT('Ctrl Pts',(-37.1870300541988,32.3023712386336,0.317569438451368));
#8269=CARTESIAN_POINT('Ctrl Pts',(-36.5451700500256,28.8815775163836,0.158784719225683));
#8270=CARTESIAN_POINT('Ctrl Pts',(-38.2187620536724,27.2947612990625,0.0529282397418946));
#8271=CARTESIAN_POINT('Ctrl Pts',(-39.2062007174671,27.0307770462543,0.));
#8272=CARTESIAN_POINT('',(-40.7937992825329,27.0307770462543,0.));
#8273=CARTESIAN_POINT('Origin',(-40.,30.,0.));
#8274=CARTESIAN_POINT('Ctrl Pts',(-43.0785897715144,30.0001480928245,0.791576552822542));
#8275=CARTESIAN_POINT('Ctrl Pts',(-43.0785941073969,30.0071343138444,0.791213130185146));
#8276=CARTESIAN_POINT('Ctrl Pts',(-43.0754097060638,31.0315771792942,0.737921467805855));
#8277=CARTESIAN_POINT('Ctrl Pts',(-41.9490297104332,33.065699934597,0.63170156568467));
#8278=CARTESIAN_POINT('Ctrl Pts',(-38.4808977151712,33.3003381572967,0.472916846458986));
#8279=CARTESIAN_POINT('Ctrl Pts',(-36.4035550591505,30.5125904676491,0.314132127233303));
#8280=CARTESIAN_POINT('Ctrl Pts',(-37.6097792569612,27.2810228199895,0.156493178413639));
#8281=CARTESIAN_POINT('Ctrl Pts',(-39.8333603928249,26.7696592028777,0.0517824693358729));
#8282=CARTESIAN_POINT('Ctrl Pts',(-40.7955475841208,27.0254684201926,2.94089839286693E-17));
#8283=CARTESIAN_POINT('Origin',(-40.,30.,12.2084234471774));
#8284=CARTESIAN_POINT('',(-43.0714347220705,30.0025993151568,1.79157655282254));
#8285=CARTESIAN_POINT('',(-43.0733147540399,29.9971878064111,1.70842344717745));
#8286=CARTESIAN_POINT('',(-43.0735,30.0000000000001,12.2084234471774));
#8287=CARTESIAN_POINT('Ctrl Pts',(-43.0733147540399,29.9971878064111,1.70842344717745));
#8288=CARTESIAN_POINT('Ctrl Pts',(-43.0662257847241,30.773290081476,1.66823136220391));
#8289=CARTESIAN_POINT('Ctrl Pts',(-42.3741034680082,32.5826846574708,1.57511103748848));
#8290=CARTESIAN_POINT('Ctrl Pts',(-39.3336051438857,33.5712517079766,1.42906247303115));
#8291=CARTESIAN_POINT('Ctrl Pts',(-36.6379949650665,31.3766528609059,1.27027775380547));
#8292=CARTESIAN_POINT('Ctrl Pts',(-37.0203225278291,27.921654956147,1.11149303457979));
#8293=CARTESIAN_POINT('Ctrl Pts',(-40.1303404958339,26.3695395185102,0.952708315354101));
#8294=CARTESIAN_POINT('Ctrl Pts',(-42.66119358551,27.8681887692102,0.818351786219991));
#8295=CARTESIAN_POINT('Ctrl Pts',(-43.0675612025287,29.4482423930718,0.736923496827774));
#8296=CARTESIAN_POINT('Ctrl Pts',(-43.0685559416287,30.0007395458647,0.708423447177451));
#8297=CARTESIAN_POINT('Ctrl Pts',(-43.0714347220705,30.0025993151568,1.79157655282254));
#8298=CARTESIAN_POINT('Ctrl Pts',(-43.0739378209611,30.3144991388018,1.77544923530318));
#8299=CARTESIAN_POINT('Ctrl Pts',(-42.886834944053,31.6470902248259,1.70639367804192));
#8300=CARTESIAN_POINT('Ctrl Pts',(-40.9659639490253,33.5021323126134,1.58440988103877));
#8301=CARTESIAN_POINT('Ctrl Pts',(-37.5812665608262,32.7106798921575,1.42562516181309));
#8302=CARTESIAN_POINT('Ctrl Pts',(-36.4108808842817,29.4376293456934,1.2668404425874));
#8303=CARTESIAN_POINT('Ctrl Pts',(-38.5262720652766,26.679450722727,1.10805572336172));
#8304=CARTESIAN_POINT('Ctrl Pts',(-41.9829120023514,26.9604737702103,0.949634426773434));
#8305=CARTESIAN_POINT('Ctrl Pts',(-43.0779626370196,28.9896732561604,0.84414136992704));
#8306=CARTESIAN_POINT('Ctrl Pts',(-43.0785897715144,30.0001480928245,0.791576552822542));
#8307=CARTESIAN_POINT('Origin',(-40.,30.,12.2084234471774));
#8308=CARTESIAN_POINT('',(-43.0693700340734,29.9983760594323,2.79157655282254));
#8309=CARTESIAN_POINT('',(-43.0781552224421,30.001056467624,2.70842344717745));
#8310=CARTESIAN_POINT('',(-43.0735,30.0000000000001,12.2084234471774));
#8311=CARTESIAN_POINT('Ctrl Pts',(-43.0781552224421,30.001056467624,2.70842344717745));
#8312=CARTESIAN_POINT('Ctrl Pts',(-43.0784146985717,30.0592829454032,2.70539570706384));
#8313=CARTESIAN_POINT('Ctrl Pts',(-43.0505260570341,31.1351190620316,2.64943972720834));
#8314=CARTESIAN_POINT('Ctrl Pts',(-41.7926562482662,33.15981253181,2.54055550761094));
#8315=CARTESIAN_POINT('Ctrl Pts',(-38.3171709803108,33.2196452983643,2.38177078838525));
#8316=CARTESIAN_POINT('Ctrl Pts',(-36.3822872674944,30.3319467392027,2.22298606915957));
#8317=CARTESIAN_POINT('Ctrl Pts',(-37.7593610245569,27.1403549081105,2.06420134993389));
#8318=CARTESIAN_POINT('Ctrl Pts',(-41.1877003040245,26.566723946295,1.9054166307082));
#8319=CARTESIAN_POINT('Ctrl Pts',(-42.9361571001743,28.485802038215,1.78682399645606));
#8320=CARTESIAN_POINT('Ctrl Pts',(-43.0755611219607,29.7512548398132,1.72115960194581));
#8321=CARTESIAN_POINT('Ctrl Pts',(-43.0733147540399,29.9971878064111,1.70842344717745));
#8322=CARTESIAN_POINT('Ctrl Pts',(-43.0693700340734,29.9983760594323,2.79157655282254));
#8323=CARTESIAN_POINT('Ctrl Pts',(-43.0664098472836,30.6161913222782,2.75968534042121));
#8324=CARTESIAN_POINT('Ctrl Pts',(-42.5856194914985,32.2636023638608,2.67486588827799));
#8325=CARTESIAN_POINT('Ctrl Pts',(-39.8982457801193,33.6314842325659,2.53711819639287));
#8326=CARTESIAN_POINT('Ctrl Pts',(-36.893606754763,31.8837073010328,2.37833347716719));
#8327=CARTESIAN_POINT('Ctrl Pts',(-36.7328194493102,28.4114272089134,2.21954875794151));
#8328=CARTESIAN_POINT('Ctrl Pts',(-39.5630819289538,26.3934597519746,2.06076403871582));
#8329=CARTESIAN_POINT('Ctrl Pts',(-42.4652479607273,27.5468314902893,1.9181066370095));
#8330=CARTESIAN_POINT('Ctrl Pts',(-43.0657229012746,29.2908751776861,1.82837747504507));
#8331=CARTESIAN_POINT('Ctrl Pts',(-43.0714347220705,30.0025993151568,1.79157655282254));
#8332=CARTESIAN_POINT('Origin',(-40.,30.,12.2084234471774));
#8333=CARTESIAN_POINT('',(-43.0773597741118,29.9982621358397,3.79157655282254));
#8334=CARTESIAN_POINT('',(-43.0701873343651,30.0021532462092,3.70842344717745));
#8335=CARTESIAN_POINT('',(-43.0735,30.0000000000001,12.2084234471774));
#8336=CARTESIAN_POINT('Ctrl Pts',(-43.0701873343651,30.0021532462092,3.70842344717745));
#8337=CARTESIAN_POINT('Ctrl Pts',(-43.0725383330132,30.3659527660857,3.68963181218187));
#8338=CARTESIAN_POINT('Ctrl Pts',(-42.8444469653874,31.7515726925092,3.6179119374444));
#8339=CARTESIAN_POINT('Ctrl Pts',(-40.7889383796118,33.5462103068538,3.49326382296504));
#8340=CARTESIAN_POINT('Ctrl Pts',(-37.4482403780577,32.585837214189,3.33447910373935));
#8341=CARTESIAN_POINT('Ctrl Pts',(-36.4436361477254,29.2581728798308,3.17569438451368));
#8342=CARTESIAN_POINT('Ctrl Pts',(-38.6948242952332,26.6096389957033,3.01690966528799));
#8343=CARTESIAN_POINT('Ctrl Pts',(-42.0751691084,27.0562431709588,2.86115268617591));
#8344=CARTESIAN_POINT('Ctrl Pts',(-43.0738787693705,29.0414198331205,2.75832394680574));
#8345=CARTESIAN_POINT('Ctrl Pts',(-43.0781552224421,30.001056467624,2.70842344717745));
#8346=CARTESIAN_POINT('Ctrl Pts',(-43.0773597741118,29.9982621358397,3.79157655282254));
#8347=CARTESIAN_POINT('Ctrl Pts',(-43.0711552743009,30.9153447223082,3.74392144553925));
#8348=CARTESIAN_POINT('Ctrl Pts',(-42.149452041489,32.8618104304301,3.64333809851406));
#8349=CARTESIAN_POINT('Ctrl Pts',(-38.8394461124454,33.4425494289825,3.48982651174697));
#8350=CARTESIAN_POINT('Ctrl Pts',(-36.4782091884119,30.8916397157027,3.33104179252129));
#8351=CARTESIAN_POINT('Ctrl Pts',(-37.3411135755689,27.5244485680153,3.17225707329561));
#8352=CARTESIAN_POINT('Ctrl Pts',(-40.6381845610556,26.4235838698918,3.01347235406992));
#8353=CARTESIAN_POINT('Ctrl Pts',(-42.8061494447326,28.1603742765857,2.88657884724557));
#8354=CARTESIAN_POINT('Ctrl Pts',(-43.0713227202757,29.590834432844,2.81261358016311));
#8355=CARTESIAN_POINT('Ctrl Pts',(-43.0693700340734,29.9983760594323,2.79157655282254));
#8356=CARTESIAN_POINT('Origin',(-40.,30.,12.2084234471774));
#8357=CARTESIAN_POINT('',(-43.0746299744679,30.0027105195562,4.79157655282254));
#8358=CARTESIAN_POINT('',(-43.0703653163513,29.9977623729938,4.70842344717746));
#8359=CARTESIAN_POINT('',(-43.0735,30.0000000000001,12.2084234471774));
#8360=CARTESIAN_POINT('Ctrl Pts',(-43.0703653163513,29.9977623729938,4.70842344717746));
#8361=CARTESIAN_POINT('Ctrl Pts',(-43.065855939257,30.6666479315962,4.67386791729991));
#8362=CARTESIAN_POINT('Ctrl Pts',(-42.5219682378253,32.3667317756905,4.58638414768047));
#8363=CARTESIAN_POINT('Ctrl Pts',(-39.7160732302253,33.6217974663328,4.44597213831914));
#8364=CARTESIAN_POINT('Ctrl Pts',(-36.802961156292,31.7253909495801,4.28718741909346));
#8365=CARTESIAN_POINT('Ctrl Pts',(-36.8166853311413,28.2494175207298,4.12840269986777));
#8366=CARTESIAN_POINT('Ctrl Pts',(-39.7446814998683,26.3760734330767,3.96961798064209));
#8367=CARTESIAN_POINT('Ctrl Pts',(-42.5322367605161,27.6494461319484,3.82962489641198));
#8368=CARTESIAN_POINT('Ctrl Pts',(-43.0659165451749,29.3412804472297,3.74256005192377));
#8369=CARTESIAN_POINT('Ctrl Pts',(-43.0701873343651,30.0021532462092,3.70842344717745));
#8370=CARTESIAN_POINT('Ctrl Pts',(-43.0746299744679,30.0027105195562,4.79157655282254));
#8371=CARTESIAN_POINT('Ctrl Pts',(-43.0764898067703,30.2050629696594,4.78108579039918));
#8372=CARTESIAN_POINT('Ctrl Pts',(-42.9660571080408,31.4263086365394,4.71766678823391));
#8373=CARTESIAN_POINT('Ctrl Pts',(-41.331906939677,33.379949083163,4.60131954632676));
#8374=CARTESIAN_POINT('Ctrl Pts',(-37.8823642126307,32.9518893225699,4.44253482710107));
#8375=CARTESIAN_POINT('Ctrl Pts',(-36.3714820672996,29.821423650004,4.2837501078754));
#8376=CARTESIAN_POINT('Ctrl Pts',(-38.1824481491975,26.8544416758625,4.1249653886497));
#8377=CARTESIAN_POINT('Ctrl Pts',(-41.6573529260186,26.767166385527,3.96618066942403));
#8378=CARTESIAN_POINT('Ctrl Pts',(-43.0274480390323,28.7774415123474,3.85505105748164));
#8379=CARTESIAN_POINT('Ctrl Pts',(-43.0780463143633,29.8967851225748,3.79684968528114));
#8380=CARTESIAN_POINT('Ctrl Pts',(-43.0773597741118,29.9982621358397,3.79157655282254));
#8381=CARTESIAN_POINT('Origin',(-40.,30.,12.2084234471774));
#8382=CARTESIAN_POINT('',(-43.0685122986719,30.0000666771389,5.79157655282255));
#8383=CARTESIAN_POINT('',(-43.0782644480807,29.9990828882529,5.70842344717746));
#8384=CARTESIAN_POINT('',(-43.0735,30.0000000000001,12.2084234471774));
#8385=CARTESIAN_POINT('Ctrl Pts',(-43.0782644480807,29.9990828882529,5.70842344717746));
#8386=CARTESIAN_POINT('Ctrl Pts',(-43.0744582485572,30.9666843435066,5.65810402241795));
#8387=CARTESIAN_POINT('Ctrl Pts',(-42.060960143324,32.9589222284193,5.55485635791654));
#8388=CARTESIAN_POINT('Ctrl Pts',(-38.6680930907584,33.3799490059277,5.39868045367324));
#8389=CARTESIAN_POINT('Ctrl Pts',(-36.4378892159304,30.7137212758022,5.23989573444757));
#8390=CARTESIAN_POINT('Ctrl Pts',(-37.4687389207455,27.3940935077848,5.08111101522187));
#8391=CARTESIAN_POINT('Ctrl Pts',(-40.81691632925,26.4601300859267,4.92232629599619));
#8392=CARTESIAN_POINT('Ctrl Pts',(-42.8513290865573,28.2648571163145,4.79809710664805));
#8393=CARTESIAN_POINT('Ctrl Pts',(-43.072762891423,29.6421249296032,4.72679615704181));
#8394=CARTESIAN_POINT('Ctrl Pts',(-43.0703653163513,29.9977623729938,4.70842344717746));
#8395=CARTESIAN_POINT('Ctrl Pts',(-43.0685122986719,30.0000666771389,5.79157655282255));
#8396=CARTESIAN_POINT('Ctrl Pts',(-43.0686107637268,30.5090426244347,5.76532189551721));
#8397=CARTESIAN_POINT('Ctrl Pts',(-42.7076773635519,32.0439604140778,5.68613899846998));
#8398=CARTESIAN_POINT('Ctrl Pts',(-40.2839267762627,33.6217975490946,5.55402786168086));
#8399=CARTESIAN_POINT('Ctrl Pts',(-37.1108843622561,32.2025082820388,5.39524314245517));
#8400=CARTESIAN_POINT('Ctrl Pts',(-36.5827795888035,28.7668590664683,5.2364584232295));
#8401=CARTESIAN_POINT('Ctrl Pts',(-39.1830836520825,26.460130005037,5.07767370400381));
#8402=CARTESIAN_POINT('Ctrl Pts',(-42.3100500865757,27.3323873304035,4.9293797472015));
#8403=CARTESIAN_POINT('Ctrl Pts',(-43.0671065373747,29.1841496595299,4.83401403014107));
#8404=CARTESIAN_POINT('Ctrl Pts',(-43.0746299744679,30.0027105195562,4.79157655282254));
#8405=CARTESIAN_POINT('Origin',(-40.,30.,12.2084234471774));
#8406=CARTESIAN_POINT('',(-43.0743851410682,29.9972554299047,6.79157655282255));
#8407=CARTESIAN_POINT('',(-43.0730718382499,30.0028093904244,6.70842344717745));
#8408=CARTESIAN_POINT('',(-43.0735,30.0000000000001,12.2084234471774));
#8409=CARTESIAN_POINT('Ctrl Pts',(-43.0730718382499,30.0028093904244,6.70842344717745));
#8410=CARTESIAN_POINT('Ctrl Pts',(-43.0753733278971,30.2568825879858,6.69526836727787));
#8411=CARTESIAN_POINT('Ctrl Pts',(-42.9303367680532,31.5306038094191,6.6291850476364));
#8412=CARTESIAN_POINT('Ctrl Pts',(-41.1605538610348,33.4425493503161,6.51017348825302));
#8413=CARTESIAN_POINT('Ctrl Pts',(-37.7368491027356,32.8418619451291,6.35138876902735));
#8414=CARTESIAN_POINT('Ctrl Pts',(-36.3850216053963,29.6394968734575,6.19260404980166));
#8415=CARTESIAN_POINT('Ctrl Pts',(-38.3426471118536,26.7671664594007,6.03381933057598));
#8416=CARTESIAN_POINT('Ctrl Pts',(-41.8175518092695,26.8544417477417,5.87503461135029));
#8417=CARTESIAN_POINT('Ctrl Pts',(-43.0546164702181,28.8811768625351,5.76656931688412));
#8418=CARTESIAN_POINT('Ctrl Pts',(-43.0784617808282,29.9489175060867,5.71103226215984));
#8419=CARTESIAN_POINT('Ctrl Pts',(-43.0782644480807,29.9990828882529,5.70842344717746));
#8420=CARTESIAN_POINT('Ctrl Pts',(-43.0743851410682,29.9972554299047,6.79157655282254));
#8421=CARTESIAN_POINT('Ctrl Pts',(-43.0669062988526,30.8079018309698,6.74955800063525));
#8422=CARTESIAN_POINT('Ctrl Pts',(-42.322228951972,32.6518220271502,6.65461120870605));
#8423=CARTESIAN_POINT('Ctrl Pts',(-39.211061602359,33.5462103878864,6.50673617703497));
#8424=CARTESIAN_POINT('Ctrl Pts',(-36.5926235900426,31.2600864669024,6.34795145780927));
#8425=CARTESIAN_POINT('Ctrl Pts',(-37.0935823963814,27.8203742040704,6.1891667385836));
#8426=CARTESIAN_POINT('Ctrl Pts',(-40.2553185059661,26.3760733502665,6.0303820193579));
#8427=CARTESIAN_POINT('Ctrl Pts',(-42.699177866637,27.9396647009882,5.89785195743756));
#8428=CARTESIAN_POINT('Ctrl Pts',(-43.0684122624869,29.4829693968151,5.81825013525911));
#8429=CARTESIAN_POINT('Ctrl Pts',(-43.0685122986719,30.0000666771389,5.79157655282255));
#8430=CARTESIAN_POINT('Origin',(-40.,30.,12.2084234471774));
#8431=CARTESIAN_POINT('',(-43.0775322998549,30.0016204989515,7.79157655282254));
#8432=CARTESIAN_POINT('',(-43.0686900017157,29.9992281658005,7.70842344717746));
#8433=CARTESIAN_POINT('',(-43.0735,30.0000000000001,12.2084234471774));
#8434=CARTESIAN_POINT('Ctrl Pts',(-43.0686900017157,29.9992281658005,7.70842344717746));
#8435=CARTESIAN_POINT('Ctrl Pts',(-43.0674305068904,30.5597738624267,7.67950447239591));
#8436=CARTESIAN_POINT('Ctrl Pts',(-42.6520725496103,32.1479823009103,7.59765725787247));
#8437=CARTESIAN_POINT('Ctrl Pts',(-40.1017542175585,33.6314841495529,7.46288180360712));
#8438=CARTESIAN_POINT('Ctrl Pts',(-37.0039609650845,32.0546974134971,7.30409708438145));
#8439=CARTESIAN_POINT('Ctrl Pts',(-36.6489919521961,28.596869076124,7.14531236515576));
#8440=CARTESIAN_POINT('Ctrl Pts',(-39.3618154535272,26.4235839516209,6.98652764593008));
#8441=CARTESIAN_POINT('Ctrl Pts',(-42.3857288994719,27.4332436093761,6.84089800660397));
#8442=CARTESIAN_POINT('Ctrl Pts',(-43.066113498482,29.2346427220807,6.74819660701977));
#8443=CARTESIAN_POINT('Ctrl Pts',(-43.0730718382499,30.0028093904244,6.70842344717745));
#8444=CARTESIAN_POINT('Ctrl Pts',(-43.0775322998549,30.0016204989515,7.79157655282254));
#8445=CARTESIAN_POINT('Ctrl Pts',(-43.0781297349685,30.0950218669743,7.78672234549517));
#8446=CARTESIAN_POINT('Ctrl Pts',(-43.0319028901288,31.2062331262121,7.72893989842591));
#8447=CARTESIAN_POINT('Ctrl Pts',(-41.6828290582353,33.2196453721168,7.61822921161475));
#8448=CARTESIAN_POINT('Ctrl Pts',(-38.20734371072,33.1598126039199,7.45944449238906));
#8449=CARTESIAN_POINT('Ctrl Pts',(-36.3730052758037,30.2072232146022,7.30065977316339));
#8450=CARTESIAN_POINT('Ctrl Pts',(-37.859120749627,27.0649245856435,7.14187505393769));
#8451=CARTESIAN_POINT('Ctrl Pts',(-41.305175734599,26.6096389182437,6.98309033471202));
#8452=CARTESIAN_POINT('Ctrl Pts',(-42.9606411884153,28.5573021347888,6.86632416767363));
#8453=CARTESIAN_POINT('Ctrl Pts',(-43.0763269459995,29.7867793784346,6.80248624037714));
#8454=CARTESIAN_POINT('Ctrl Pts',(-43.0743851410682,29.9972554299047,6.79157655282254));
#8455=CARTESIAN_POINT('Origin',(-40.,30.,12.2084234471774));
#8456=CARTESIAN_POINT('',(-43.0694985803644,30.001724961275,8.79157655282255));
#8457=CARTESIAN_POINT('',(-43.0759023900792,29.9975851856081,8.70842344717746));
#8458=CARTESIAN_POINT('',(-43.0735,30.0000000000001,12.2084234471774));
#8459=CARTESIAN_POINT('Ctrl Pts',(-43.0759023900792,29.9975851856081,8.70842344717746));
#8460=CARTESIAN_POINT('Ctrl Pts',(-43.0684825656409,30.8585344935406,8.66374057751394));
#8461=CARTESIAN_POINT('Ctrl Pts',(-42.2429728816432,32.751778358711,8.56612946810854));
#8462=CARTESIAN_POINT('Ctrl Pts',(-39.0340360732831,33.502132231285,8.41559011896122));
#8463=CARTESIAN_POINT('Ctrl Pts',(-36.533663382972,31.0874481722331,8.25680539973555));
#8464=CARTESIAN_POINT('Ctrl Pts',(-37.2066643030969,27.6772193954211,8.09802068050986));
#8465=CARTESIAN_POINT('Ctrl Pts',(-40.4369180610355,26.3934598345883,7.93923596128418));
#8466=CARTESIAN_POINT('Ctrl Pts',(-42.7517134474539,28.0439010187842,7.80937021684004));
#8467=CARTESIAN_POINT('Ctrl Pts',(-43.0697356662044,29.5338489379978,7.7324327121378));
#8468=CARTESIAN_POINT('Ctrl Pts',(-43.0686900017157,29.9992281658005,7.70842344717746));
#8469=CARTESIAN_POINT('Ctrl Pts',(-43.0694985803644,30.001724961275,8.79157655282254));
#8470=CARTESIAN_POINT('Ctrl Pts',(-43.0715488058998,30.4011124160455,8.77095845061321));
#8471=CARTESIAN_POINT('Ctrl Pts',(-42.813491762819,31.8232184749255,8.69741210866198));
#8472=CARTESIAN_POINT('Ctrl Pts',(-40.6663948741839,33.5712517973455,8.57093752696885));
#8473=CARTESIAN_POINT('Ctrl Pts',(-37.3607500279849,32.4964767903705,8.41215280774316));
#8474=CARTESIAN_POINT('Ctrl Pts',(-36.4712754607486,29.1361944352982,8.25336808851748));
#8475=CARTESIAN_POINT('Ctrl Pts',(-38.812299668292,26.5667238666358,8.0945833692918));
#8476=CARTESIAN_POINT('Ctrl Pts',(-42.1358312714109,27.1228183719866,7.94065285739349));
#8477=CARTESIAN_POINT('Ctrl Pts',(-43.0716155531895,29.0766125437756,7.83965058523707));
#8478=CARTESIAN_POINT('Ctrl Pts',(-43.0775322998549,30.0016204989515,7.79157655282254));
#8479=CARTESIAN_POINT('Origin',(-40.,30.,12.2084234471774));
#8480=CARTESIAN_POINT('',(-43.070401160077,29.9965365385191,9.79157655282254));
#8481=CARTESIAN_POINT('',(-43.0762854577871,30.0022177574501,9.70842344717746));
#8482=CARTESIAN_POINT('',(-43.0735,30.0000000000001,12.2084234471774));
#8483=CARTESIAN_POINT('',(-40.7937992825329,27.0307770462543,10.));
#8484=CARTESIAN_POINT('Ctrl Pts',(-40.7937992825329,27.0307770462543,10.));
#8485=CARTESIAN_POINT('Ctrl Pts',(-41.7812379463276,27.2947612990625,9.94707176025811));
#8486=CARTESIAN_POINT('Ctrl Pts',(-42.8796301082842,28.3362025511078,9.87759727786562));
#8487=CARTESIAN_POINT('Ctrl Pts',(-43.0728217505486,29.676453251849,9.80812279547313));
#8488=CARTESIAN_POINT('Ctrl Pts',(-43.070401160077,29.9965365385191,9.79157655282254));
#8489=CARTESIAN_POINT('',(-39.2044539122456,27.0254726963224,10.));
#8490=CARTESIAN_POINT('Origin',(-40.,30.,10.));
#8491=CARTESIAN_POINT('Ctrl Pts',(-39.2044525003272,27.0254684088901,10.));
#8492=CARTESIAN_POINT('Ctrl Pts',(-40.1666397594312,26.7696591275303,9.94821753066413));
#8493=CARTESIAN_POINT('Ctrl Pts',(-42.2305611524612,27.2443057138018,9.85102534638995));
#8494=CARTESIAN_POINT('Ctrl Pts',(-43.069053821799,29.1277457869104,9.75383316211576));
#8495=CARTESIAN_POINT('Ctrl Pts',(-43.0762854577871,30.0022177574501,9.70842344717746));
#8496=CARTESIAN_POINT('Origin',(40.,-30.,12.2084234471775));
#8497=CARTESIAN_POINT('',(36.9214106298517,-29.999851864063,0.791576552822544));
#8498=CARTESIAN_POINT('',(36.9314436920733,-29.9992606141577,0.708423447177453));
#8499=CARTESIAN_POINT('',(36.9265,-29.9999999999999,12.2084234471775));
#8500=CARTESIAN_POINT('',(40.7937992825329,-32.9692229537457,0.));
#8501=CARTESIAN_POINT('Ctrl Pts',(36.9314436920733,-29.9992606141577,0.708423447177453));
#8502=CARTESIAN_POINT('Ctrl Pts',(36.9305910605549,-29.5256998684954,0.68399525708588));
#8503=CARTESIAN_POINT('Ctrl Pts',(37.2564685526814,-28.0273013665652,0.606638827252413));
#8504=CARTESIAN_POINT('Ctrl Pts',(39.5908855945796,-26.390973476394,0.47635415767705));
#8505=CARTESIAN_POINT('Ctrl Pts',(42.8129706543341,-27.6976309032298,0.317569438451368));
#8506=CARTESIAN_POINT('Ctrl Pts',(43.4548291366816,-31.1184172884943,0.158784719225683));
#8507=CARTESIAN_POINT('Ctrl Pts',(41.7812379463276,-32.7052387009375,0.0529282397418946));
#8508=CARTESIAN_POINT('Ctrl Pts',(40.7937992825329,-32.9692229537457,0.));
#8509=CARTESIAN_POINT('',(39.2062007174671,-32.9692229537457,0.));
#8510=CARTESIAN_POINT('Origin',(40.,-30.,0.));
#8511=CARTESIAN_POINT('Ctrl Pts',(36.9214106298517,-29.999851864063,0.791576552822544));
#8512=CARTESIAN_POINT('Ctrl Pts',(36.9214062940579,-29.9928656441791,0.791213130185147));
#8513=CARTESIAN_POINT('Ctrl Pts',(36.9245907081615,-28.9684229460631,0.737921467805856));
#8514=CARTESIAN_POINT('Ctrl Pts',(38.0509706569457,-26.9343007433511,0.63170156568467));
#8515=CARTESIAN_POINT('Ctrl Pts',(41.5191018646847,-26.6996618298828,0.472916846458986));
#8516=CARTESIAN_POINT('Ctrl Pts',(43.5964448997665,-29.4874103675251,0.314132127233304));
#8517=CARTESIAN_POINT('Ctrl Pts',(42.3902195200648,-32.7189755800011,0.15649317841364));
#8518=CARTESIAN_POINT('Ctrl Pts',(40.1666405050975,-33.2303412422155,0.0517824693358737));
#8519=CARTESIAN_POINT('Ctrl Pts',(39.2044529144508,-32.9745316477842,-4.47233396150271E-18));
#8520=CARTESIAN_POINT('Origin',(40.,-30.,12.2084234471775));
#8521=CARTESIAN_POINT('',(36.9285656908778,-29.9974006839639,1.79157655282254));
#8522=CARTESIAN_POINT('',(36.9266848795226,-30.0028121938109,1.70842344717745));
#8523=CARTESIAN_POINT('',(36.9265,-29.9999999999999,12.2084234471775));
#8524=CARTESIAN_POINT('Ctrl Pts',(36.9266848795226,-30.0028121938109,1.70842344717745));
#8525=CARTESIAN_POINT('Ctrl Pts',(36.9337738480587,-29.2267098301857,1.66823136220391));
#8526=CARTESIAN_POINT('Ctrl Pts',(37.6258962419323,-27.4173150512511,1.57511103748848));
#8527=CARTESIAN_POINT('Ctrl Pts',(40.6663949504281,-26.4287478255293,1.42906247303115));
#8528=CARTESIAN_POINT('Ctrl Pts',(43.362005411603,-28.6233470492352,1.27027775380547));
#8529=CARTESIAN_POINT('Ctrl Pts',(42.9796778661648,-32.0783451559703,1.11149303457979));
#8530=CARTESIAN_POINT('Ctrl Pts',(39.869659432244,-33.6304611605218,0.952708315354101));
#8531=CARTESIAN_POINT('Ctrl Pts',(37.3388061489086,-32.1318111502224,0.818351786219991));
#8532=CARTESIAN_POINT('Ctrl Pts',(36.932438446106,-30.5517577378998,0.736923496827775));
#8533=CARTESIAN_POINT('Ctrl Pts',(36.9314436920733,-29.9992606141577,0.708423447177453));
#8534=CARTESIAN_POINT('Ctrl Pts',(36.9285656908778,-29.9974006839639,1.79157655282254));
#8535=CARTESIAN_POINT('Ctrl Pts',(36.9260625923045,-29.6855009021205,1.77544923530318));
#8536=CARTESIAN_POINT('Ctrl Pts',(37.1131654440729,-28.3529099953329,1.70639367804192));
#8537=CARTESIAN_POINT('Ctrl Pts',(39.034036182301,-26.4978681661549,1.58440988103877));
#8538=CARTESIAN_POINT('Ctrl Pts',(42.4187331109537,-27.2893204582939,1.42562516181309));
#8539=CARTESIAN_POINT('Ctrl Pts',(43.5891186388302,-30.5623706046428,1.26684044258741));
#8540=CARTESIAN_POINT('Ctrl Pts',(41.4737277243454,-33.3205487833603,1.10805572336172));
#8541=CARTESIAN_POINT('Ctrl Pts',(38.0170882892501,-33.039525905726,0.949634426773433));
#8542=CARTESIAN_POINT('Ctrl Pts',(36.9220377515051,-31.0103265364098,0.844141369927042));
#8543=CARTESIAN_POINT('Ctrl Pts',(36.9214106298517,-29.999851864063,0.791576552822544));
#8544=CARTESIAN_POINT('Origin',(40.,-30.,12.2084234471775));
#8545=CARTESIAN_POINT('',(36.9306303788003,-30.0016239403382,2.79157655282254));
#8546=CARTESIAN_POINT('',(36.9218444103647,-29.9989435321732,2.70842344717745));
#8547=CARTESIAN_POINT('',(36.9265,-29.9999999999999,12.2084234471775));
#8548=CARTESIAN_POINT('Ctrl Pts',(36.9218444103647,-29.9989435321732,2.70842344717745));
#8549=CARTESIAN_POINT('Ctrl Pts',(36.921584934203,-29.9407170474496,2.70539570706384));
#8550=CARTESIAN_POINT('Ctrl Pts',(36.9494735790417,-28.8648808025215,2.64943972720834));
#8551=CARTESIAN_POINT('Ctrl Pts',(38.2073435376042,-26.840187091708,2.54055550761094));
#8552=CARTESIAN_POINT('Ctrl Pts',(41.682829220934,-26.7803543165819,2.38177078838526));
#8553=CARTESIAN_POINT('Ctrl Pts',(43.61771316324,-29.668053222969,2.22298606915957));
#8554=CARTESIAN_POINT('Ctrl Pts',(42.2406392443386,-32.8596454297127,2.06420134993389));
#8555=CARTESIAN_POINT('Ctrl Pts',(38.8122995514484,-33.4332764695832,1.9054166307082));
#8556=CARTESIAN_POINT('Ctrl Pts',(37.063842552554,-31.5141981352583,1.78682399645606));
#8557=CARTESIAN_POINT('Ctrl Pts',(36.9244385118489,-30.248745188472,1.72115960194581));
#8558=CARTESIAN_POINT('Ctrl Pts',(36.9266848795226,-30.0028121938109,1.70842344717745));
#8559=CARTESIAN_POINT('Ctrl Pts',(36.9306303788003,-30.0016239403382,2.79157655282254));
#8560=CARTESIAN_POINT('Ctrl Pts',(36.9335905651907,-29.3838087605833,2.75968534042121));
#8561=CARTESIAN_POINT('Ctrl Pts',(37.4143808562999,-27.7363979405694,2.67486588827799));
#8562=CARTESIAN_POINT('Ctrl Pts',(40.1017542062109,-26.3685162560978,2.53711819639287));
#8563=CARTESIAN_POINT('Ctrl Pts',(43.1063928273453,-28.1162929520197,2.37833347716719));
#8564=CARTESIAN_POINT('Ctrl Pts',(43.2671801112825,-31.58857257803,2.2195487579415));
#8565=CARTESIAN_POINT('Ctrl Pts',(40.4369180121167,-33.6065397617092,2.06076403871582));
#8566=CARTESIAN_POINT('Ctrl Pts',(37.5347523711613,-32.4531681815965,1.9181066370095));
#8567=CARTESIAN_POINT('Ctrl Pts',(36.9342775109495,-30.7091247260472,1.82837747504507));
#8568=CARTESIAN_POINT('Ctrl Pts',(36.9285656908778,-29.9974006839639,1.79157655282254));
#8569=CARTESIAN_POINT('Origin',(40.,-30.,12.2084234471775));
#8570=CARTESIAN_POINT('',(36.9226406398379,-30.0017378639268,3.79157655282254));
#8571=CARTESIAN_POINT('',(36.9298122993513,-29.9978467535325,3.70842344717745));
#8572=CARTESIAN_POINT('',(36.9265,-29.9999999999999,12.2084234471775));
#8573=CARTESIAN_POINT('Ctrl Pts',(36.9298122993513,-29.9978467535325,3.70842344717745));
#8574=CARTESIAN_POINT('Ctrl Pts',(36.9274613004229,-29.634047190253,3.68963181218188));
#8575=CARTESIAN_POINT('Ctrl Pts',(37.155552695261,-28.2484270985199,3.61791193744441));
#8576=CARTESIAN_POINT('Ctrl Pts',(39.211061526259,-26.4537892700808,3.49326382296504));
#8577=CARTESIAN_POINT('Ctrl Pts',(42.5517599263879,-27.4141624772917,3.33447910373936));
#8578=CARTESIAN_POINT('Ctrl Pts',(43.5563642765403,-30.7418272087093,3.17569438451367));
#8579=CARTESIAN_POINT('Ctrl Pts',(41.3051758605191,-33.3903614087074,3.01690966528799));
#8580=CARTESIAN_POINT('Ctrl Pts',(37.9248306439518,-32.9437571803748,2.86115268617591));
#8581=CARTESIAN_POINT('Ctrl Pts',(36.9261208639649,-30.9585802811283,2.75832394680574));
#8582=CARTESIAN_POINT('Ctrl Pts',(36.9218444103647,-29.9989435321732,2.70842344717745));
#8583=CARTESIAN_POINT('Ctrl Pts',(36.9226406398379,-30.0017378639268,3.79157655282254));
#8584=CARTESIAN_POINT('Ctrl Pts',(36.9288451388142,-29.0846554008188,3.74392144553925));
#8585=CARTESIAN_POINT('Ctrl Pts',(37.8505482476435,-27.1381899545233,3.64333809851406));
#8586=CARTESIAN_POINT('Ctrl Pts',(41.1605537314434,-26.5574510340941,3.48982651174697));
#8587=CARTESIAN_POINT('Ctrl Pts',(43.5217903378555,-29.1083604042289,3.33104179252129));
#8588=CARTESIAN_POINT('Ctrl Pts',(42.6588860667731,-32.4755510990005,3.17225707329561));
#8589=CARTESIAN_POINT('Ctrl Pts',(39.3618155247875,-33.5764156490026,3.01347235406992));
#8590=CARTESIAN_POINT('Ctrl Pts',(37.1938509327382,-31.8396254759918,2.88657884724557));
#8591=CARTESIAN_POINT('Ctrl Pts',(36.9286776928615,-30.4091655121155,2.81261358016311));
#8592=CARTESIAN_POINT('Ctrl Pts',(36.9306303788003,-30.0016239403382,2.79157655282254));
#8593=CARTESIAN_POINT('Origin',(40.,-30.,12.2084234471775));
#8594=CARTESIAN_POINT('',(36.9253704391146,-29.9972894808084,4.79157655282255));
#8595=CARTESIAN_POINT('',(36.929634317343,-30.0022376272732,4.70842344717745));
#8596=CARTESIAN_POINT('',(36.9265,-29.9999999999999,12.2084234471775));
#8597=CARTESIAN_POINT('Ctrl Pts',(36.929634317343,-30.0022376272731,4.70842344717745));
#8598=CARTESIAN_POINT('Ctrl Pts',(36.9341436949753,-29.3333519888702,4.67386791729991));
#8599=CARTESIAN_POINT('Ctrl Pts',(37.4780314612948,-27.6332679419497,4.58638414768048));
#8600=CARTESIAN_POINT('Ctrl Pts',(40.2839268036481,-26.3782021015739,4.44597213831914));
#8601=CARTESIAN_POINT('Ctrl Pts',(43.1970392251266,-28.2746088445741,4.28718741909346));
#8602=CARTESIAN_POINT('Ctrl Pts',(43.1833150486392,-31.7505826881217,4.12840269986777));
#8603=CARTESIAN_POINT('Ctrl Pts',(40.2553185305929,-33.6239269992694,3.9696179806421));
#8604=CARTESIAN_POINT('Ctrl Pts',(37.4677629373775,-32.3505541484834,3.82962489641198));
#8605=CARTESIAN_POINT('Ctrl Pts',(36.9340830890508,-30.6587196313569,3.74256005192377));
#8606=CARTESIAN_POINT('Ctrl Pts',(36.9298122993513,-29.9978467535325,3.70842344717745));
#8607=CARTESIAN_POINT('Ctrl Pts',(36.9253704391146,-29.9972894808084,4.79157655282255));
#8608=CARTESIAN_POINT('Ctrl Pts',(36.9235106070623,-29.7949370579245,4.78108579039918));
#8609=CARTESIAN_POINT('Ctrl Pts',(37.0339432909371,-28.5736915553199,4.71766678823392));
#8610=CARTESIAN_POINT('Ctrl Pts',(38.6680932394838,-26.6200513714892,4.60131954632676));
#8611=CARTESIAN_POINT('Ctrl Pts',(42.1176355025165,-27.0481110745022,4.44253482710108));
#8612=CARTESIAN_POINT('Ctrl Pts',(43.6285174446119,-30.1785763259747,4.28375010787539));
#8613=CARTESIAN_POINT('Ctrl Pts',(41.8175516063153,-33.1455579010144,4.12496538864971));
#8614=CARTESIAN_POINT('Ctrl Pts',(38.3426472969195,-33.2328331796093,3.96618066942402));
#8615=CARTESIAN_POINT('Ctrl Pts',(36.9725523682035,-31.2225583232012,3.85505105748164));
#8616=CARTESIAN_POINT('Ctrl Pts',(36.9219540996787,-30.1032148635415,3.79684968528114));
#8617=CARTESIAN_POINT('Ctrl Pts',(36.9226406398379,-30.0017378639268,3.79157655282254));
#8618=CARTESIAN_POINT('Origin',(40.,-30.,12.2084234471775));
#8619=CARTESIAN_POINT('',(36.9314881140875,-29.9999333228699,5.79157655282255));
#8620=CARTESIAN_POINT('',(36.9217351846713,-30.0009171118566,5.70842344717746));
#8621=CARTESIAN_POINT('',(36.9265,-29.9999999999999,12.2084234471775));
#8622=CARTESIAN_POINT('Ctrl Pts',(36.9217351846712,-30.0009171118566,5.70842344717746));
#8623=CARTESIAN_POINT('Ctrl Pts',(36.9255413846488,-29.0333155411646,5.65810402241795));
#8624=CARTESIAN_POINT('Ctrl Pts',(37.939039610796,-27.0410774185704,5.55485635791655));
#8625=CARTESIAN_POINT('Ctrl Pts',(41.3319070681429,-26.6200505908322,5.39868045367324));
#8626=CARTESIAN_POINT('Ctrl Pts',(43.5621112090423,-29.2862786390484,5.23989573444757));
#8627=CARTESIAN_POINT('Ctrl Pts',(42.531261381243,-32.6059068031093,5.08111101522187));
#8628=CARTESIAN_POINT('Ctrl Pts',(39.1830835732889,-33.5398703363926,4.92232629599619));
#8629=CARTESIAN_POINT('Ctrl Pts',(37.1486705732688,-31.7351430906943,4.79809710664805));
#8630=CARTESIAN_POINT('Ctrl Pts',(36.9272367419853,-30.3578751130926,4.7267961570418));
#8631=CARTESIAN_POINT('Ctrl Pts',(36.929634317343,-30.0022376272731,4.70842344717745));
#8632=CARTESIAN_POINT('Ctrl Pts',(36.9314881140875,-29.9999333228699,5.79157655282255));
#8633=CARTESIAN_POINT('Ctrl Pts',(36.931389649046,-29.4909574440388,5.76532189551721));
#8634=CARTESIAN_POINT('Ctrl Pts',(37.2923230006704,-27.956039860865,5.68613899846999));
#8635=CARTESIAN_POINT('Ctrl Pts',(39.7160732619294,-26.3782029380897,5.55402786168086));
#8636=CARTESIAN_POINT('Ctrl Pts',(42.8891152491159,-27.7974920142308,5.39524314245518));
#8637=CARTESIAN_POINT('Ctrl Pts',(43.4172199515306,-31.2331407676563,5.2364584232295));
#8638=CARTESIAN_POINT('Ctrl Pts',(40.8169162380303,-33.5398695187991,5.07767370400381));
#8639=CARTESIAN_POINT('Ctrl Pts',(37.6899502241597,-32.6676123107638,4.92937974720149));
#8640=CARTESIAN_POINT('Ctrl Pts',(36.9328938751957,-30.8158502307263,4.83401403014107));
#8641=CARTESIAN_POINT('Ctrl Pts',(36.9253704391146,-29.9972894808084,4.79157655282255));
#8642=CARTESIAN_POINT('Origin',(40.,-30.,12.2084234471775));
#8643=CARTESIAN_POINT('',(36.9256152724736,-30.0027445697125,6.79157655282255));
#8644=CARTESIAN_POINT('',(36.9269277951216,-29.9971906092403,6.70842344717746));
#8645=CARTESIAN_POINT('',(36.9265,-29.9999999999999,12.2084234471775));
#8646=CARTESIAN_POINT('Ctrl Pts',(36.9269277951216,-29.9971906092403,6.70842344717746));
#8647=CARTESIAN_POINT('Ctrl Pts',(36.9246263051997,-29.7431173813678,6.69526836727788));
#8648=CARTESIAN_POINT('Ctrl Pts',(37.0696628823468,-28.4693960079781,6.6291850476364));
#8649=CARTESIAN_POINT('Ctrl Pts',(38.8394460005071,-26.5574502389721,6.51017348825302));
#8650=CARTESIAN_POINT('Ctrl Pts',(42.2631511672664,-27.1581377158282,6.35138876902735));
#8651=CARTESIAN_POINT('Ctrl Pts',(43.6149788258837,-30.3605031695509,6.19260404980166));
#8652=CARTESIAN_POINT('Ctrl Pts',(41.6573530858745,-33.2328339262885,6.03381933057598));
#8653=CARTESIAN_POINT('Ctrl Pts',(38.1824479738899,-33.1455586275345,5.87503461135029));
#8654=CARTESIAN_POINT('Ctrl Pts',(36.9453831653551,-31.1188232709446,5.76656931688412));
#8655=CARTESIAN_POINT('Ctrl Pts',(36.9215378519002,-30.0510825000077,5.71103226215984));
#8656=CARTESIAN_POINT('Ctrl Pts',(36.9217351846712,-30.0009171118566,5.70842344717746));
#8657=CARTESIAN_POINT('Ctrl Pts',(36.9256152724736,-30.0027445697125,6.79157655282255));
#8658=CARTESIAN_POINT('Ctrl Pts',(36.9330941136838,-29.192098277692,6.74955800063525));
#8659=CARTESIAN_POINT('Ctrl Pts',(37.6777713604131,-27.3481783295783,6.65461120870605));
#8660=CARTESIAN_POINT('Ctrl Pts',(40.7889382915105,-26.453790089119,6.50673617703496));
#8661=CARTESIAN_POINT('Ctrl Pts',(43.4073759516192,-28.7399137026036,6.34795145780928));
#8662=CARTESIAN_POINT('Ctrl Pts',(42.9064172126614,-32.1796255027351,6.18916673858359));
#8663=CARTESIAN_POINT('Ctrl Pts',(39.7446815283789,-33.6239261622643,6.03038201935791));
#8664=CARTESIAN_POINT('Ctrl Pts',(37.3008224964414,-32.0603350218663,5.89785195743756));
#8665=CARTESIAN_POINT('Ctrl Pts',(36.9315881502591,-30.5170305336365,5.81825013525911));
#8666=CARTESIAN_POINT('Ctrl Pts',(36.9314881140875,-29.9999333228699,5.79157655282255));
#8667=CARTESIAN_POINT('Origin',(40.,-30.,12.2084234471775));
#8668=CARTESIAN_POINT('',(36.9224681139214,-29.9983795008932,7.79157655282255));
#8669=CARTESIAN_POINT('',(36.9313096321944,-30.0007718341681,7.70842344717745));
#8670=CARTESIAN_POINT('',(36.9265,-29.9999999999999,12.2084234471775));
#8671=CARTESIAN_POINT('Ctrl Pts',(36.9313096321944,-30.0007718341681,7.70842344717745));
#8672=CARTESIAN_POINT('Ctrl Pts',(36.932569127163,-29.4402260707305,7.67950447239591));
#8673=CARTESIAN_POINT('Ctrl Pts',(37.3479271339629,-27.8520174430537,7.59765725787246));
#8674=CARTESIAN_POINT('Ctrl Pts',(39.8982457703173,-26.3685154170426,7.46288180360713));
#8675=CARTESIAN_POINT('Ctrl Pts',(42.9960393923464,-27.9453023414519,7.30409708438144));
#8676=CARTESIAN_POINT('Ctrl Pts',(43.3510084475949,-31.4031310912316,7.14531236515576));
#8677=CARTESIAN_POINT('Ctrl Pts',(40.6381846226088,-33.576416475081,6.98652764593008));
#8678=CARTESIAN_POINT('Ctrl Pts',(37.6142708159026,-32.5667566968382,6.84089800660397));
#8679=CARTESIAN_POINT('Ctrl Pts',(36.9338861357197,-30.7653573692269,6.74819660701977));
#8680=CARTESIAN_POINT('Ctrl Pts',(36.9269277951216,-29.9971906092403,6.70842344717746));
#8681=CARTESIAN_POINT('Ctrl Pts',(36.9224681139214,-29.9983795008932,7.79157655282255));
#8682=CARTESIAN_POINT('Ctrl Pts',(36.9218706788586,-29.9049781453709,7.78672234549517));
#8683=CARTESIAN_POINT('Ctrl Pts',(36.9680975171812,-28.7937670349628,7.7289398984259));
#8684=CARTESIAN_POINT('Ctrl Pts',(38.3171711686706,-26.7803550620374,7.61822921161474));
#8685=CARTESIAN_POINT('Ctrl Pts',(41.7926560478477,-26.8401878205589,7.45944449238907));
#8686=CARTESIAN_POINT('Ctrl Pts',(43.6269942364715,-29.7927768135681,7.30065977316338));
#8687=CARTESIAN_POINT('Ctrl Pts',(42.1408789623084,-32.935075019391,7.1418750539377));
#8688=CARTESIAN_POINT('Ctrl Pts',(38.6948244410116,-33.3903606257847,6.98309033471201));
#8689=CARTESIAN_POINT('Ctrl Pts',(37.0393592098282,-31.4426976711376,6.86632416767363));
#8690=CARTESIAN_POINT('Ctrl Pts',(36.9236734678033,-30.2132205928703,6.80248624037714));
#8691=CARTESIAN_POINT('Ctrl Pts',(36.9256152724736,-30.0027445697125,6.79157655282255));
#8692=CARTESIAN_POINT('Origin',(40.,-30.,12.2084234471775));
#8693=CARTESIAN_POINT('',(36.9305018352452,-29.9982750548043,8.79157655282255));
#8694=CARTESIAN_POINT('',(36.9240972445879,-30.002414807271,8.70842344717745));
#8695=CARTESIAN_POINT('',(36.9265,-29.9999999999999,12.2084234471775));
#8696=CARTESIAN_POINT('Ctrl Pts',(36.9240972445879,-30.002414807271,8.70842344717746));
#8697=CARTESIAN_POINT('Ctrl Pts',(36.9315170701463,-29.1414653963739,8.66374057751394));
#8698=CARTESIAN_POINT('Ctrl Pts',(37.7570268484348,-27.248221324497,8.56612946810854));
#8699=CARTESIAN_POINT('Ctrl Pts',(40.9659640431824,-26.4978673441227,8.41559011896122));
#8700=CARTESIAN_POINT('Ctrl Pts',(43.4663370299824,-28.9125517016798,8.25680539973555));
#8701=CARTESIAN_POINT('Ctrl Pts',(42.7933360304446,-32.322780879739,8.09802068050986));
#8702=CARTESIAN_POINT('Ctrl Pts',(39.5630818867002,-33.6065405967288,7.93923596128418));
#8703=CARTESIAN_POINT('Ctrl Pts',(37.2482862242861,-31.9560992143217,7.80937021684005));
#8704=CARTESIAN_POINT('Ctrl Pts',(36.9302639675868,-30.4661511174393,7.7324327121378));
#8705=CARTESIAN_POINT('Ctrl Pts',(36.9313096321944,-30.0007718341681,7.70842344717745));
#8706=CARTESIAN_POINT('Ctrl Pts',(36.9305018352452,-29.9982750548043,8.79157655282255));
#8707=CARTESIAN_POINT('Ctrl Pts',(36.9284516052967,-29.598887638351,8.77095845061321));
#8708=CARTESIAN_POINT('Ctrl Pts',(37.186508597033,-28.1767817125267,8.69741210866198));
#8709=CARTESIAN_POINT('Ctrl Pts',(39.3336052322159,-26.4287487288557,8.57093752696886));
#8710=CARTESIAN_POINT('Ctrl Pts',(42.6392496071423,-27.5035235206868,8.41215280774315));
#8711=CARTESIAN_POINT('Ctrl Pts',(43.5287240702543,-30.8638054618116,8.25336808851749));
#8712=CARTESIAN_POINT('Ctrl Pts',(41.1877001687398,-33.4332756644217,8.09458336929179));
#8713=CARTESIAN_POINT('Ctrl Pts',(37.8641690175257,-32.8771812444488,7.94065285739349));
#8714=CARTESIAN_POINT('Ctrl Pts',(36.9283848600841,-30.9233873322688,7.83965058523707));
#8715=CARTESIAN_POINT('Ctrl Pts',(36.9224681139214,-29.9983795008932,7.79157655282255));
#8716=CARTESIAN_POINT('Origin',(40.,-30.,12.2084234471775));
#8717=CARTESIAN_POINT('',(36.9295986129496,-30.0034658759783,9.79157655282255));
#8718=CARTESIAN_POINT('',(36.9237142109313,-29.9977821171135,9.70842344717746));
#8719=CARTESIAN_POINT('',(36.9265,-29.9999999999999,12.2084234471775));
#8720=CARTESIAN_POINT('',(39.2062007174671,-32.9692229537457,10.));
#8721=CARTESIAN_POINT('Ctrl Pts',(39.2062007174671,-32.9692229537457,10.));
#8722=CARTESIAN_POINT('Ctrl Pts',(38.2187620536724,-32.7052387009375,9.94707176025811));
#8723=CARTESIAN_POINT('Ctrl Pts',(37.1203692887103,-31.663801299125,9.87759727786562));
#8724=CARTESIAN_POINT('Ctrl Pts',(36.9271779329065,-30.3235495409403,9.80812279547314));
#8725=CARTESIAN_POINT('Ctrl Pts',(36.9295986129496,-30.0034658759783,9.79157655282254));
#8726=CARTESIAN_POINT('',(40.7955465233069,-32.9745272340617,10.));
#8727=CARTESIAN_POINT('Origin',(40.,-30.,10.));
#8728=CARTESIAN_POINT('Ctrl Pts',(40.795547939453,-32.9745315332036,10.));
#8729=CARTESIAN_POINT('Ctrl Pts',(39.8333610342226,-33.2303404802746,9.94821753066413));
#8730=CARTESIAN_POINT('Ctrl Pts',(37.7694379004992,-32.755695571864,9.85102534638994));
#8731=CARTESIAN_POINT('Ctrl Pts',(36.9309457034163,-30.8722543866673,9.75383316211577));
#8732=CARTESIAN_POINT('Ctrl Pts',(36.9237142109313,-29.9977821171135,9.70842344717746));
#8733=CARTESIAN_POINT('Origin',(-40.,-30.,12.2084234471775));
#8734=CARTESIAN_POINT('',(-43.0785899477782,-29.9998519260269,0.791576552822544));
#8735=CARTESIAN_POINT('',(-43.0685561331992,-29.9992605379075,0.708423447177453));
#8736=CARTESIAN_POINT('',(-43.0735,-29.9999999999999,12.2084234471775));
#8737=CARTESIAN_POINT('',(-39.2062007174671,-32.9692229537457,0.));
#8738=CARTESIAN_POINT('Ctrl Pts',(-43.0685561331992,-29.9992605379075,0.708423447177453));
#8739=CARTESIAN_POINT('Ctrl Pts',(-43.0694087586157,-29.525699780414,0.683995257085881));
#8740=CARTESIAN_POINT('Ctrl Pts',(-42.7435312639193,-28.0273012908912,0.606638827252414));
#8741=CARTESIAN_POINT('Ctrl Pts',(-40.4091143639642,-26.3909743325875,0.47635415767705));
#8742=CARTESIAN_POINT('Ctrl Pts',(-37.1870296834247,-27.6976298827388,0.317569438451369));
#8743=CARTESIAN_POINT('Ctrl Pts',(-36.5451704756118,-31.1184197653857,0.158784719225683));
#8744=CARTESIAN_POINT('Ctrl Pts',(-38.2187620536724,-32.7052387009375,0.0529282397418946));
#8745=CARTESIAN_POINT('Ctrl Pts',(-39.2062007174671,-32.9692229537457,0.));
#8746=CARTESIAN_POINT('',(-40.7937992825329,-32.9692229537457,0.));
#8747=CARTESIAN_POINT('Origin',(-40.,-30.,0.));
#8748=CARTESIAN_POINT('Ctrl Pts',(-43.0785899477782,-29.9998519260269,0.791576552822544));
#8749=CARTESIAN_POINT('Ctrl Pts',(-43.0785942836995,-29.9928657045085,0.791213130185147));
#8750=CARTESIAN_POINT('Ctrl Pts',(-43.0754098879479,-28.9684227656317,0.737921467805856));
#8751=CARTESIAN_POINT('Ctrl Pts',(-41.9490298715236,-26.9342997681684,0.631701565684669));
#8752=CARTESIAN_POINT('Ctrl Pts',(-38.4808975311013,-26.6996618476225,0.472916846458986));
#8753=CARTESIAN_POINT('Ctrl Pts',(-36.4035550403569,-29.4874091667537,0.314132127233303));
#8754=CARTESIAN_POINT('Ctrl Pts',(-37.6097787213515,-32.7189778808771,0.156493178413639));
#8755=CARTESIAN_POINT('Ctrl Pts',(-39.8333607858277,-33.2303406028725,0.051782469335873));
#8756=CARTESIAN_POINT('Ctrl Pts',(-40.7955478019228,-32.974531551058,4.67562186884374E-17));
#8757=CARTESIAN_POINT('Origin',(-40.,-30.,12.2084234471775));
#8758=CARTESIAN_POINT('',(-43.071434903389,-29.9974006852265,1.79157655282254));
#8759=CARTESIAN_POINT('',(-43.0733149456894,-30.0028121937047,1.70842344717745));
#8760=CARTESIAN_POINT('',(-43.0735,-29.9999999999999,12.2084234471775));
#8761=CARTESIAN_POINT('Ctrl Pts',(-43.0733149456894,-30.0028121937047,1.70842344717745));
#8762=CARTESIAN_POINT('Ctrl Pts',(-43.0662259767823,-29.2267098723251,1.66823136220391));
#8763=CARTESIAN_POINT('Ctrl Pts',(-42.3741036197155,-27.4173151902012,1.57511103748848));
#8764=CARTESIAN_POINT('Ctrl Pts',(-39.333605094551,-26.4287480480142,1.42906247303115));
#8765=CARTESIAN_POINT('Ctrl Pts',(-36.6379947680772,-28.6233470921482,1.27027775380547));
#8766=CARTESIAN_POINT('Ctrl Pts',(-37.0203223217504,-32.078345102403,1.11149303457979));
#8767=CARTESIAN_POINT('Ctrl Pts',(-40.1303405334711,-33.6304608367794,0.952708315354102));
#8768=CARTESIAN_POINT('Ctrl Pts',(-42.661193724397,-32.1318111884618,0.81835178621999));
#8769=CARTESIAN_POINT('Ctrl Pts',(-43.0675613862855,-30.5517576754528,0.736923496827775));
#8770=CARTESIAN_POINT('Ctrl Pts',(-43.0685561331992,-29.9992605379075,0.708423447177453));
#8771=CARTESIAN_POINT('Ctrl Pts',(-43.071434903389,-29.9974006852265,1.79157655282254));
#8772=CARTESIAN_POINT('Ctrl Pts',(-43.0739380024191,-29.6855008432268,1.77544923530318));
#8773=CARTESIAN_POINT('Ctrl Pts',(-42.8868351144726,-28.3529096785031,1.70639367804192));
#8774=CARTESIAN_POINT('Ctrl Pts',(-40.9659640066834,-26.4978674771854,1.58440988103877));
#8775=CARTESIAN_POINT('Ctrl Pts',(-37.5812664167199,-27.2893199539358,1.42562516181309));
#8776=CARTESIAN_POINT('Ctrl Pts',(-36.410880674872,-30.5623706761659,1.26684044258741));
#8777=CARTESIAN_POINT('Ctrl Pts',(-38.5262719729362,-33.320549494049,1.10805572336172));
#8778=CARTESIAN_POINT('Ctrl Pts',(-41.9829121303265,-33.0395263722366,0.949634426773433));
#8779=CARTESIAN_POINT('Ctrl Pts',(-43.0779628076698,-31.0103268347954,0.844141369927042));
#8780=CARTESIAN_POINT('Ctrl Pts',(-43.0785899477782,-29.9998519260269,0.791576552822544));
#8781=CARTESIAN_POINT('Origin',(-40.,-30.,12.2084234471775));
#8782=CARTESIAN_POINT('',(-43.0693702153585,-30.0016239406685,2.79157655282254));
#8783=CARTESIAN_POINT('',(-43.078155414487,-29.9989435322699,2.70842344717745));
#8784=CARTESIAN_POINT('',(-43.0735,-29.9999999999999,12.2084234471775));
#8785=CARTESIAN_POINT('Ctrl Pts',(-43.078155414487,-29.9989435322699,2.70842344717745));
#8786=CARTESIAN_POINT('Ctrl Pts',(-43.0784148906334,-29.9407170508587,2.70539570706384));
#8787=CARTESIAN_POINT('Ctrl Pts',(-43.0505262473693,-28.8648808671286,2.64943972720834));
#8788=CARTESIAN_POINT('Ctrl Pts',(-41.7926563602578,-26.8401872712874,2.54055550761094));
#8789=CARTESIAN_POINT('Ctrl Pts',(-38.3171708750578,-26.7803545002487,2.38177078838525));
#8790=CARTESIAN_POINT('Ctrl Pts',(-36.3822870422175,-29.6680532410143,2.22298606915957));
#8791=CARTESIAN_POINT('Ctrl Pts',(-37.7593608839214,-32.8596452685709,2.06420134993389));
#8792=CARTESIAN_POINT('Ctrl Pts',(-41.1877003796151,-33.4332762712177,1.9054166307082));
#8793=CARTESIAN_POINT('Ctrl Pts',(-42.9361572817983,-31.5141980525073,1.78682399645606));
#8794=CARTESIAN_POINT('Ctrl Pts',(-43.0755613134807,-30.248745174979,1.72115960194581));
#8795=CARTESIAN_POINT('Ctrl Pts',(-43.0733149456894,-30.0028121937047,1.70842344717745));
#8796=CARTESIAN_POINT('Ctrl Pts',(-43.0693702153585,-30.0016239406685,2.79157655282254));
#8797=CARTESIAN_POINT('Ctrl Pts',(-43.0664100283933,-29.3838086413388,2.75968534042121));
#8798=CARTESIAN_POINT('Ctrl Pts',(-42.5856196442103,-27.7363975024695,2.67486588827799));
#8799=CARTESIAN_POINT('Ctrl Pts',(-39.898245774117,-26.3685155528715,2.53711819639287));
#8800=CARTESIAN_POINT('Ctrl Pts',(-36.8936065712748,-28.1162925878559,2.37833347716719));
#8801=CARTESIAN_POINT('Ctrl Pts',(-36.7328192563745,-31.5885728846373,2.2195487579415));
#8802=CARTESIAN_POINT('Ctrl Pts',(-39.5630819030797,-33.6065404615547,2.06076403871582));
#8803=CARTESIAN_POINT('Ctrl Pts',(-42.4652481064523,-32.4531686537838,1.9181066370095));
#8804=CARTESIAN_POINT('Ctrl Pts',(-43.0657230822749,-30.7091248645808,1.82837747504507));
#8805=CARTESIAN_POINT('Ctrl Pts',(-43.071434903389,-29.9974006852265,1.79157655282254));
#8806=CARTESIAN_POINT('Origin',(-40.,-30.,12.2084234471775));
#8807=CARTESIAN_POINT('',(-43.0773599558693,-30.0017378642629,3.79157655282254));
#8808=CARTESIAN_POINT('',(-43.0701875259343,-29.9978467536557,3.70842344717745));
#8809=CARTESIAN_POINT('',(-43.0735,-29.9999999999999,12.2084234471775));
#8810=CARTESIAN_POINT('Ctrl Pts',(-43.0701875259343,-29.9978467536557,3.70842344717745));
#8811=CARTESIAN_POINT('Ctrl Pts',(-43.0725385247289,-29.6340472110791,3.68963181218188));
#8812=CARTESIAN_POINT('Ctrl Pts',(-42.8444471428709,-28.2484271981974,3.61791193744441));
#8813=CARTESIAN_POINT('Ctrl Pts',(-40.7889384288422,-26.4537894718797,3.49326382296504));
#8814=CARTESIAN_POINT('Ctrl Pts',(-37.4482402188302,-27.414162624453,3.33447910373936));
#8815=CARTESIAN_POINT('Ctrl Pts',(-36.4436359258312,-30.7418271664764,3.17569438451367));
#8816=CARTESIAN_POINT('Ctrl Pts',(-38.6948242137735,-33.3903612158066,3.01690966528799));
#8817=CARTESIAN_POINT('Ctrl Pts',(-42.0751692379219,-32.9437570127916,2.86115268617591));
#8818=CARTESIAN_POINT('Ctrl Pts',(-43.0738789611389,-30.9585802266324,2.75832394680574));
#8819=CARTESIAN_POINT('Ctrl Pts',(-43.078155414487,-29.9989435322699,2.70842344717745));
#8820=CARTESIAN_POINT('Ctrl Pts',(-43.0773599558693,-30.0017378642629,3.79157655282254));
#8821=CARTESIAN_POINT('Ctrl Pts',(-43.0711554556919,-29.084655223629,3.74392144553925));
#8822=CARTESIAN_POINT('Ctrl Pts',(-42.1494521684416,-27.1381894005441,3.64333809851406));
#8823=CARTESIAN_POINT('Ctrl Pts',(-38.8394460438999,-26.5574503676893,3.48982651174697));
#8824=CARTESIAN_POINT('Ctrl Pts',(-36.4782089804049,-29.1083602316377,3.33104179252129));
#8825=CARTESIAN_POINT('Ctrl Pts',(-37.341113418528,-32.4755515781919,3.17225707329561));
#8826=CARTESIAN_POINT('Ctrl Pts',(-40.6381845987477,-33.5764163413526,3.01347235406993));
#8827=CARTESIAN_POINT('Ctrl Pts',(-42.8061496104729,-31.839625832053,2.88657884724557));
#8828=CARTESIAN_POINT('Ctrl Pts',(-43.0713229016765,-30.4091655913233,2.81261358016311));
#8829=CARTESIAN_POINT('Ctrl Pts',(-43.0693702153585,-30.0016239406685,2.79157655282254));
#8830=CARTESIAN_POINT('Origin',(-40.,-30.,12.2084234471775));
#8831=CARTESIAN_POINT('',(-43.0746301560641,-29.9972894802837,4.79157655282255));
#8832=CARTESIAN_POINT('',(-43.0703655079321,-30.0022376271458,4.70842344717746));
#8833=CARTESIAN_POINT('',(-43.0735,-29.9999999999999,12.2084234471775));
#8834=CARTESIAN_POINT('Ctrl Pts',(-43.0703655079321,-30.0022376271458,4.70842344717746));
#8835=CARTESIAN_POINT('Ctrl Pts',(-43.0658561305564,-29.3333520268071,4.67386791729991));
#8836=CARTESIAN_POINT('Ctrl Pts',(-42.5219683951878,-27.6332680766331,4.58638414768047));
#8837=CARTESIAN_POINT('Ctrl Pts',(-39.7160732125092,-26.378202307679,4.44597213831914));
#8838=CARTESIAN_POINT('Ctrl Pts',(-36.8029609568071,-28.274608942761,4.28718741909346));
#8839=CARTESIAN_POINT('Ctrl Pts',(-36.8166851325132,-31.7505825885012,4.12840269986777));
#8840=CARTESIAN_POINT('Ctrl Pts',(-39.7446814839369,-33.6239267930437,3.96961798064209));
#8841=CARTESIAN_POINT('Ctrl Pts',(-42.5322369185202,-32.3505540147196,3.82962489641198));
#8842=CARTESIAN_POINT('Ctrl Pts',(-43.0659167364777,-30.6587195938717,3.74256005192377));
#8843=CARTESIAN_POINT('Ctrl Pts',(-43.0701875259343,-29.9978467536557,3.70842344717745));
#8844=CARTESIAN_POINT('Ctrl Pts',(-43.0746301560641,-29.9972894802837,4.79157655282255));
#8845=CARTESIAN_POINT('Ctrl Pts',(-43.0764899884764,-29.794937018229,4.78108579039918));
#8846=CARTESIAN_POINT('Ctrl Pts',(-42.9660572832244,-28.5736912792188,4.71766678823392));
#8847=CARTESIAN_POINT('Ctrl Pts',(-41.3319070183432,-26.6200507172078,4.60131954632676));
#8848=CARTESIAN_POINT('Ctrl Pts',(-37.8823640875572,-27.0481105030832,4.44253482710108));
#8849=CARTESIAN_POINT('Ctrl Pts',(-36.3714818529893,-30.1785763605433,4.28375010787539));
#8850=CARTESIAN_POINT('Ctrl Pts',(-38.1824480418478,-33.1455585099229,4.12496538864971));
#8851=CARTESIAN_POINT('Ctrl Pts',(-41.6573530239065,-33.2328338054134,3.96618066942403));
#8852=CARTESIAN_POINT('Ctrl Pts',(-43.0274482178419,-31.2225585598601,3.85505105748164));
#8853=CARTESIAN_POINT('Ctrl Pts',(-43.0780464961614,-30.1032148835213,3.79684968528114));
#8854=CARTESIAN_POINT('Ctrl Pts',(-43.0773599558693,-30.0017378642629,3.79157655282254));
#8855=CARTESIAN_POINT('Origin',(-40.,-30.,12.2084234471775));
#8856=CARTESIAN_POINT('',(-43.0685124799068,-29.9999333228573,5.79157655282255));
#8857=CARTESIAN_POINT('',(-43.0782646401543,-30.0009171118044,5.70842344717746));
#8858=CARTESIAN_POINT('',(-43.0735,-29.9999999999999,12.2084234471775));
#8859=CARTESIAN_POINT('Ctrl Pts',(-43.0782646401543,-30.0009171118044,5.70842344717746));
#8860=CARTESIAN_POINT('Ctrl Pts',(-43.0744584403933,-29.0333155961755,5.65810402241795));
#8861=CARTESIAN_POINT('Ctrl Pts',(-42.0609602719212,-27.0410775869535,5.55485635791654));
#8862=CARTESIAN_POINT('Ctrl Pts',(-38.6680930076518,-26.6200507831746,5.39868045367324));
#8863=CARTESIAN_POINT('Ctrl Pts',(-36.4378889936663,-29.286278679664,5.23989573444756));
#8864=CARTESIAN_POINT('Ctrl Pts',(-37.4687387628032,-32.6059066548152,5.08111101522187));
#8865=CARTESIAN_POINT('Ctrl Pts',(-40.8169163802229,-33.5398701349496,4.92232629599619));
#8866=CARTESIAN_POINT('Ctrl Pts',(-42.8513292644709,-31.7351429919527,4.79809710664805));
#8867=CARTESIAN_POINT('Ctrl Pts',(-43.0727630831533,-30.357875092727,4.72679615704181));
#8868=CARTESIAN_POINT('Ctrl Pts',(-43.0703655079321,-30.0022376271458,4.70842344717746));
#8869=CARTESIAN_POINT('Ctrl Pts',(-43.0685124799068,-29.9999333228573,5.79157655282255));
#8870=CARTESIAN_POINT('Ctrl Pts',(-43.0686109449675,-29.4909573454998,5.76532189551721));
#8871=CARTESIAN_POINT('Ctrl Pts',(-42.7076775234749,-27.9560394652001,5.68613899846998));
#8872=CARTESIAN_POINT('Ctrl Pts',(-40.2839267930322,-26.378202236992,5.55402786168086));
#8873=CARTESIAN_POINT('Ctrl Pts',(-37.1108841916168,-27.7974915878749,5.39524314245518));
#8874=CARTESIAN_POINT('Ctrl Pts',(-36.5827793869729,-31.2331410063646,5.23645842322949));
#8875=CARTESIAN_POINT('Ctrl Pts',(-39.1830836038332,-33.5398702040376,5.07767370400381));
#8876=CARTESIAN_POINT('Ctrl Pts',(-42.3100502230137,-32.6676128271532,4.9293797472015));
#8877=CARTESIAN_POINT('Ctrl Pts',(-43.0671067185266,-30.8158503886565,4.83401403014107));
#8878=CARTESIAN_POINT('Ctrl Pts',(-43.0746301560641,-29.9972894802837,4.79157655282255));
#8879=CARTESIAN_POINT('Origin',(-40.,-30.,12.2084234471775));
#8880=CARTESIAN_POINT('',(-43.0743853226466,-30.0027445702633,6.79157655282254));
#8881=CARTESIAN_POINT('',(-43.0730720299995,-29.9971906094003,6.70842344717746));
#8882=CARTESIAN_POINT('',(-43.0735,-29.9999999999999,12.2084234471775));
#8883=CARTESIAN_POINT('Ctrl Pts',(-43.0730720299995,-29.9971906094003,6.70842344717746));
#8884=CARTESIAN_POINT('Ctrl Pts',(-43.0753735197904,-29.7431173959859,6.69526836727788));
#8885=CARTESIAN_POINT('Ctrl Pts',(-42.9303369508968,-28.4693960950782,6.6291850476364));
#8886=CARTESIAN_POINT('Ctrl Pts',(-41.1605539334494,-26.5574504348784,6.51017348825302));
#8887=CARTESIAN_POINT('Ctrl Pts',(-37.7368489615224,-27.1581378775489,6.35138876902735));
#8888=CARTESIAN_POINT('Ctrl Pts',(-36.3850213798334,-30.3605031490362,6.19260404980165));
#8889=CARTESIAN_POINT('Ctrl Pts',(-38.3426470084403,-33.2328337423178,6.03381933057598));
#8890=CARTESIAN_POINT('Ctrl Pts',(-41.8175519226788,-33.1455584485307,5.87503461135029));
#8891=CARTESIAN_POINT('Ctrl Pts',(-43.0546166608162,-31.1188232072758,5.76656931688412));
#8892=CARTESIAN_POINT('Ctrl Pts',(-43.0784619729141,-30.0510824971007,5.71103226215984));
#8893=CARTESIAN_POINT('Ctrl Pts',(-43.0782646401543,-30.0009171118044,5.70842344717746));
#8894=CARTESIAN_POINT('Ctrl Pts',(-43.0743853226466,-30.0027445702633,6.79157655282254));
#8895=CARTESIAN_POINT('Ctrl Pts',(-43.0669064799895,-29.1920981213188,6.74955800063525));
#8896=CARTESIAN_POINT('Ctrl Pts',(-42.3222290891344,-27.3481778162171,6.65461120870605));
#8897=CARTESIAN_POINT('Ctrl Pts',(-39.2110615557591,-26.4537894026696,6.50673617703496));
#8898=CARTESIAN_POINT('Ctrl Pts',(-36.592623388795,-28.7399134586708,6.34795145780928));
#8899=CARTESIAN_POINT('Ctrl Pts',(-37.0935822247194,-32.1796259246658,6.18916673858359));
#8900=CARTESIAN_POINT('Ctrl Pts',(-40.2553185210464,-33.623926863772,6.03038201935791));
#8901=CARTESIAN_POINT('Ctrl Pts',(-42.6991780260579,-32.0603354207011,5.89785195743756));
#8902=CARTESIAN_POINT('Ctrl Pts',(-43.0684124437158,-30.5170306337223,5.81825013525911));
#8903=CARTESIAN_POINT('Ctrl Pts',(-43.0685124799068,-29.9999333228573,5.79157655282255));
#8904=CARTESIAN_POINT('Origin',(-40.,-30.,12.2084234471775));
#8905=CARTESIAN_POINT('',(-43.0775324815367,-29.9983795011158,7.79157655282255));
#8906=CARTESIAN_POINT('',(-43.0686901931836,-30.000771834183,7.70842344717745));
#8907=CARTESIAN_POINT('',(-43.0735,-29.9999999999999,12.2084234471775));
#8908=CARTESIAN_POINT('Ctrl Pts',(-43.0686901931836,-30.000771834183,7.70842344717745));
#8909=CARTESIAN_POINT('Ctrl Pts',(-43.0674306982834,-29.4402261026139,7.67950447239591));
#8910=CARTESIAN_POINT('Ctrl Pts',(-42.652072715104,-27.8520175651811,7.59765725787246));
#8911=CARTESIAN_POINT('Ctrl Pts',(-40.1017542238995,-26.368515623773,7.46288180360714));
#8912=CARTESIAN_POINT('Ctrl Pts',(-37.0039607781453,-27.9453024583394,7.30409708438144));
#8913=CARTESIAN_POINT('Ctrl Pts',(-36.6489917431023,-31.4031310114043,7.14531236515577));
#8914=CARTESIAN_POINT('Ctrl Pts',(-39.3618154137075,-33.5764162715476,6.98652764593008));
#8915=CARTESIAN_POINT('Ctrl Pts',(-42.3857290483333,-32.5667565507764,6.84089800660397));
#8916=CARTESIAN_POINT('Ctrl Pts',(-43.0661136897974,-30.7653573256739,6.74819660701977));
#8917=CARTESIAN_POINT('Ctrl Pts',(-43.0730720299995,-29.9971906094003,6.70842344717746));
#8918=CARTESIAN_POINT('Ctrl Pts',(-43.0775324815367,-29.9983795011158,7.79157655282255));
#8919=CARTESIAN_POINT('Ctrl Pts',(-43.0781299166727,-29.904978127604,7.78672234549517));
#8920=CARTESIAN_POINT('Ctrl Pts',(-43.0319030689719,-28.7937668030163,7.72893989842591));
#8921=CARTESIAN_POINT('Ctrl Pts',(-41.6828291578641,-26.7803544372571,7.61822921161475));
#8922=CARTESIAN_POINT('Ctrl Pts',(-38.2073436047123,-26.8401872096979,7.45944449238906));
#8923=CARTESIAN_POINT('Ctrl Pts',(-36.3730050616526,-29.7927767730296,7.30065977316338));
#8924=CARTESIAN_POINT('Ctrl Pts',(-37.8591206231434,-32.9350755877781,7.1418750539377));
#8925=CARTESIAN_POINT('Ctrl Pts',(-41.3051758117063,-33.390361281965,6.98309033471201));
#8926=CARTESIAN_POINT('Ctrl Pts',(-42.9606413632765,-31.4426979504252,6.86632416767362));
#8927=CARTESIAN_POINT('Ctrl Pts',(-43.0763271276925,-30.2132206341649,6.80248624037714));
#8928=CARTESIAN_POINT('Ctrl Pts',(-43.0743853226466,-30.0027445702633,6.79157655282254));
#8929=CARTESIAN_POINT('Origin',(-40.,-30.,12.2084234471775));
#8930=CARTESIAN_POINT('',(-43.069498762849,-29.9982750316902,8.79157655282255));
#8931=CARTESIAN_POINT('',(-43.0759025811495,-30.0024148106623,8.70842344717746));
#8932=CARTESIAN_POINT('',(-43.0735,-29.9999999999999,12.2084234471775));
#8933=CARTESIAN_POINT('Ctrl Pts',(-43.0759025811495,-30.0024148106623,8.70842344717746));
#8934=CARTESIAN_POINT('Ctrl Pts',(-43.0684827561252,-29.1414654488785,8.66374057751394));
#8935=CARTESIAN_POINT('Ctrl Pts',(-42.242973022817,-27.2482214756128,8.56612946810854));
#8936=CARTESIAN_POINT('Ctrl Pts',(-39.0340360123693,-26.4978675466446,8.41559011896124));
#8937=CARTESIAN_POINT('Ctrl Pts',(-36.5336631669943,-28.9125517618253,8.25680539973554));
#8938=CARTESIAN_POINT('Ctrl Pts',(-37.2066641286517,-32.3227807484881,8.09802068050986));
#8939=CARTESIAN_POINT('Ctrl Pts',(-40.4369180883703,-33.6065403909949,7.93923596128418));
#8940=CARTESIAN_POINT('Ctrl Pts',(-42.7517136191364,-31.9560991031317,7.80937021684005));
#8941=CARTESIAN_POINT('Ctrl Pts',(-43.0697358577345,-30.4661510909961,7.7324327121378));
#8942=CARTESIAN_POINT('Ctrl Pts',(-43.0686901931836,-30.000771834183,7.70842344717745));
#8943=CARTESIAN_POINT('Ctrl Pts',(-43.069498762849,-29.9982750316902,8.79157655282255));
#8944=CARTESIAN_POINT('Ctrl Pts',(-43.0715489864528,-29.5988875600661,8.77095845061321));
#8945=CARTESIAN_POINT('Ctrl Pts',(-42.8134919208485,-28.1767814426558,8.69741210866198));
#8946=CARTESIAN_POINT('Ctrl Pts',(-40.6663949208769,-26.4287479717036,8.57093752696886));
#8947=CARTESIAN_POINT('Ctrl Pts',(-37.3607498677919,-27.5035230729969,8.41215280774315));
#8948=CARTESIAN_POINT('Ctrl Pts',(-36.4712752548112,-30.8638056099088,8.25336808851749));
#8949=CARTESIAN_POINT('Ctrl Pts',(-38.8122995967417,-33.4332763392514,8.0945833692918));
#8950=CARTESIAN_POINT('Ctrl Pts',(-42.1358313982743,-32.8771817964379,7.94065285739349));
#8951=CARTESIAN_POINT('Ctrl Pts',(-43.07161573465,-30.9233875106515,7.83965058523707));
#8952=CARTESIAN_POINT('Ctrl Pts',(-43.0775324815367,-29.9983795011158,7.79157655282255));
#8953=CARTESIAN_POINT('Origin',(-40.,-30.,12.2084234471775));
#8954=CARTESIAN_POINT('',(-43.0704010605908,-30.0034624020472,9.79157655282255));
#8955=CARTESIAN_POINT('',(-43.0762856310176,-29.997782176874,9.70842344717746));
#8956=CARTESIAN_POINT('',(-43.0735,-29.9999999999999,12.2084234471775));
#8957=CARTESIAN_POINT('',(-40.7937992825329,-32.9692229537457,10.));
#8958=CARTESIAN_POINT('Ctrl Pts',(-40.7937992825329,-32.9692229537457,10.));
#8959=CARTESIAN_POINT('Ctrl Pts',(-41.7812379463276,-32.7052387009375,9.94707176025811));
#8960=CARTESIAN_POINT('Ctrl Pts',(-42.879629843998,-31.663795760744,9.87759727786561));
#8961=CARTESIAN_POINT('Ctrl Pts',(-43.072821611806,-30.3235455230037,9.80812279547314));
#8962=CARTESIAN_POINT('Ctrl Pts',(-43.0704010605908,-30.0034624020472,9.79157655282255));
#8963=CARTESIAN_POINT('',(-39.204453684107,-32.9745272669182,10.));
#8964=CARTESIAN_POINT('Origin',(-40.,-30.,10.));
#8965=CARTESIAN_POINT('Ctrl Pts',(-39.2044522699742,-32.9745315604842,10.));
#8966=CARTESIAN_POINT('Ctrl Pts',(-40.166639343954,-33.2303406669821,9.94821753066412));
#8967=CARTESIAN_POINT('Ctrl Pts',(-42.2305616481375,-32.7556949590643,9.85102534638995));
#8968=CARTESIAN_POINT('Ctrl Pts',(-43.0690540701593,-30.8722543038914,9.75383316211577));
#8969=CARTESIAN_POINT('Ctrl Pts',(-43.0762856310176,-29.997782176874,9.70842344717746));
#8970=CARTESIAN_POINT('Origin',(-40.,-30.,12.2084234471775));
#8971=CARTESIAN_POINT('Ctrl Pts',(-43.0762856310176,-29.997782176874,9.70842344717746));
#8972=CARTESIAN_POINT('Ctrl Pts',(-43.0774829666484,-29.852995089222,9.70090492237387));
#8973=CARTESIAN_POINT('Ctrl Pts',(-43.0023605019912,-28.6901611816683,9.64045815782839));
#8974=CARTESIAN_POINT('Ctrl Pts',(-41.5191024081009,-26.6996618460447,9.52708315354101));
#8975=CARTESIAN_POINT('Ctrl Pts',(-38.0509701816934,-26.934299866359,9.36829843431533));
#8976=CARTESIAN_POINT('Ctrl Pts',(-36.3671808918873,-29.9750448667934,9.20951371508965));
#8977=CARTESIAN_POINT('Ctrl Pts',(-38.0091582883336,-33.0388816507496,9.05072899586396));
#8978=CARTESIAN_POINT('Ctrl Pts',(-41.4737279965523,-33.3205494224222,8.89194427663828));
#8979=CARTESIAN_POINT('Ctrl Pts',(-42.9938368358631,-31.3385369294681,8.77784242707611));
#8980=CARTESIAN_POINT('Ctrl Pts',(-43.0772717681266,-30.1612865697975,8.71666881725583));
#8981=CARTESIAN_POINT('Ctrl Pts',(-43.0759025811495,-30.0024148106623,8.70842344717746));
#8982=CARTESIAN_POINT('Ctrl Pts',(-43.0704010605908,-30.0034624020472,9.79157655282255));
#8983=CARTESIAN_POINT('Ctrl Pts',(-43.0650787352067,-29.2996613384747,9.75519455573124));
#8984=CARTESIAN_POINT('Ctrl Pts',(-42.4772114414296,-27.5614694578342,9.66588431889805));
#8985=CARTESIAN_POINT('Ctrl Pts',(-39.5908856218057,-26.3909740388041,9.52364584232295));
#8986=CARTESIAN_POINT('Ctrl Pts',(-36.745809981275,-28.3852514028181,9.36486112309727));
#8987=CARTESIAN_POINT('Ctrl Pts',(-36.8786561820279,-31.8593324073604,9.20607640387158));
#8988=CARTESIAN_POINT('Ctrl Pts',(-39.869659454766,-33.6304609478428,9.0472916846459));
#8989=CARTESIAN_POINT('Ctrl Pts',(-42.5758437009482,-32.2798864461415,8.90912506762956));
#8990=CARTESIAN_POINT('Ctrl Pts',(-43.0662859062079,-30.6241456383026,8.8238866903551));
#8991=CARTESIAN_POINT('Ctrl Pts',(-43.069498762849,-29.9982750316902,8.79157655282255));
#8992=CARTESIAN_POINT('Ctrl Pts',(-38.0865340033349,-28.364012796625,10.));
#8993=CARTESIAN_POINT('Ctrl Pts',(-37.5424734719262,-29.0003511034471,9.94707176025811));
#8994=CARTESIAN_POINT('Ctrl Pts',(-37.1490030310892,-30.8479858487614,9.84121528077432));
#8995=CARTESIAN_POINT('Ctrl Pts',(-39.1694205041011,-32.8592860233099,9.68243056154863));
#8996=CARTESIAN_POINT('Ctrl Pts',(-41.9506458901437,-32.2463502392111,9.52364584232295));
#8997=CARTESIAN_POINT('Ctrl Pts',(-42.9458435562516,-29.5801375894759,9.36486112309726));
#8998=CARTESIAN_POINT('Ctrl Pts',(-41.2442948795815,-27.2966971522426,9.20607640387158));
#8999=CARTESIAN_POINT('Ctrl Pts',(-38.4035521172648,-27.4888888607642,9.0472916846459));
#9000=CARTESIAN_POINT('Ctrl Pts',(-37.0243624191724,-29.9795592816503,8.88850696542021));
#9001=CARTESIAN_POINT('Ctrl Pts',(-38.3693040477892,-32.4891441534934,8.72972224619453));
#9002=CARTESIAN_POINT('Ctrl Pts',(-41.2071287559201,-32.7198578724412,8.57093752696884));
#9003=CARTESIAN_POINT('Ctrl Pts',(-42.9398430866436,-30.460637110478,8.41215280774317));
#9004=CARTESIAN_POINT('Ctrl Pts',(-41.9811816092491,-27.779685411444,8.25336808851748));
#9005=CARTESIAN_POINT('Ctrl Pts',(-39.2087801077402,-27.1314076943803,8.0945833692918));
#9006=CARTESIAN_POINT('Ctrl Pts',(-37.1607278421696,-29.1092725102961,7.93579865006611));
#9007=CARTESIAN_POINT('Ctrl Pts',(-37.7119820868328,-31.9025868014703,7.77701393084044));
#9008=CARTESIAN_POINT('Ctrl Pts',(-40.3578790588815,-32.9541127165542,7.61822921161474));
#9009=CARTESIAN_POINT('Ctrl Pts',(-42.6761436022691,-31.3011980345695,7.45944449238907));
#9010=CARTESIAN_POINT('Ctrl Pts',(-42.5444429166006,-28.4570576484011,7.30065977316337));
#9011=CARTESIAN_POINT('Ctrl Pts',(-40.0833467573344,-27.025455696388,7.1418750539377));
#9012=CARTESIAN_POINT('Ctrl Pts',(-37.5459480263481,-28.3169998174294,6.98309033471201));
#9013=CARTESIAN_POINT('Ctrl Pts',(-37.255193334394,-31.1493028538182,6.82430561548633));
#9014=CARTESIAN_POINT('Ctrl Pts',(-39.4772638047856,-32.9294380880498,6.66552089626065));
#9015=CARTESIAN_POINT('Ctrl Pts',(-42.1778906257405,-32.0277211571395,6.50673617703496));
#9016=CARTESIAN_POINT('Ctrl Pts',(-42.8846945563006,-29.2696589968946,6.34795145780928));
#9017=CARTESIAN_POINT('Ctrl Pts',(-40.950608273128,-27.1802119634965,6.18916673858359));
#9018=CARTESIAN_POINT('Ctrl Pts',(-38.1462558193046,-27.6722342953406,6.03038201935791));
#9019=CARTESIAN_POINT('Ctrl Pts',(-37.0389755405013,-30.2952876777936,5.87159730013223));
#9020=CARTESIAN_POINT('Ctrl Pts',(-38.642464240686,-32.6480100687441,5.71281258090654));
#9021=CARTESIAN_POINT('Ctrl Pts',(-41.4887545031215,-32.5765229849279,5.55402786168087));
#9022=CARTESIAN_POINT('Ctrl Pts',(-42.9721146109695,-30.1462716703736,5.39524314245517));
#9023=CARTESIAN_POINT('Ctrl Pts',(-41.7345528893855,-27.5821110579311,5.2364584232295));
#9024=CARTESIAN_POINT('Ctrl Pts',(-38.9090366509723,-27.2314878303699,5.07767370400381));
#9025=CARTESIAN_POINT('Ctrl Pts',(-37.0822793367675,-29.4153917605512,4.91888898477813));
#9026=CARTESIAN_POINT('Ctrl Pts',(-37.9266470913801,-32.134494876687,4.76010426555244));
#9027=CARTESIAN_POINT('Ctrl Pts',(-40.6691351837356,-32.8995031933417,4.60131954632676));
#9028=CARTESIAN_POINT('Ctrl Pts',(-42.7990410689418,-31.0100642339135,4.44253482710107));
#9029=CARTESIAN_POINT('Ctrl Pts',(-42.3664710934277,-28.1959281537966,4.28375010787539));
#9030=CARTESIAN_POINT('Ctrl Pts',(-39.7674359240253,-27.0333900470415,4.12496538864971));
#9031=CARTESIAN_POINT('Ctrl Pts',(-37.3813093244711,-28.5867343463155,3.96618066942403));
#9032=CARTESIAN_POINT('Ctrl Pts',(-37.3925507796004,-31.4339000053853,3.80739595019834));
#9033=CARTESIAN_POINT('Ctrl Pts',(-39.7908689233158,-32.9683538966935,3.64861123097266));
#9034=CARTESIAN_POINT('Ctrl Pts',(-42.3806431125633,-31.7853288297545,3.48982651174697));
#9035=CARTESIAN_POINT('Ctrl Pts',(-42.7909778595383,-28.9678647125816,3.33104179252129));
#9036=CARTESIAN_POINT('Ctrl Pts',(-40.646218478806,-27.0953033985544,3.17225707329561));
#9037=CARTESIAN_POINT('Ctrl Pts',(-37.9098567596893,-27.881943844822,3.01347235406992));
#9038=CARTESIAN_POINT('Ctrl Pts',(-37.0869866417049,-30.6076297028158,2.85468763484424));
#9039=CARTESIAN_POINT('Ctrl Pts',(-38.9309321484219,-32.777040624953,2.69590291561856));
#9040=CARTESIAN_POINT('Ctrl Pts',(-41.7535915815893,-32.4041166904058,2.53711819639287));
#9041=CARTESIAN_POINT('Ctrl Pts',(-42.9708669527046,-29.830263717713,2.37833347716719));
#9042=CARTESIAN_POINT('Ctrl Pts',(-41.4683625791277,-27.4118013520306,2.21954875794151));
#9043=CARTESIAN_POINT('Ctrl Pts',(-38.621596771745,-27.3627924042219,2.06076403871582));
#9044=CARTESIAN_POINT('Ctrl Pts',(-37.0367358479852,-29.7281028255258,1.90197931949014));
#9045=CARTESIAN_POINT('Ctrl Pts',(-38.1646953067422,-32.3423318573701,1.74319460026445));
#9046=CARTESIAN_POINT('Ctrl Pts',(-40.9728438931775,-32.812192293083,1.58440988103877));
#9047=CARTESIAN_POINT('Ctrl Pts',(-42.8903739628085,-30.707542080798,1.42562516181309));
#9048=CARTESIAN_POINT('Ctrl Pts',(-42.1618064338936,-27.9551389132726,1.2668404425874));
#9049=CARTESIAN_POINT('Ctrl Pts',(-39.454156767702,-27.0747919996342,1.10805572336172));
#9050=CARTESIAN_POINT('Ctrl Pts',(-37.2461857259263,-28.8723853276339,0.949271004136036));
#9051=CARTESIAN_POINT('Ctrl Pts',(-37.5593497462198,-31.7023698699528,0.790486284910354));
#9052=CARTESIAN_POINT('Ctrl Pts',(-40.1067617676959,-32.9737059237326,0.63170156568467));
#9053=CARTESIAN_POINT('Ctrl Pts',(-42.5566887710618,-31.5229768750616,0.472916846458986));
#9054=CARTESIAN_POINT('Ctrl Pts',(-42.6655029077533,-28.6773613681587,0.314132127233303));
#9055=CARTESIAN_POINT('Ctrl Pts',(-40.3351050630486,-27.0438515966452,0.155347408007618));
#9056=CARTESIAN_POINT('Ctrl Pts',(-37.6958995373424,-28.1141315210005,-0.00343731121806404));
#9057=CARTESIAN_POINT('Ctrl Pts',(-37.1701534642436,-30.9160962288461,-0.162222030443749));
#9058=CARTESIAN_POINT('Ctrl Pts',(-38.5409902294193,-32.2158576312381,-0.268078509927538));
#9059=CARTESIAN_POINT('Ctrl Pts',(-39.3498000020249,-32.4320868020351,-0.321006749669432));
#9060=CARTESIAN_POINT('Ctrl Pts',(-37.9456684496579,-28.2435746787731,10.1070022498898));
#9061=CARTESIAN_POINT('Ctrl Pts',(-37.3615552660859,-28.9267589437008,10.0540740101479));
#9062=CARTESIAN_POINT('Ctrl Pts',(-36.9391183154699,-30.9104128771509,9.94821753066413));
#9063=CARTESIAN_POINT('Ctrl Pts',(-39.1082748967234,-33.0697809625963,9.78943281143844));
#9064=CARTESIAN_POINT('Ctrl Pts',(-42.0942485534896,-32.41172206748,9.63064809221276));
#9065=CARTESIAN_POINT('Ctrl Pts',(-43.1627106886284,-29.5492281554804,9.47186337298707));
#9066=CARTESIAN_POINT('Ctrl Pts',(-41.335897389088,-27.09768538351,9.3130786537614));
#9067=CARTESIAN_POINT('Ctrl Pts',(-38.2860248054076,-27.3040258626292,9.1542939345357));
#9068=CARTESIAN_POINT('Ctrl Pts',(-36.8053019100774,-29.978054476698,8.99550921531003));
#9069=CARTESIAN_POINT('Ctrl Pts',(-38.249255461304,-32.6723899859121,8.83672449608433));
#9070=CARTESIAN_POINT('Ctrl Pts',(-41.2959951694642,-32.9200883891015,8.67793977685867));
#9071=CARTESIAN_POINT('Ctrl Pts',(-43.1562684764051,-30.4945482966316,8.51915505763297));
#9072=CARTESIAN_POINT('Ctrl Pts',(-42.1270322513865,-27.6162302758946,8.36037033840729));
#9073=CARTESIAN_POINT('Ctrl Pts',(-39.1505320759499,-26.920227645135,8.20158561918161));
#9074=CARTESIAN_POINT('Ctrl Pts',(-36.9517062837778,-29.0436989274726,8.04280089995592));
#9075=CARTESIAN_POINT('Ctrl Pts',(-37.5435427674391,-32.0426514504762,7.88401618073024));
#9076=CARTESIAN_POINT('Ctrl Pts',(-40.3842254020444,-33.1715886080345,7.72523146150456));
#9077=CARTESIAN_POINT('Ctrl Pts',(-42.8731559614695,-31.3969896409542,7.56644674227887));
#9078=CARTESIAN_POINT('Ctrl Pts',(-42.7317597337645,-28.3434693071248,7.40766202305319));
#9079=CARTESIAN_POINT('Ctrl Pts',(-40.0894825795227,-26.806475672183,7.24887730382751));
#9080=CARTESIAN_POINT('Ctrl Pts',(-37.3652856102805,-28.1931006977328,7.09009258460182));
#9081=CARTESIAN_POINT('Ctrl Pts',(-37.0531261372968,-31.2339122396802,6.93130786537614));
#9082=CARTESIAN_POINT('Ctrl Pts',(-39.4387810077596,-33.145097482549,6.77252314615045));
#9083=CARTESIAN_POINT('Ctrl Pts',(-42.3382225936864,-32.1769979480524,6.61373842692477));
#9084=CARTESIAN_POINT('Ctrl Pts',(-43.0970600211537,-29.2158927476094,6.45495370769909));
#9085=CARTESIAN_POINT('Ctrl Pts',(-41.0205901599018,-26.9726247872904,6.29616898847341));
#9086=CARTESIAN_POINT('Ctrl Pts',(-38.0097868667106,-27.5008688227433,6.13738426924772));
#9087=CARTESIAN_POINT('Ctrl Pts',(-36.8209908202787,-30.3170261682078,5.97859955002204));
#9088=CARTESIAN_POINT('Ctrl Pts',(-38.5425251632707,-32.8429512932687,5.81981483079635));
#9089=CARTESIAN_POINT('Ctrl Pts',(-41.598353642974,-32.7662014727955,5.66103011157068));
#9090=CARTESIAN_POINT('Ctrl Pts',(-43.1909157660438,-30.1570398992684,5.50224539234498));
#9091=CARTESIAN_POINT('Ctrl Pts',(-41.8622472166279,-27.4041108921859,5.34346067311931));
#9092=CARTESIAN_POINT('Ctrl Pts',(-38.8287221031988,-27.0276754813048,5.18467595389362));
#9093=CARTESIAN_POINT('Ctrl Pts',(-36.8674825557338,-29.3723540669221,5.02589123466794));
#9094=CARTESIAN_POINT('Ctrl Pts',(-37.7740109818545,-32.291632136063,4.86710651544225));
#9095=CARTESIAN_POINT('Ctrl Pts',(-40.7183955825647,-33.1129588405443,4.70832179621657));
#9096=CARTESIAN_POINT('Ctrl Pts',(-43.0051008947389,-31.0844231500414,4.54953707699088));
#9097=CARTESIAN_POINT('Ctrl Pts',(-42.5406859796171,-28.0631159794849,4.3907523577652));
#9098=CARTESIAN_POINT('Ctrl Pts',(-39.7503150201867,-26.8149941339207,4.23196763853952));
#9099=CARTESIAN_POINT('Ctrl Pts',(-37.1885265352497,-28.4826925451306,4.07318291931384));
#9100=CARTESIAN_POINT('Ctrl Pts',(-37.2005955639047,-31.5394608664239,3.91439820008815));
#9101=CARTESIAN_POINT('Ctrl Pts',(-39.7754731101895,-33.1868781954769,3.75561348086247));
#9102=CARTESIAN_POINT('Ctrl Pts',(-42.5559013145607,-31.9167611805448,3.59682876163678));
#9103=CARTESIAN_POINT('Ctrl Pts',(-42.9964440879267,-28.891880969476,3.4380440424111));
#9104=CARTESIAN_POINT('Ctrl Pts',(-40.6937917954847,-26.8814654229962,3.27925932318542));
#9105=CARTESIAN_POINT('Ctrl Pts',(-37.755984579403,-27.7260167713657,3.12047460395974));
#9106=CARTESIAN_POINT('Ctrl Pts',(-36.8725364030803,-30.6523621907026,2.96168988473405));
#9107=CARTESIAN_POINT('Ctrl Pts',(-38.8522295035391,-32.9814808219043,2.80290516550837));
#9108=CARTESIAN_POINT('Ctrl Pts',(-41.8826874994131,-32.5811029704277,2.64412044628268));
#9109=CARTESIAN_POINT('Ctrl Pts',(-43.1895762576637,-29.8177680708476,2.485335727057));
#9110=CARTESIAN_POINT('Ctrl Pts',(-41.5764605061711,-27.2212633251162,2.32655100783131));
#9111=CARTESIAN_POINT('Ctrl Pts',(-38.5201214728493,-27.1686464362308,2.16776628860563));
#9112=CARTESIAN_POINT('Ctrl Pts',(-36.8185862460626,-29.7080862973553,2.00898156937995));
#9113=CARTESIAN_POINT('Ctrl Pts',(-38.0295838324686,-32.5147696611037,1.85019685015426));
#9114=CARTESIAN_POINT('Ctrl Pts',(-41.0444627219901,-33.0192202857946,1.69141213092858));
#9115=CARTESIAN_POINT('Ctrl Pts',(-43.1031575342513,-30.7596299188548,1.5326274117029));
#9116=CARTESIAN_POINT('Ctrl Pts',(-42.3209543156871,-27.8046003148985,1.37384269247721));
#9117=CARTESIAN_POINT('Ctrl Pts',(-39.4139728766517,-26.8594440157609,1.21505797325153));
#9118=CARTESIAN_POINT('Ctrl Pts',(-37.0434554066433,-28.789372582472,1.05627325402585));
#9119=CARTESIAN_POINT('Ctrl Pts',(-37.3796739380633,-31.8276949474362,0.897488534800165));
#9120=CARTESIAN_POINT('Ctrl Pts',(-40.1146213562876,-33.1926242280815,0.738703815574481));
#9121=CARTESIAN_POINT('Ctrl Pts',(-42.7449071036286,-31.6350953977407,0.579919096348796));
#9122=CARTESIAN_POINT('Ctrl Pts',(-42.8617319202273,-28.5799913477279,0.421134377123115));
#9123=CARTESIAN_POINT('Ctrl Pts',(-40.3597748300205,-26.8262258419593,0.262349657897428));
#9124=CARTESIAN_POINT('Ctrl Pts',(-37.5262762527031,-27.9752976415799,0.103564938671747));
#9125=CARTESIAN_POINT('Ctrl Pts',(-36.9618258013664,-30.9835374076926,-0.0552197805539386));
#9126=CARTESIAN_POINT('Ctrl Pts',(-38.4335808375037,-32.3789846544712,-0.161076260037727));
#9127=CARTESIAN_POINT('Ctrl Pts',(-39.301933573839,-32.6111321859386,-0.214004499779622));
#9128=CARTESIAN_POINT('Ctrl Pts',(-37.8048028959809,-28.1231365609212,10.2140044997796));
#9129=CARTESIAN_POINT('Ctrl Pts',(-37.1806370602456,-28.8531667839546,10.1610762600377));
#9130=CARTESIAN_POINT('Ctrl Pts',(-36.7292335998507,-30.9728399055403,10.0552197805539));
#9131=CARTESIAN_POINT('Ctrl Pts',(-39.0471292893458,-33.2802759018827,9.89643506132826));
#9132=CARTESIAN_POINT('Ctrl Pts',(-42.2378512168355,-32.577093895749,9.73765034210256));
#9133=CARTESIAN_POINT('Ctrl Pts',(-43.3795778210052,-29.5183187214848,9.5788656228769));
#9134=CARTESIAN_POINT('Ctrl Pts',(-41.4274998985944,-26.8986736147774,9.4200809036512));
#9135=CARTESIAN_POINT('Ctrl Pts',(-38.1684974935506,-27.1191628644941,9.26129618442552));
#9136=CARTESIAN_POINT('Ctrl Pts',(-36.5862414009823,-29.9765496717457,9.10251146519984));
#9137=CARTESIAN_POINT('Ctrl Pts',(-38.1292068748188,-32.8556358183309,8.94372674597415));
#9138=CARTESIAN_POINT('Ctrl Pts',(-41.3848615830082,-33.1203189057619,8.78494202674847));
#9139=CARTESIAN_POINT('Ctrl Pts',(-43.3726938661667,-30.5284594827854,8.6261573075228));
#9140=CARTESIAN_POINT('Ctrl Pts',(-42.2728828935239,-27.4527751403451,8.4673725882971));
#9141=CARTESIAN_POINT('Ctrl Pts',(-39.0922840441595,-26.7090475958899,8.30858786907142));
#9142=CARTESIAN_POINT('Ctrl Pts',(-36.7426847253861,-28.9781253446489,8.14980314984574));
#9143=CARTESIAN_POINT('Ctrl Pts',(-37.3751034480454,-32.1827160994822,7.99101843062005));
#9144=CARTESIAN_POINT('Ctrl Pts',(-40.4105717452074,-33.3890644995146,7.83223371139437));
#9145=CARTESIAN_POINT('Ctrl Pts',(-43.07016832067,-31.492781247339,7.67344899216868));
#9146=CARTESIAN_POINT('Ctrl Pts',(-42.9190765509283,-28.2298809658486,7.514664272943));
#9147=CARTESIAN_POINT('Ctrl Pts',(-40.0956184017111,-26.587495647978,7.35587955371732));
#9148=CARTESIAN_POINT('Ctrl Pts',(-37.1846231942129,-28.0692015780361,7.19709483449163));
#9149=CARTESIAN_POINT('Ctrl Pts',(-36.8510589401995,-31.3185216255423,7.03831011526596));
#9150=CARTESIAN_POINT('Ctrl Pts',(-39.4002982107335,-33.3607568770483,6.87952539604026));
#9151=CARTESIAN_POINT('Ctrl Pts',(-42.4985545616324,-32.3262747389653,6.72074067681459));
#9152=CARTESIAN_POINT('Ctrl Pts',(-43.3094254860068,-29.1621264983242,6.56195595758889));
#9153=CARTESIAN_POINT('Ctrl Pts',(-41.0905720466756,-26.7650376110844,6.40317123836323));
#9154=CARTESIAN_POINT('Ctrl Pts',(-37.8733179141165,-27.3295033501461,6.24438651913752));
#9155=CARTESIAN_POINT('Ctrl Pts',(-36.6030061000561,-30.338764658622,6.08560179991185));
#9156=CARTESIAN_POINT('Ctrl Pts',(-38.4425860858555,-33.0378925177933,5.92681708068616));
#9157=CARTESIAN_POINT('Ctrl Pts',(-41.7079527828264,-32.9558799606631,5.76803236146049));
#9158=CARTESIAN_POINT('Ctrl Pts',(-43.4097169211181,-30.1678081281632,5.60924764223479));
#9159=CARTESIAN_POINT('Ctrl Pts',(-41.9899415438703,-27.2261107264408,5.45046292300912));
#9160=CARTESIAN_POINT('Ctrl Pts',(-38.7484075554253,-26.8238631322397,5.29167820378342));
#9161=CARTESIAN_POINT('Ctrl Pts',(-36.6526857747,-29.3293163732931,5.13289348455775));
#9162=CARTESIAN_POINT('Ctrl Pts',(-37.6213748723289,-32.4487693954391,4.97410876533206));
#9163=CARTESIAN_POINT('Ctrl Pts',(-40.7676559813938,-33.326414487747,4.81532404610638));
#9164=CARTESIAN_POINT('Ctrl Pts',(-43.2111607205359,-31.1587820661693,4.65653932688069));
#9165=CARTESIAN_POINT('Ctrl Pts',(-42.7149008658065,-27.9303038051732,4.49775460765502));
#9166=CARTESIAN_POINT('Ctrl Pts',(-39.733194116348,-26.5965982207998,4.33896988842933));
#9167=CARTESIAN_POINT('Ctrl Pts',(-36.9957437460284,-28.3786507439458,4.18018516920365));
#9168=CARTESIAN_POINT('Ctrl Pts',(-37.0086403482089,-31.6450217274626,4.02140044997796));
#9169=CARTESIAN_POINT('Ctrl Pts',(-39.7600772970632,-33.4054024942603,3.86261573075228));
#9170=CARTESIAN_POINT('Ctrl Pts',(-42.7311595165581,-32.0481935313351,3.70383101152659));
#9171=CARTESIAN_POINT('Ctrl Pts',(-43.201910316315,-28.8158972263705,3.54504629230092));
#9172=CARTESIAN_POINT('Ctrl Pts',(-40.7413651121635,-26.6676274474379,3.38626157307523));
#9173=CARTESIAN_POINT('Ctrl Pts',(-37.6021123991165,-27.5700896979093,3.22747685384955));
#9174=CARTESIAN_POINT('Ctrl Pts',(-36.6580861644558,-30.6970946785895,3.06869213462386));
#9175=CARTESIAN_POINT('Ctrl Pts',(-38.7735268586563,-33.1859210188555,2.90990741539818));
#9176=CARTESIAN_POINT('Ctrl Pts',(-42.0117834172368,-32.7580892504496,2.7511226961725));
#9177=CARTESIAN_POINT('Ctrl Pts',(-43.4082855626228,-29.805272423982,2.59233797694681));
#9178=CARTESIAN_POINT('Ctrl Pts',(-41.6845584332144,-27.0307252982018,2.43355325772113));
#9179=CARTESIAN_POINT('Ctrl Pts',(-38.4186461739536,-26.9745004682398,2.27476853849544));
#9180=CARTESIAN_POINT('Ctrl Pts',(-36.6004366441401,-29.6880697691848,2.11598381926976));
#9181=CARTESIAN_POINT('Ctrl Pts',(-37.894472358195,-32.6872074648372,1.95719910004408));
#9182=CARTESIAN_POINT('Ctrl Pts',(-41.1160815508026,-33.2262482785062,1.79841438081839));
#9183=CARTESIAN_POINT('Ctrl Pts',(-43.315941105694,-30.8117177569115,1.63962966159271));
#9184=CARTESIAN_POINT('Ctrl Pts',(-42.4801021974805,-27.6540617165245,1.48084494236703));
#9185=CARTESIAN_POINT('Ctrl Pts',(-39.3737889856013,-26.6440960318875,1.32206022314134));
#9186=CARTESIAN_POINT('Ctrl Pts',(-36.8407250873603,-28.7063598373101,1.16327550391566));
#9187=CARTESIAN_POINT('Ctrl Pts',(-37.1999981299068,-31.9530200249197,1.00449078468997));
#9188=CARTESIAN_POINT('Ctrl Pts',(-40.1224809448793,-33.4115425324305,0.845706065464292));
#9189=CARTESIAN_POINT('Ctrl Pts',(-42.9331254361953,-31.7472139204198,0.686921346238607));
#9190=CARTESIAN_POINT('Ctrl Pts',(-43.0579609327015,-28.4826213272971,0.528136627012925));
#9191=CARTESIAN_POINT('Ctrl Pts',(-40.3844445969923,-26.6086000872734,0.369351907787239));
#9192=CARTESIAN_POINT('Ctrl Pts',(-37.3566529680639,-27.8364637621594,0.210567188561558));
#9193=CARTESIAN_POINT('Ctrl Pts',(-36.7534981384891,-31.0509785865391,0.0517824693358723));
#9194=CARTESIAN_POINT('Ctrl Pts',(-38.326171445588,-32.5421116777044,-0.0540740101479163));
#9195=CARTESIAN_POINT('Ctrl Pts',(-39.2540671456531,-32.7901775698422,-0.107002249889811));
#9196=CARTESIAN_POINT('Ctrl Pts',(-37.6639373423038,-28.0026984430693,10.3210067496694));
#9197=CARTESIAN_POINT('Ctrl Pts',(-36.9997188544053,-28.7795746242084,10.2680785099275));
#9198=CARTESIAN_POINT('Ctrl Pts',(-36.5193488842315,-31.0352669339298,10.1622220304438));
#9199=CARTESIAN_POINT('Ctrl Pts',(-38.9859836819681,-33.490770841169,10.0034373112181));
#9200=CARTESIAN_POINT('Ctrl Pts',(-42.3814538801814,-32.7424657240179,9.84465259199238));
#9201=CARTESIAN_POINT('Ctrl Pts',(-43.596444953382,-29.4874092874893,9.6858678727667));
#9202=CARTESIAN_POINT('Ctrl Pts',(-41.5191024081009,-26.6996618460447,9.52708315354101));
#9203=CARTESIAN_POINT('Ctrl Pts',(-38.0509701816934,-26.934299866359,9.36829843431533));
#9204=CARTESIAN_POINT('Ctrl Pts',(-36.3671808918873,-29.9750448667934,9.20951371508965));
#9205=CARTESIAN_POINT('Ctrl Pts',(-38.0091582883336,-33.0388816507496,9.05072899586396));
#9206=CARTESIAN_POINT('Ctrl Pts',(-41.4737279965523,-33.3205494224222,8.89194427663828));
#9207=CARTESIAN_POINT('Ctrl Pts',(-43.5891192559282,-30.562370668939,8.73315955741259));
#9208=CARTESIAN_POINT('Ctrl Pts',(-42.4187335356612,-27.2893200047958,8.57437483818692));
#9209=CARTESIAN_POINT('Ctrl Pts',(-39.0340360123693,-26.4978675466446,8.41559011896124));
#9210=CARTESIAN_POINT('Ctrl Pts',(-36.5336631669943,-28.9125517618253,8.25680539973554));
#9211=CARTESIAN_POINT('Ctrl Pts',(-37.2066641286517,-32.3227807484881,8.09802068050986));
#9212=CARTESIAN_POINT('Ctrl Pts',(-40.4369180883703,-33.6065403909949,7.93923596128418));
#9213=CARTESIAN_POINT('Ctrl Pts',(-43.2671806798705,-31.5885728537237,7.7804512420585));
#9214=CARTESIAN_POINT('Ctrl Pts',(-43.1063933680922,-28.1162926245723,7.62166652283281));
#9215=CARTESIAN_POINT('Ctrl Pts',(-40.1017542238995,-26.368515623773,7.46288180360714));
#9216=CARTESIAN_POINT('Ctrl Pts',(-37.0039607781453,-27.9453024583394,7.30409708438144));
#9217=CARTESIAN_POINT('Ctrl Pts',(-36.6489917431023,-31.4031310114043,7.14531236515577));
#9218=CARTESIAN_POINT('Ctrl Pts',(-39.3618154137075,-33.5764162715476,6.98652764593008));
#9219=CARTESIAN_POINT('Ctrl Pts',(-42.6588865295783,-32.4755515298782,6.82774292670439));
#9220=CARTESIAN_POINT('Ctrl Pts',(-43.5217909508599,-29.1083602490389,6.66895820747872));
#9221=CARTESIAN_POINT('Ctrl Pts',(-41.1605539334494,-26.5574504348784,6.51017348825302));
#9222=CARTESIAN_POINT('Ctrl Pts',(-37.7368489615224,-27.1581378775489,6.35138876902735));
#9223=CARTESIAN_POINT('Ctrl Pts',(-36.3850213798334,-30.3605031490362,6.19260404980165));
#9224=CARTESIAN_POINT('Ctrl Pts',(-38.3426470084403,-33.2328337423178,6.03381933057598));
#9225=CARTESIAN_POINT('Ctrl Pts',(-41.8175519226788,-33.1455584485307,5.87503461135029));
#9226=CARTESIAN_POINT('Ctrl Pts',(-43.6285180761925,-30.1785763570579,5.71624989212461));
#9227=CARTESIAN_POINT('Ctrl Pts',(-42.1176358711127,-27.0481105606956,5.55746517289893));
#9228=CARTESIAN_POINT('Ctrl Pts',(-38.6680930076518,-26.6200507831746,5.39868045367324));
#9229=CARTESIAN_POINT('Ctrl Pts',(-36.4378889936663,-29.286278679664,5.23989573444756));
#9230=CARTESIAN_POINT('Ctrl Pts',(-37.4687387628032,-32.6059066548152,5.08111101522187));
#9231=CARTESIAN_POINT('Ctrl Pts',(-40.8169163802229,-33.5398701349496,4.92232629599619));
#9232=CARTESIAN_POINT('Ctrl Pts',(-43.4172205463328,-31.2331409822972,4.76354157677051));
#9233=CARTESIAN_POINT('Ctrl Pts',(-42.889115751996,-27.7974916308615,4.60475685754482));
#9234=CARTESIAN_POINT('Ctrl Pts',(-39.7160732125092,-26.378202307679,4.44597213831914));
#9235=CARTESIAN_POINT('Ctrl Pts',(-36.8029609568071,-28.274608942761,4.28718741909346));
#9236=CARTESIAN_POINT('Ctrl Pts',(-36.8166851325132,-31.7505825885012,4.12840269986777));
#9237=CARTESIAN_POINT('Ctrl Pts',(-39.7446814839369,-33.6239267930437,3.96961798064209));
#9238=CARTESIAN_POINT('Ctrl Pts',(-42.9064177185554,-32.1796258821253,3.8108332614164));
#9239=CARTESIAN_POINT('Ctrl Pts',(-43.4073765447034,-28.7399134832649,3.65204854219072));
#9240=CARTESIAN_POINT('Ctrl Pts',(-40.7889384288422,-26.4537894718797,3.49326382296504));
#9241=CARTESIAN_POINT('Ctrl Pts',(-37.4482402188302,-27.414162624453,3.33447910373936));
#9242=CARTESIAN_POINT('Ctrl Pts',(-36.4436359258312,-30.7418271664764,3.17569438451367));
#9243=CARTESIAN_POINT('Ctrl Pts',(-38.6948242137735,-33.3903612158066,3.01690966528799));
#9244=CARTESIAN_POINT('Ctrl Pts',(-42.1408793350605,-32.9350755304716,2.85812494606231));
#9245=CARTESIAN_POINT('Ctrl Pts',(-43.6269948675819,-29.7927767771166,2.69934022683662));
#9246=CARTESIAN_POINT('Ctrl Pts',(-41.7926563602578,-26.8401872712874,2.54055550761094));
#9247=CARTESIAN_POINT('Ctrl Pts',(-38.3171708750578,-26.7803545002487,2.38177078838525));
#9248=CARTESIAN_POINT('Ctrl Pts',(-36.3822870422175,-29.6680532410143,2.22298606915957));
#9249=CARTESIAN_POINT('Ctrl Pts',(-37.7593608839214,-32.8596452685709,2.06420134993389));
#9250=CARTESIAN_POINT('Ctrl Pts',(-41.1877003796151,-33.4332762712177,1.9054166307082));
#9251=CARTESIAN_POINT('Ctrl Pts',(-43.5287246771368,-30.8638055949683,1.74663191148252));
#9252=CARTESIAN_POINT('Ctrl Pts',(-42.6392500792739,-27.5035231181503,1.58784719225684));
#9253=CARTESIAN_POINT('Ctrl Pts',(-39.333605094551,-26.4287480480142,1.42906247303115));
#9254=CARTESIAN_POINT('Ctrl Pts',(-36.6379947680772,-28.6233470921482,1.27027775380547));
#9255=CARTESIAN_POINT('Ctrl Pts',(-37.0203223217504,-32.078345102403,1.11149303457979));
#9256=CARTESIAN_POINT('Ctrl Pts',(-40.1303405334711,-33.6304608367794,0.952708315354102));
#9257=CARTESIAN_POINT('Ctrl Pts',(-43.1213437687621,-31.859332443099,0.793923596128418));
#9258=CARTESIAN_POINT('Ctrl Pts',(-43.2541899451756,-28.3852513068663,0.635138876902736));
#9259=CARTESIAN_POINT('Ctrl Pts',(-40.4091143639642,-26.3909743325875,0.47635415767705));
#9260=CARTESIAN_POINT('Ctrl Pts',(-37.1870296834247,-27.6976298827388,0.317569438451369));
#9261=CARTESIAN_POINT('Ctrl Pts',(-36.5451704756118,-31.1184197653857,0.158784719225683));
#9262=CARTESIAN_POINT('Ctrl Pts',(-38.2187620536724,-32.7052387009375,0.0529282397418946));
#9263=CARTESIAN_POINT('Ctrl Pts',(-39.2062007174671,-32.9692229537457,0.));
#9264=CARTESIAN_POINT('Ctrl Pts',(-39.2062007174671,-32.9692229537457,0.));
#9265=CARTESIAN_POINT('Ctrl Pts',(-39.1131466107856,-32.9351833458516,-1.6060879670377E-16));
#9266=CARTESIAN_POINT('Ctrl Pts',(-39.0221597277766,-32.8963742919489,-4.44513565583088E-16));
#9267=CARTESIAN_POINT('Ctrl Pts',(-38.9334478499662,-32.8531245205888,-6.10622663543836E-16));
#9268=CARTESIAN_POINT('Ctrl Pts',(-38.8427661867135,-32.8089144181874,-7.80420098298495E-16));
#9269=CARTESIAN_POINT('Ctrl Pts',(-38.7544610131422,-32.760063585673,-3.00700937848116E-15));
#9270=CARTESIAN_POINT('Ctrl Pts',(-38.6687831978432,-32.7068775858309,-3.05311331771918E-15));
#9271=CARTESIAN_POINT('Ctrl Pts',(-38.5858338035881,-32.655385300992,-3.09774907108449E-15));
#9272=CARTESIAN_POINT('Ctrl Pts',(-38.5053467696029,-32.5998286976775,-1.98203717691243E-15));
#9273=CARTESIAN_POINT('Ctrl Pts',(-38.4275834630713,-32.5404543773605,-2.16493489801906E-15));
#9274=CARTESIAN_POINT('Ctrl Pts',(-38.3595405698561,-32.4885018470831,-2.32497040398736E-15));
#9275=CARTESIAN_POINT('Ctrl Pts',(-38.2935833272372,-32.4336256602705,1.05568646747328E-15));
#9276=CARTESIAN_POINT('Ctrl Pts',(-38.2299120950925,-32.3759780448687,2.27595720048157E-15));
#9277=CARTESIAN_POINT('Ctrl Pts',(-38.2165695179232,-32.363897742176,2.53167011625481E-15));
#9278=CARTESIAN_POINT('Ctrl Pts',(-38.2033255561917,-32.3516938355638,-1.36442326856797E-15));
#9279=CARTESIAN_POINT('Ctrl Pts',(-38.1901992329768,-32.3393840298394,-1.38777878078145E-15));
#9280=CARTESIAN_POINT('Ctrl Pts',(-38.1177716356207,-32.2714617611321,-1.51664835125835E-15));
#9281=CARTESIAN_POINT('Ctrl Pts',(-38.0488097561366,-32.2002182797225,-1.51379216107608E-15));
#9282=CARTESIAN_POINT('Ctrl Pts',(-37.9835529381418,-32.125944757074,-1.16573417585641E-15));
#9283=CARTESIAN_POINT('Ctrl Pts',(-37.9186574569704,-32.0520824980997,-8.19603440089208E-16));
#9284=CARTESIAN_POINT('Ctrl Pts',(-37.8574256347879,-31.9752228624939,6.49623181554391E-16));
#9285=CARTESIAN_POINT('Ctrl Pts',(-37.8001364752534,-31.8956254663677,3.33066907387547E-16));
#9286=CARTESIAN_POINT('Ctrl Pts',(-37.7442813766686,-31.8180205504665,2.44346627378703E-17));
#9287=CARTESIAN_POINT('Ctrl Pts',(-37.6921737559928,-31.7378124817103,9.32925077816174E-16));
#9288=CARTESIAN_POINT('Ctrl Pts',(-37.6441190472323,-31.6552277434766,1.16573417585641E-15));
#9289=CARTESIAN_POINT('Ctrl Pts',(-37.6233914631522,-31.619606216479,1.26615243410233E-15));
#9290=CARTESIAN_POINT('Ctrl Pts',(-37.6034185407569,-31.5835423973841,-2.77132270277859E-15));
#9291=CARTESIAN_POINT('Ctrl Pts',(-37.584227773746,-31.5470541286155,-3.08086889333481E-15));
#9292=CARTESIAN_POINT('Ctrl Pts',(-37.5705624211823,-31.5210715789405,-3.30129040261011E-15));
#9293=CARTESIAN_POINT('Ctrl Pts',(-37.5572937042546,-31.4948738056765,1.83855327584014E-15));
#9294=CARTESIAN_POINT('Ctrl Pts',(-37.5444321465139,-31.4684672473934,1.80411241501588E-15));
#9295=CARTESIAN_POINT('Ctrl Pts',(-37.5388166481749,-31.4569378520303,1.78907515431618E-15));
#9296=CARTESIAN_POINT('Ctrl Pts',(-37.5332796940573,-31.4453704534221,7.2015229496451E-16));
#9297=CARTESIAN_POINT('Ctrl Pts',(-37.5278258543441,-31.4337738641374,6.38378239159465E-16));
#9298=CARTESIAN_POINT('Ctrl Pts',(-37.487598010987,-31.3482367376823,3.52079810388171E-17));
#9299=CARTESIAN_POINT('Ctrl Pts',(-37.4518262054158,-31.2609864756373,-4.26555916893969E-15));
#9300=CARTESIAN_POINT('Ctrl Pts',(-37.4207614166239,-31.1722603981052,-3.63598040564739E-15));
#9301=CARTESIAN_POINT('Ctrl Pts',(-37.3903833382621,-31.085495676991,-3.0203189526013E-15));
#9302=CARTESIAN_POINT('Ctrl Pts',(-37.3645062551562,-30.9973189926276,-6.38813711439151E-16));
#9303=CARTESIAN_POINT('Ctrl Pts',(-37.3434139855678,-30.9079434560133,-1.60982338570648E-15));
#9304=CARTESIAN_POINT('Ctrl Pts',(-37.3396853045659,-30.8921436927865,-1.7814779964148E-15));
#9305=CARTESIAN_POINT('Ctrl Pts',(-37.3361062849538,-30.8763064560273,-1.28296660226899E-15));
#9306=CARTESIAN_POINT('Ctrl Pts',(-37.3326786669098,-30.8604329174724,-1.2490009027033E-15));
#9307=CARTESIAN_POINT('Ctrl Pts',(-37.3125677659889,-30.7672979307153,-1.02302944293106E-15));
#9308=CARTESIAN_POINT('Ctrl Pts',(-37.2976648337907,-30.6729122002239,-7.87763452680115E-16));
#9309=CARTESIAN_POINT('Ctrl Pts',(-37.2878913789518,-30.5776846228188,-2.22044604925031E-16));
#9310=CARTESIAN_POINT('Ctrl Pts',(-37.2846134893309,-30.5457465320667,-3.23098621953069E-17));
#9311=CARTESIAN_POINT('Ctrl Pts',(-37.2819130028101,-30.513713867855,-1.58807512465196E-15));
#9312=CARTESIAN_POINT('Ctrl Pts',(-37.2797881830403,-30.4816025255615,-1.66533453693773E-15));
#9313=CARTESIAN_POINT('Ctrl Pts',(-37.2785995619339,-30.4636394871208,-1.70855334044072E-15));
#9314=CARTESIAN_POINT('Ctrl Pts',(-37.2775910929928,-30.4456518334769,1.44829596815902E-15));
#9315=CARTESIAN_POINT('Ctrl Pts',(-37.2767625516214,-30.4276423921194,1.77635683940025E-15));
#9316=CARTESIAN_POINT('Ctrl Pts',(-37.276188285258,-30.4151599540007,2.00373754728324E-15));
#9317=CARTESIAN_POINT('Ctrl Pts',(-37.2757005703862,-30.4026685786166,-6.72593298636936E-16));
#9318=CARTESIAN_POINT('Ctrl Pts',(-37.2752994571504,-30.3901786876117,-5.82867087928207E-16));
#9319=CARTESIAN_POINT('Ctrl Pts',(-37.2723066310671,-30.2969878670748,8.66070649168054E-17));
#9320=CARTESIAN_POINT('Ctrl Pts',(-37.2741233925594,-30.2037325944215,1.1534185885948E-15));
#9321=CARTESIAN_POINT('Ctrl Pts',(-37.280610638584,-30.1107879986708,1.01307850997046E-15));
#9322=CARTESIAN_POINT('Ctrl Pts',(-37.2871108431702,-30.0176577419689,8.72458095816411E-16));
#9323=CARTESIAN_POINT('Ctrl Pts',(-37.2983005933798,-29.9248384229594,-3.4945567965877E-15));
#9324=CARTESIAN_POINT('Ctrl Pts',(-37.314090996424,-29.8327194250238,-2.87270207621759E-15));
#9325=CARTESIAN_POINT('Ctrl Pts',(-37.3296582910756,-29.7419020101763,-2.25963376913325E-15));
#9326=CARTESIAN_POINT('Ctrl Pts',(-37.3496976162604,-29.6517644189367,7.72310224401951E-16));
#9327=CARTESIAN_POINT('Ctrl Pts',(-37.3741668412413,-29.5627049129401,1.0547118733939E-15));
#9328=CARTESIAN_POINT('Ctrl Pts',(-37.3836805051461,-29.5280784706137,1.1645099718931E-15));
#9329=CARTESIAN_POINT('Ctrl Pts',(-37.3938642491001,-29.4936153373462,-7.07244990223136E-16));
#9330=CARTESIAN_POINT('Ctrl Pts',(-37.4047171636237,-29.4593403829489,-6.10622663543836E-16));
#9331=CARTESIAN_POINT('Ctrl Pts',(-37.4105213799507,-29.4410098921402,-5.58948352016791E-16));
#9332=CARTESIAN_POINT('Ctrl Pts',(-37.4165170058423,-29.422733239581,1.26908615097469E-15));
#9333=CARTESIAN_POINT('Ctrl Pts',(-37.4227039978848,-29.4045143438212,1.13797860024079E-15));
#9334=CARTESIAN_POINT('Ctrl Pts',(-37.4281525928791,-29.3884698130449,1.02251830228993E-15));
#9335=CARTESIAN_POINT('Ctrl Pts',(-37.433750081042,-29.3724690012651,1.19736360869678E-15));
#9336=CARTESIAN_POINT('Ctrl Pts',(-37.4394903112345,-29.3565309947013,1.08246744900953E-15));
#9337=CARTESIAN_POINT('Ctrl Pts',(-37.4719157874641,-29.2665002057519,4.33440742784894E-16));
#9338=CARTESIAN_POINT('Ctrl Pts',(-37.5089323079084,-29.1783481505351,-1.87205846606356E-15));
#9339=CARTESIAN_POINT('Ctrl Pts',(-37.5504668382682,-29.0925193983103,-1.58206781009085E-15));
#9340=CARTESIAN_POINT('Ctrl Pts',(-37.581617736038,-29.0281478341417,-1.36457481811132E-15));
#9341=CARTESIAN_POINT('Ctrl Pts',(-37.6153111627318,-28.9650836648662,-1.04020469733639E-15));
#9342=CARTESIAN_POINT('Ctrl Pts',(-37.6515336753454,-28.9035316000466,-5.55111512312578E-17));
#9343=CARTESIAN_POINT('Ctrl Pts',(-37.6664654555227,-28.8781583767379,3.50402920200024E-16));
#9344=CARTESIAN_POINT('Ctrl Pts',(-37.6818271624147,-28.8530423027494,2.30518069273612E-15));
#9345=CARTESIAN_POINT('Ctrl Pts',(-37.6976185122319,-28.8281986233529,2.70616862252382E-15));
#9346=CARTESIAN_POINT('Ctrl Pts',(-37.7070511545528,-28.8133587556787,2.94569062415713E-15));
#9347=CARTESIAN_POINT('Ctrl Pts',(-37.7166324161044,-28.7986234989397,1.52399745346112E-15));
#9348=CARTESIAN_POINT('Ctrl Pts',(-37.7263602579883,-28.7839981748651,1.3392065234541E-15));
#9349=CARTESIAN_POINT('Ctrl Pts',(-37.7738889351269,-28.7125411842724,4.3634764116111E-16));
#9350=CARTESIAN_POINT('Ctrl Pts',(-37.8249264001993,-28.6436861696345,1.61280770038306E-15));
#9351=CARTESIAN_POINT('Ctrl Pts',(-37.8794382711486,-28.5777858428738,1.28022592527088E-15));
#9352=CARTESIAN_POINT('Ctrl Pts',(-37.9310243099595,-28.5154226042852,9.65494912375114E-16));
#9353=CARTESIAN_POINT('Ctrl Pts',(-37.9857222891604,-28.4557051705816,1.05564516917403E-15));
#9354=CARTESIAN_POINT('Ctrl Pts',(-38.0435268618259,-28.3989683289331,2.25470683790086E-15));
#9355=CARTESIAN_POINT('Ctrl Pts',(-38.0564928356052,-28.3862418547597,2.53840998574205E-15));
#9356=CARTESIAN_POINT('Ctrl Pts',(-38.0696151991774,-28.3736655038365,-1.14231766349927E-17));
#9357=CARTESIAN_POINT('Ctrl Pts',(-38.0828907223999,-28.3612406061267,5.55111512312578E-17));
#9358=CARTESIAN_POINT('Ctrl Pts',(-38.0865340033349,-28.364012796625,10.));
#9359=CARTESIAN_POINT('Ctrl Pts',(-38.0249212788374,-28.4219136285024,10.));
#9360=CARTESIAN_POINT('Ctrl Pts',(-37.9666797322405,-28.4829649756762,10.));
#9361=CARTESIAN_POINT('Ctrl Pts',(-37.9118062499715,-28.546782039445,10.));
#9362=CARTESIAN_POINT('Ctrl Pts',(-37.8554800838191,-28.6122885534946,10.));
#9363=CARTESIAN_POINT('Ctrl Pts',(-37.8027022343369,-28.6807095897459,10.));
#9364=CARTESIAN_POINT('Ctrl Pts',(-37.7534948834915,-28.7516775265204,10.));
#9365=CARTESIAN_POINT('Ctrl Pts',(-37.702593238571,-28.825089011926,10.));
#9366=CARTESIAN_POINT('Ctrl Pts',(-37.6555116194557,-28.9012263275327,10.));
#9367=CARTESIAN_POINT('Ctrl Pts',(-37.6123095085901,-28.9797265490615,10.));
#9368=CARTESIAN_POINT('Ctrl Pts',(-37.5934085850863,-29.0140703959804,10.));
#9369=CARTESIAN_POINT('Ctrl Pts',(-37.5752507177294,-29.0488670241427,10.));
#9370=CARTESIAN_POINT('Ctrl Pts',(-37.5578433328344,-29.084088131034,10.));
#9371=CARTESIAN_POINT('Ctrl Pts',(-37.5483351016093,-29.1033265422224,10.));
#9372=CARTESIAN_POINT('Ctrl Pts',(-37.5390508073497,-29.1226916181739,10.));
#9373=CARTESIAN_POINT('Ctrl Pts',(-37.5299918639726,-29.1421788751806,10.));
#9374=CARTESIAN_POINT('Ctrl Pts',(-37.5213418802068,-29.1607863937102,10.));
#9375=CARTESIAN_POINT('Ctrl Pts',(-37.5128948696392,-29.1795113098859,10.));
#9376=CARTESIAN_POINT('Ctrl Pts',(-37.5046661632847,-29.1983169400782,10.));
#9377=CARTESIAN_POINT('Ctrl Pts',(-37.4681053960581,-29.2818717831342,10.));
#9378=CARTESIAN_POINT('Ctrl Pts',(-37.4358048459705,-29.3671100877142,10.));
#9379=CARTESIAN_POINT('Ctrl Pts',(-37.4077887832518,-29.4536330059159,10.));
#9380=CARTESIAN_POINT('Ctrl Pts',(-37.3793104271871,-29.5415836397024,10.));
#9381=CARTESIAN_POINT('Ctrl Pts',(-37.3552586298795,-29.6308623874248,10.));
#9382=CARTESIAN_POINT('Ctrl Pts',(-37.3356979907178,-29.7210874579434,10.));
#9383=CARTESIAN_POINT('Ctrl Pts',(-37.3164756210823,-29.8097522322151,10.));
#9384=CARTESIAN_POINT('Ctrl Pts',(-37.3015901593891,-29.8993317913654,10.));
#9385=CARTESIAN_POINT('Ctrl Pts',(-37.2911456116882,-29.9894866561166,10.));
#9386=CARTESIAN_POINT('Ctrl Pts',(-37.2870154699214,-30.0251370627254,10.));
#9387=CARTESIAN_POINT('Ctrl Pts',(-37.2835802457749,-30.0608776102139,10.));
#9388=CARTESIAN_POINT('Ctrl Pts',(-37.2808483993985,-30.0966878419291,10.));
#9389=CARTESIAN_POINT('Ctrl Pts',(-37.279231497492,-30.1178828960977,10.));
#9390=CARTESIAN_POINT('Ctrl Pts',(-37.2778610197106,-30.13910236557,10.));
#9391=CARTESIAN_POINT('Ctrl Pts',(-37.276738922573,-30.1603420317173,10.));
#9392=CARTESIAN_POINT('Ctrl Pts',(-37.275992018335,-30.1744798421861,10.));
#9393=CARTESIAN_POINT('Ctrl Pts',(-37.2753552426062,-30.1886265975985,10.));
#9394=CARTESIAN_POINT('Ctrl Pts',(-37.2748295234487,-30.2027664976382,10.));
#9395=CARTESIAN_POINT('Ctrl Pts',(-37.2712907888299,-30.2979453646585,10.));
#9396=CARTESIAN_POINT('Ctrl Pts',(-37.2727707826484,-30.3929751968539,10.));
#9397=CARTESIAN_POINT('Ctrl Pts',(-37.2793281519079,-30.4874572708813,10.));
#9398=CARTESIAN_POINT('Ctrl Pts',(-37.2858630328702,-30.5816153215274,10.));
#9399=CARTESIAN_POINT('Ctrl Pts',(-37.2974401643112,-30.6752303180479,10.));
#9400=CARTESIAN_POINT('Ctrl Pts',(-37.3141655895868,-30.7679255281587,10.));
#9401=CARTESIAN_POINT('Ctrl Pts',(-37.3161024540939,-30.7786599674617,10.));
#9402=CARTESIAN_POINT('Ctrl Pts',(-37.318108416306,-30.7893820824334,10.));
#9403=CARTESIAN_POINT('Ctrl Pts',(-37.3201836861397,-30.8000912944808,10.));
#9404=CARTESIAN_POINT('Ctrl Pts',(-37.3377286165496,-30.8906300654228,10.));
#9405=CARTESIAN_POINT('Ctrl Pts',(-37.3602229262488,-30.9802469068505,10.));
#9406=CARTESIAN_POINT('Ctrl Pts',(-37.3873913235099,-31.0687038922713,10.));
#9407=CARTESIAN_POINT('Ctrl Pts',(-37.3981396071766,-31.1036989919992,10.));
#9408=CARTESIAN_POINT('Ctrl Pts',(-37.4096200259303,-31.1385125085135,10.));
#9409=CARTESIAN_POINT('Ctrl Pts',(-37.4218177279703,-31.1731293672529,10.));
#9410=CARTESIAN_POINT('Ctrl Pts',(-37.4277721424854,-31.1900278884227,10.));
#9411=CARTESIAN_POINT('Ctrl Pts',(-37.4338975028831,-31.2068795420036,10.));
#9412=CARTESIAN_POINT('Ctrl Pts',(-37.4401921825299,-31.2236825462617,10.));
#9413=CARTESIAN_POINT('Ctrl Pts',(-37.4454367253902,-31.2376823176491,10.));
#9414=CARTESIAN_POINT('Ctrl Pts',(-37.4507959097479,-31.251640508919,10.));
#9415=CARTESIAN_POINT('Ctrl Pts',(-37.4562665217367,-31.2655515407123,10.));
#9416=CARTESIAN_POINT('Ctrl Pts',(-37.4904911315776,-31.3525801284799,10.));
#9417=CARTESIAN_POINT('Ctrl Pts',(-37.5290941815582,-31.4378205888918,10.));
#9418=CARTESIAN_POINT('Ctrl Pts',(-37.5717431863619,-31.5210410503347,10.));
#9419=CARTESIAN_POINT('Ctrl Pts',(-37.6159724064538,-31.6073449658009,10.));
#9420=CARTESIAN_POINT('Ctrl Pts',(-37.6645530837038,-31.6914771466329,10.));
#9421=CARTESIAN_POINT('Ctrl Pts',(-37.717170350465,-31.7731754529168,10.));
#9422=CARTESIAN_POINT('Ctrl Pts',(-37.7703652467546,-31.8557706388191,10.));
#9423=CARTESIAN_POINT('Ctrl Pts',(-37.8276862641756,-31.9358790367524,10.));
#9424=CARTESIAN_POINT('Ctrl Pts',(-37.8888596681732,-32.0132144212221,10.));
#9425=CARTESIAN_POINT('Ctrl Pts',(-37.9126768228721,-32.0433240553972,10.));
#9426=CARTESIAN_POINT('Ctrl Pts',(-37.9370784537989,-32.0730131141866,10.));
#9427=CARTESIAN_POINT('Ctrl Pts',(-37.9620502718248,-32.1022636654044,10.));
#9428=CARTESIAN_POINT('Ctrl Pts',(-37.9820385514047,-32.1256767863474,10.));
#9429=CARTESIAN_POINT('Ctrl Pts',(-38.0023921666863,-32.1488089475494,10.));
#9430=CARTESIAN_POINT('Ctrl Pts',(-38.0231042262141,-32.17165061074,10.));
#9431=CARTESIAN_POINT('Ctrl Pts',(-38.0346509963009,-32.1843846139862,10.));
#9432=CARTESIAN_POINT('Ctrl Pts',(-38.0463040959221,-32.1970226665823,10.));
#9433=CARTESIAN_POINT('Ctrl Pts',(-38.0580572806936,-32.2095583549418,10.));
#9434=CARTESIAN_POINT('Ctrl Pts',(-38.1271126580838,-32.2832113015552,10.));
#9435=CARTESIAN_POINT('Ctrl Pts',(-38.1996686238852,-32.3533868119705,10.));
#9436=CARTESIAN_POINT('Ctrl Pts',(-38.2754132400136,-32.4197960351437,10.));
#9437=CARTESIAN_POINT('Ctrl Pts',(-38.3396640840132,-32.476128073727,10.));
#9438=CARTESIAN_POINT('Ctrl Pts',(-38.4062103469001,-32.5297501453147,10.));
#9439=CARTESIAN_POINT('Ctrl Pts',(-38.4748864946038,-32.5804710235722,10.));
#9440=CARTESIAN_POINT('Ctrl Pts',(-38.4975765316306,-32.5972287865536,10.));
#9441=CARTESIAN_POINT('Ctrl Pts',(-38.5204992313683,-32.6136697219234,10.));
#9442=CARTESIAN_POINT('Ctrl Pts',(-38.5436490948133,-32.629786492381,10.));
#9443=CARTESIAN_POINT('Ctrl Pts',(-38.5602427937514,-32.6413389076885,10.));
#9444=CARTESIAN_POINT('Ctrl Pts',(-38.5769541763244,-32.652725292037,10.));
#9445=CARTESIAN_POINT('Ctrl Pts',(-38.5937666592579,-32.6639334564857,10.));
#9446=CARTESIAN_POINT('Ctrl Pts',(-38.6801204794835,-32.721501860967,10.));
#9447=CARTESIAN_POINT('Ctrl Pts',(-38.7692236934361,-32.774432012051,10.));
#9448=CARTESIAN_POINT('Ctrl Pts',(-38.860767757559,-32.822402446742,10.));
#9449=CARTESIAN_POINT('Ctrl Pts',(-38.9523118216819,-32.8703728814329,10.));
#9450=CARTESIAN_POINT('Ctrl Pts',(-39.0462973813034,-32.9133845104196,10.));
#9451=CARTESIAN_POINT('Ctrl Pts',(-39.1424539364134,-32.951075124157,10.));
#9452=CARTESIAN_POINT('Ctrl Pts',(-39.1630219002104,-32.9591371764835,10.));
#9453=CARTESIAN_POINT('Ctrl Pts',(-39.1836893128189,-32.9669555963369,10.));
#9454=CARTESIAN_POINT('Ctrl Pts',(-39.2044522699742,-32.9745315604842,10.));
#9455=CARTESIAN_POINT('Ctrl Pts',(-42.51946795121,-30.0019779683886,8.38741669750802));
#9456=CARTESIAN_POINT('Ctrl Pts',(-42.5205894505478,-30.1321096272865,8.3956620675864));
#9457=CARTESIAN_POINT('Ctrl Pts',(-42.5113779533637,-30.2620820270818,8.40390743766478));
#9458=CARTESIAN_POINT('Ctrl Pts',(-42.4912804519573,-30.3903486209662,8.41215280774316));
#9459=CARTESIAN_POINT('Ctrl Pts',(-42.3622716430691,-31.213710697799,8.46508104748505));
#9460=CARTESIAN_POINT('Ctrl Pts',(-41.7847001994946,-31.9667842851201,8.51800928722694));
#9461=CARTESIAN_POINT('Ctrl Pts',(-41.0229436930189,-32.3048687922893,8.57093752696884));
#9462=CARTESIAN_POINT('Ctrl Pts',(-40.2611871865431,-32.6429532994586,8.62386576671073));
#9463=CARTESIAN_POINT('Ctrl Pts',(-39.3152456171661,-32.566048726476,8.67679400645262));
#9464=CARTESIAN_POINT('Ctrl Pts',(-38.6181178943748,-32.1093322946775,8.72972224619452));
#9465=CARTESIAN_POINT('Ctrl Pts',(-37.9209901715836,-31.652615862879,8.78265048593641));
#9466=CARTESIAN_POINT('Ctrl Pts',(-37.472676295378,-30.8160875722647,8.83557872567831));
#9467=CARTESIAN_POINT('Ctrl Pts',(-37.4783843069573,-29.9827116901432,8.8885069654202));
#9468=CARTESIAN_POINT('Ctrl Pts',(-37.4840923185365,-29.1493358080216,8.9414352051621));
#9469=CARTESIAN_POINT('Ctrl Pts',(-37.9438222179007,-28.3191123343929,8.994363444904));
#9470=CARTESIAN_POINT('Ctrl Pts',(-38.6471442946355,-27.8719686461583,9.04729168464589));
#9471=CARTESIAN_POINT('Ctrl Pts',(-39.3504663713704,-27.4248249579237,9.10021992438779));
#9472=CARTESIAN_POINT('Ctrl Pts',(-40.297380625476,-27.3607610550832,9.15314816412968));
#9473=CARTESIAN_POINT('Ctrl Pts',(-41.0544291986404,-27.7093025098685,9.20607640387157));
#9474=CARTESIAN_POINT('Ctrl Pts',(-41.8114777718049,-28.0578439646537,9.25900464361346));
#9475=CARTESIAN_POINT('Ctrl Pts',(-42.3786606640282,-28.8189907770648,9.31193288335536));
#9476=CARTESIAN_POINT('Ctrl Pts',(-42.4963858324552,-29.6439329582262,9.36486112309726));
#9477=CARTESIAN_POINT('Ctrl Pts',(-42.5131088446533,-29.7611170603394,9.37237964790084));
#9478=CARTESIAN_POINT('Ctrl Pts',(-42.5207624429925,-29.8795884617265,9.37989817270443));
#9479=CARTESIAN_POINT('Ctrl Pts',(-42.5197817068771,-29.9981833838556,9.38741669750801));
#9480=CARTESIAN_POINT('Ctrl Pts',(-40.7937992825329,-32.9692229537457,10.));
#9481=CARTESIAN_POINT('Ctrl Pts',(-41.7812379463276,-32.7052387009375,9.94707176025811));
#9482=CARTESIAN_POINT('Ctrl Pts',(-43.4548293913714,-31.1184189156626,9.84121528077431));
#9483=CARTESIAN_POINT('Ctrl Pts',(-42.8129704324572,-27.6976302329706,9.68243056154864));
#9484=CARTESIAN_POINT('Ctrl Pts',(-39.5908856218057,-26.3909740388041,9.52364584232295));
#9485=CARTESIAN_POINT('Ctrl Pts',(-36.745809981275,-28.3852514028181,9.36486112309727));
#9486=CARTESIAN_POINT('Ctrl Pts',(-36.8786561820279,-31.8593324073604,9.20607640387158));
#9487=CARTESIAN_POINT('Ctrl Pts',(-39.869659454766,-33.6304609478428,9.0472916846459));
#9488=CARTESIAN_POINT('Ctrl Pts',(-42.9796777427015,-32.0783451207568,8.88850696542022));
#9489=CARTESIAN_POINT('Ctrl Pts',(-43.3620052935445,-28.6233470774409,8.72972224619453));
#9490=CARTESIAN_POINT('Ctrl Pts',(-40.6663949208769,-26.4287479717036,8.57093752696886));
#9491=CARTESIAN_POINT('Ctrl Pts',(-37.3607498677919,-27.5035230729969,8.41215280774315));
#9492=CARTESIAN_POINT('Ctrl Pts',(-36.4712752548112,-30.8638056099088,8.25336808851749));
#9493=CARTESIAN_POINT('Ctrl Pts',(-38.8122995967417,-33.4332763392514,8.0945833692918));
#9494=CARTESIAN_POINT('Ctrl Pts',(-42.2406391600676,-32.8596453238364,7.93579865006611));
#9495=CARTESIAN_POINT('Ctrl Pts',(-43.6177130282472,-29.6680532348257,7.77701393084043));
#9496=CARTESIAN_POINT('Ctrl Pts',(-41.6828291578641,-26.7803544372571,7.61822921161475));
#9497=CARTESIAN_POINT('Ctrl Pts',(-38.2073436047123,-26.8401872096979,7.45944449238906));
#9498=CARTESIAN_POINT('Ctrl Pts',(-36.3730050616526,-29.7927767730296,7.30065977316338));
#9499=CARTESIAN_POINT('Ctrl Pts',(-37.8591206231434,-32.9350755877781,7.1418750539377));
#9500=CARTESIAN_POINT('Ctrl Pts',(-41.3051758117063,-33.390361281965,6.98309033471201));
#9501=CARTESIAN_POINT('Ctrl Pts',(-43.5563641435752,-30.7418271809609,6.82430561548632));
#9502=CARTESIAN_POINT('Ctrl Pts',(-42.5517598309746,-27.4141625739817,6.66552089626065));
#9503=CARTESIAN_POINT('Ctrl Pts',(-39.2110615557591,-26.4537894026696,6.50673617703496));
#9504=CARTESIAN_POINT('Ctrl Pts',(-36.592623388795,-28.7399134586708,6.34795145780928));
#9505=CARTESIAN_POINT('Ctrl Pts',(-37.0935822247194,-32.1796259246658,6.18916673858359));
#9506=CARTESIAN_POINT('Ctrl Pts',(-40.2553185210464,-33.623926863772,6.03038201935791));
#9507=CARTESIAN_POINT('Ctrl Pts',(-43.1833149296159,-31.7505826226676,5.87159730013223));
#9508=CARTESIAN_POINT('Ctrl Pts',(-43.1970391055899,-28.2746089090863,5.71281258090654));
#9509=CARTESIAN_POINT('Ctrl Pts',(-40.2839267930322,-26.378202236992,5.55402786168086));
#9510=CARTESIAN_POINT('Ctrl Pts',(-37.1108841916168,-27.7974915878749,5.39524314245518));
#9511=CARTESIAN_POINT('Ctrl Pts',(-36.5827793869729,-31.2331410063646,5.23645842322949));
#9512=CARTESIAN_POINT('Ctrl Pts',(-39.1830836038332,-33.5398702040376,5.07767370400381));
#9513=CARTESIAN_POINT('Ctrl Pts',(-42.5312612865998,-32.605906705675,4.91888898477813));
#9514=CARTESIAN_POINT('Ctrl Pts',(-43.5621110758558,-29.2862786657343,4.76010426555244));
#9515=CARTESIAN_POINT('Ctrl Pts',(-41.3319070183432,-26.6200507172078,4.60131954632676));
#9516=CARTESIAN_POINT('Ctrl Pts',(-37.8823640875572,-27.0481105030832,4.44253482710108));
#9517=CARTESIAN_POINT('Ctrl Pts',(-36.3714818529893,-30.1785763605433,4.28375010787539));
#9518=CARTESIAN_POINT('Ctrl Pts',(-38.1824480418478,-33.1455585099229,4.12496538864971));
#9519=CARTESIAN_POINT('Ctrl Pts',(-41.6573530239065,-33.2328338054134,3.96618066942403));
#9520=CARTESIAN_POINT('Ctrl Pts',(-43.6149786907205,-30.3605031560721,3.80739595019834));
#9521=CARTESIAN_POINT('Ctrl Pts',(-42.2631510826477,-27.1581378220842,3.64861123097266));
#9522=CARTESIAN_POINT('Ctrl Pts',(-38.8394460438999,-26.5574503676893,3.48982651174697));
#9523=CARTESIAN_POINT('Ctrl Pts',(-36.4782089804049,-29.1083602316377,3.33104179252129));
#9524=CARTESIAN_POINT('Ctrl Pts',(-37.341113418528,-32.4755515781919,3.17225707329561));
#9525=CARTESIAN_POINT('Ctrl Pts',(-40.6381845987477,-33.5764163413526,3.01347235406993));
#9526=CARTESIAN_POINT('Ctrl Pts',(-43.3510083223003,-31.4031310387823,2.85468763484424));
#9527=CARTESIAN_POINT('Ctrl Pts',(-42.9960392803275,-27.945302418251,2.69590291561856));
#9528=CARTESIAN_POINT('Ctrl Pts',(-39.898245774117,-26.3685155528715,2.53711819639287));
#9529=CARTESIAN_POINT('Ctrl Pts',(-36.8936065712748,-28.1162925878559,2.37833347716719));
#9530=CARTESIAN_POINT('Ctrl Pts',(-36.7328192563745,-31.5885728846373,2.2195487579415));
#9531=CARTESIAN_POINT('Ctrl Pts',(-39.5630819030797,-33.6065404615547,2.06076403871582));
#9532=CARTESIAN_POINT('Ctrl Pts',(-42.7933359259129,-32.3227807935024,1.90197931949014));
#9533=CARTESIAN_POINT('Ctrl Pts',(-43.4663369005618,-28.912551741198,1.74319460026445));
#9534=CARTESIAN_POINT('Ctrl Pts',(-40.9659640066834,-26.4978674771854,1.58440988103877));
#9535=CARTESIAN_POINT('Ctrl Pts',(-37.5812664167199,-27.2893199539358,1.42562516181309));
#9536=CARTESIAN_POINT('Ctrl Pts',(-36.410880674872,-30.5623706761659,1.26684044258741));
#9537=CARTESIAN_POINT('Ctrl Pts',(-38.5262719729362,-33.320549494049,1.10805572336172));
#9538=CARTESIAN_POINT('Ctrl Pts',(-41.9908417541182,-33.0388816977749,0.949271004136036));
#9539=CARTESIAN_POINT('Ctrl Pts',(-43.6328191716239,-29.9750448881763,0.790486284910355));
#9540=CARTESIAN_POINT('Ctrl Pts',(-41.9490298715236,-26.9342997681684,0.631701565684669));
#9541=CARTESIAN_POINT('Ctrl Pts',(-38.4808975311013,-26.6996618476225,0.472916846458986));
#9542=CARTESIAN_POINT('Ctrl Pts',(-36.4035550403569,-29.4874091667537,0.314132127233303));
#9543=CARTESIAN_POINT('Ctrl Pts',(-37.6185459416804,-32.7424659580649,0.155347408007618));
#9544=CARTESIAN_POINT('Ctrl Pts',(-41.0140166119162,-33.4907706181827,-0.00343731121806399));
#9545=CARTESIAN_POINT('Ctrl Pts',(-43.4806505248308,-31.0352675588419,-0.162222030443749));
#9546=CARTESIAN_POINT('Ctrl Pts',(-43.0002811455947,-28.7795746242083,-0.268078509927538));
#9547=CARTESIAN_POINT('Ctrl Pts',(-42.3360626576962,-28.0026984430693,-0.321006749669432));
#9548=CARTESIAN_POINT('Ctrl Pts',(-40.745932854347,-32.7901775698422,10.1070022498898));
#9549=CARTESIAN_POINT('Ctrl Pts',(-41.673828554412,-32.5421116777044,10.0540740101479));
#9550=CARTESIAN_POINT('Ctrl Pts',(-43.2465017365151,-31.0509777880547,9.94821753066413));
#9551=CARTESIAN_POINT('Ctrl Pts',(-42.6433471408303,-27.836464091272,9.78943281143844));
#9552=CARTESIAN_POINT('Ctrl Pts',(-39.6155553896356,-26.6085998112053,9.63064809221276));
#9553=CARTESIAN_POINT('Ctrl Pts',(-36.9420389981841,-28.482621417463,9.47186337298707));
#9554=CARTESIAN_POINT('Ctrl Pts',(-37.0668745175621,-31.7472138868363,9.31307865376139));
#9555=CARTESIAN_POINT('Ctrl Pts',(-39.877519044067,-33.4115426367967,9.1542939345357));
#9556=CARTESIAN_POINT('Ctrl Pts',(-42.8000019306586,-31.9530200421666,8.99550921531003));
#9557=CARTESIAN_POINT('Ctrl Pts',(-43.1592749705456,-28.7063598234897,8.83672449608434));
#9558=CARTESIAN_POINT('Ctrl Pts',(-40.6262110288963,-26.6440959601784,8.67793977685866));
#9559=CARTESIAN_POINT('Ctrl Pts',(-37.5198977527772,-27.6540616740938,8.51915505763297));
#9560=CARTESIAN_POINT('Ctrl Pts',(-36.6840588303576,-30.8117177709512,8.3603703384073));
#9561=CARTESIAN_POINT('Ctrl Pts',(-38.8839184269799,-33.2262483424373,8.2015856191816));
#9562=CARTESIAN_POINT('Ctrl Pts',(-42.1055276831414,-32.6872075167703,8.04280089995592));
#9563=CARTESIAN_POINT('Ctrl Pts',(-43.3995634220756,-29.6880697633694,7.88401618073025));
#9564=CARTESIAN_POINT('Ctrl Pts',(-41.5813538569833,-26.9745004090466,7.72523146150455));
#9565=CARTESIAN_POINT('Ctrl Pts',(-38.315441533868,-27.0307252403262,7.56644674227887));
#9566=CARTESIAN_POINT('Ctrl Pts',(-36.5917143708789,-29.8052724201415,7.40766202305319));
#9567=CARTESIAN_POINT('Ctrl Pts',(-37.9882165434875,-32.7580893043005,7.24887730382751));
#9568=CARTESIAN_POINT('Ctrl Pts',(-41.226473165287,-33.1859210810244,7.09009258460182));
#9569=CARTESIAN_POINT('Ctrl Pts',(-43.3419139007655,-30.6970946922006,6.93130786537613));
#9570=CARTESIAN_POINT('Ctrl Pts',(-42.397887647685,-27.5700896504815,6.77252314615046));
#9571=CARTESIAN_POINT('Ctrl Pts',(-39.2586348733664,-26.6676273824012,6.61373842692477));
#9572=CARTESIAN_POINT('Ctrl Pts',(-36.7980896211934,-28.8158972032594,6.45495370769909));
#9573=CARTESIAN_POINT('Ctrl Pts',(-37.2688404301373,-32.0481935713103,6.2961689884734));
#9574=CARTESIAN_POINT('Ctrl Pts',(-40.2399227076196,-33.4054025607237,6.13738426924772));
#9575=CARTESIAN_POINT('Ctrl Pts',(-42.9913597101737,-31.6450217595687,5.97859955002204));
#9576=CARTESIAN_POINT('Ctrl Pts',(-43.004256312606,-28.3786507123017,5.81981483079635));
#9577=CARTESIAN_POINT('Ctrl Pts',(-40.2668058888593,-26.5965981543753,5.66103011157067));
#9578=CARTESIAN_POINT('Ctrl Pts',(-37.2850990812065,-27.9303037647787,5.50224539234499));
#9579=CARTESIAN_POINT('Ctrl Pts',(-36.7888392167916,-31.1587820887854,5.3434606731193));
#9580=CARTESIAN_POINT('Ctrl Pts',(-39.2323440036238,-33.326414552669,5.18467595389362));
#9581=CARTESIAN_POINT('Ctrl Pts',(-42.378625174095,-32.448769443232,5.02589123466794));
#9582=CARTESIAN_POINT('Ctrl Pts',(-43.3473142906298,-29.3293163602033,4.86710651544225));
#9583=CARTESIAN_POINT('Ctrl Pts',(-41.2515924690022,-26.8238630702507,4.70832179621657));
#9584=CARTESIAN_POINT('Ctrl Pts',(-38.0100584172918,-27.2261106723024,4.54953707699089));
#9585=CARTESIAN_POINT('Ctrl Pts',(-36.590283012334,-30.1678081314383,4.39075235776521));
#9586=CARTESIAN_POINT('Ctrl Pts',(-38.2920471838393,-32.9558800183533,4.23196763853952));
#9587=CARTESIAN_POINT('Ctrl Pts',(-41.5574139445407,-33.0378925770842,4.07318291931383));
#9588=CARTESIAN_POINT('Ctrl Pts',(-43.3969939662434,-30.3387646652336,3.91439820008815));
#9589=CARTESIAN_POINT('Ctrl Pts',(-42.1266821273902,-27.329503298026,3.75561348086246));
#9590=CARTESIAN_POINT('Ctrl Pts',(-38.9094279320396,-26.7650375479468,3.59682876163679));
#9591=CARTESIAN_POINT('Ctrl Pts',(-36.6905744494028,-29.1621264819722,3.4380440424111));
#9592=CARTESIAN_POINT('Ctrl Pts',(-37.5014453896032,-32.3262747843657,3.27925932318542));
#9593=CARTESIAN_POINT('Ctrl Pts',(-40.5997018009706,-33.360756942644,3.12047460395974));
#9594=CARTESIAN_POINT('Ctrl Pts',(-43.1489411212593,-31.3185216512694,2.96168988473405));
#9595=CARTESIAN_POINT('Ctrl Pts',(-42.815376860734,-28.0692015403651,2.80290516550837));
#9596=CARTESIAN_POINT('Ctrl Pts',(-39.9043815964251,-26.5874955813519,2.64412044628268));
#9597=CARTESIAN_POINT('Ctrl Pts',(-37.0809233920948,-28.2298809313462,2.485335727057));
#9598=CARTESIAN_POINT('Ctrl Pts',(-36.9298316194194,-31.4927812763885,2.32655100783131));
#9599=CARTESIAN_POINT('Ctrl Pts',(-39.5894282467582,-33.3890645658197,2.16776628860563));
#9600=CARTESIAN_POINT('Ctrl Pts',(-42.624896603229,-32.1827161417821,2.00898156937995));
#9601=CARTESIAN_POINT('Ctrl Pts',(-43.2573153380963,-28.9781253252655,1.85019685015427));
#9602=CARTESIAN_POINT('Ctrl Pts',(-40.9077159737442,-26.7090475306191,1.69141213092858));
#9603=CARTESIAN_POINT('Ctrl Pts',(-37.7271170617287,-27.4527750925521,1.5326274117029));
#9604=CARTESIAN_POINT('Ctrl Pts',(-36.6273060688062,-30.5284594895764,1.37384269247722));
#9605=CARTESIAN_POINT('Ctrl Pts',(-38.6151383883202,-33.1203189730695,1.21505797325153));
#9606=CARTESIAN_POINT('Ctrl Pts',(-41.8707931650731,-32.8556358625206,1.05627325402585));
#9607=CARTESIAN_POINT('Ctrl Pts',(-43.4137586586991,-29.9765496918393,0.897488534800165));
#9608=CARTESIAN_POINT('Ctrl Pts',(-41.8315025564575,-27.1191627722244,0.73870381557448));
#9609=CARTESIAN_POINT('Ctrl Pts',(-38.5725000442738,-26.8986736162599,0.579919096348797));
#9610=CARTESIAN_POINT('Ctrl Pts',(-36.6204221731113,-29.5183186080297,0.421134377123114));
#9611=CARTESIAN_POINT('Ctrl Pts',(-37.7621486157681,-32.5770941156828,0.262349657897428));
#9612=CARTESIAN_POINT('Ctrl Pts',(-40.9528709868172,-33.2802756923425,0.103564938671747));
#9613=CARTESIAN_POINT('Ctrl Pts',(-43.2707658448453,-30.97284049277,-0.0552197805539385));
#9614=CARTESIAN_POINT('Ctrl Pts',(-42.8193629397544,-28.8531667839546,-0.161076260037727));
#9615=CARTESIAN_POINT('Ctrl Pts',(-42.1951971040191,-28.1231365609212,-0.214004499779622));
#9616=CARTESIAN_POINT('Ctrl Pts',(-40.698066426161,-32.6111321859386,10.2140044997796));
#9617=CARTESIAN_POINT('Ctrl Pts',(-41.5664191624963,-32.3789846544712,10.1610762600377));
#9618=CARTESIAN_POINT('Ctrl Pts',(-43.0381740816587,-30.9835366604468,10.0552197805539));
#9619=CARTESIAN_POINT('Ctrl Pts',(-42.4737238492034,-27.9752979495734,9.89643506132826));
#9620=CARTESIAN_POINT('Ctrl Pts',(-39.6402251574656,-26.8262255836064,9.73765034210257));
#9621=CARTESIAN_POINT('Ctrl Pts',(-37.1382680150933,-28.5799914321079,9.57886562287689));
#9622=CARTESIAN_POINT('Ctrl Pts',(-37.2550928530962,-31.6350953663122,9.4200809036512));
#9623=CARTESIAN_POINT('Ctrl Pts',(-39.8853786333681,-33.1926243257506,9.26129618442552));
#9624=CARTESIAN_POINT('Ctrl Pts',(-42.6203261186156,-31.8276949635764,9.10251146519983));
#9625=CARTESIAN_POINT('Ctrl Pts',(-42.9565446475468,-28.7893725695385,8.94372674597416));
#9626=CARTESIAN_POINT('Ctrl Pts',(-40.5860271369156,-26.8594439486533,8.78494202674846));
#9627=CARTESIAN_POINT('Ctrl Pts',(-37.6790456377626,-27.8046002751907,8.62615730752279));
#9628=CARTESIAN_POINT('Ctrl Pts',(-36.8968424059039,-30.7596299319935,8.4673725882971));
#9629=CARTESIAN_POINT('Ctrl Pts',(-38.9555372572181,-33.0192203456233,8.30858786907142));
#9630=CARTESIAN_POINT('Ctrl Pts',(-41.9704162062153,-32.5147697097042,8.14980314984574));
#9631=CARTESIAN_POINT('Ctrl Pts',(-43.181413815904,-29.7080862919131,7.99101843062005));
#9632=CARTESIAN_POINT('Ctrl Pts',(-41.4798785561023,-27.1686463808361,7.83223371139437));
#9633=CARTESIAN_POINT('Ctrl Pts',(-38.4235394630237,-27.2212632709545,7.67344899216868));
#9634=CARTESIAN_POINT('Ctrl Pts',(-36.8104236801052,-29.8177680672534,7.51466427294301));
#9635=CARTESIAN_POINT('Ctrl Pts',(-38.1173124638315,-32.5811030208231,7.35587955371732));
#9636=CARTESIAN_POINT('Ctrl Pts',(-41.1477705188678,-32.9814808800838,7.19709483449163));
#9637=CARTESIAN_POINT('Ctrl Pts',(-43.1274636579556,-30.6523622034403,7.03831011526595));
#9638=CARTESIAN_POINT('Ctrl Pts',(-42.2440154643954,-27.7260167269812,6.87952539604026));
#9639=CARTESIAN_POINT('Ctrl Pts',(-39.3062081909736,-26.8814653621329,6.72074067681458));
#9640=CARTESIAN_POINT('Ctrl Pts',(-37.0035558535919,-28.891880947848,6.5619559575889));
#9641=CARTESIAN_POINT('Ctrl Pts',(-37.4440986355553,-31.9167612179548,6.40317123836321));
#9642=CARTESIAN_POINT('Ctrl Pts',(-40.2245268941928,-33.1868782576754,6.24438651913754));
#9643=CARTESIAN_POINT('Ctrl Pts',(-42.7994044907315,-31.5394608964698,6.08560179991185));
#9644=CARTESIAN_POINT('Ctrl Pts',(-42.8114735196222,-28.4826925155172,5.92681708068617));
#9645=CARTESIAN_POINT('Ctrl Pts',(-40.2496849846864,-26.8149940717586,5.76803236146048));
#9646=CARTESIAN_POINT('Ctrl Pts',(-37.4593139707961,-28.0631159416825,5.6092476422348));
#9647=CARTESIAN_POINT('Ctrl Pts',(-36.9948990466102,-31.0844231712062,5.45046292300912));
#9648=CARTESIAN_POINT('Ctrl Pts',(-39.2816044034143,-33.1129589013003,5.29167820378343));
#9649=CARTESIAN_POINT('Ctrl Pts',(-42.2259890615903,-32.2916321807891,5.13289348455775));
#9650=CARTESIAN_POINT('Ctrl Pts',(-43.1325175054039,-29.3723540546723,4.97410876533206));
#9651=CARTESIAN_POINT('Ctrl Pts',(-41.1712779196612,-27.0276754232936,4.81532404610638));
#9652=CARTESIAN_POINT('Ctrl Pts',(-38.1377527470264,-27.4041108415216,4.6565393268807));
#9653=CARTESIAN_POINT('Ctrl Pts',(-36.8090841716787,-30.1570399023334,4.49775460765501));
#9654=CARTESIAN_POINT('Ctrl Pts',(-38.4016463258308,-32.7662015267838,4.33896988842933));
#9655=CARTESIAN_POINT('Ctrl Pts',(-41.457474865175,-32.8429513487549,4.18018516920364));
#9656=CARTESIAN_POINT('Ctrl Pts',(-43.1790092417664,-30.3170261743952,4.02140044997796));
#9657=CARTESIAN_POINT('Ctrl Pts',(-41.9902131721327,-27.5008687739677,3.86261573075228));
#9658=CARTESIAN_POINT('Ctrl Pts',(-38.9794098201792,-26.9726247282044,3.70383101152659));
#9659=CARTESIAN_POINT('Ctrl Pts',(-36.9029399184007,-29.2158927323067,3.54504629230091));
#9660=CARTESIAN_POINT('Ctrl Pts',(-37.6617773606783,-32.1769979905394,3.38626157307523));
#9661=CARTESIAN_POINT('Ctrl Pts',(-40.5612190031936,-33.1450975439355,3.22747685384954));
#9662=CARTESIAN_POINT('Ctrl Pts',(-42.9468739202182,-31.2339122637565,3.06869213462387));
#9663=CARTESIAN_POINT('Ctrl Pts',(-42.6347144411405,-28.1931006624791,2.90990741539817));
#9664=CARTESIAN_POINT('Ctrl Pts',(-39.9105174187331,-26.8064756098323,2.7511226961725));
#9665=CARTESIAN_POINT('Ctrl Pts',(-37.2682402129149,-28.3434692748364,2.59233797694681));
#9666=CARTESIAN_POINT('Ctrl Pts',(-37.1268439824643,-31.3969896681396,2.43355325772113));
#9667=CARTESIAN_POINT('Ctrl Pts',(-39.6157745904367,-33.1715886700848,2.27476853849544));
#9668=CARTESIAN_POINT('Ctrl Pts',(-42.456457280545,-32.0426514900617,2.11598381926976));
#9669=CARTESIAN_POINT('Ctrl Pts',(-43.048293775631,-29.0436989093329,1.95719910004408));
#9670=CARTESIAN_POINT('Ctrl Pts',(-40.8494679408049,-26.9202275840527,1.79841438081839));
#9671=CARTESIAN_POINT('Ctrl Pts',(-37.8729677067375,-27.6162302311684,1.63962966159271));
#9672=CARTESIAN_POINT('Ctrl Pts',(-36.8437314627405,-30.494548302987,1.48084494236703));
#9673=CARTESIAN_POINT('Ctrl Pts',(-38.7040048037041,-32.92008845209,1.32206022314134));
#9674=CARTESIAN_POINT('Ctrl Pts',(-41.7507445760281,-32.6723900272662,1.16327550391566));
#9675=CARTESIAN_POINT('Ctrl Pts',(-43.1946981457743,-29.9780544955022,1.00449078468998));
#9676=CARTESIAN_POINT('Ctrl Pts',(-41.7139752413914,-27.3040257762804,0.845706065464291));
#9677=CARTESIAN_POINT('Ctrl Pts',(-38.6641025574464,-27.0976853848974,0.686921346238608));
#9678=CARTESIAN_POINT('Ctrl Pts',(-36.8372893058656,-29.5492280493056,0.528136627012925));
#9679=CARTESIAN_POINT('Ctrl Pts',(-37.9057512898559,-32.4117222733007,0.369351907787239));
#9680=CARTESIAN_POINT('Ctrl Pts',(-40.8917253617181,-33.0697807665023,0.210567188561557));
#9681=CARTESIAN_POINT('Ctrl Pts',(-43.0608811648599,-30.9104134266981,0.0517824693358723));
#9682=CARTESIAN_POINT('Ctrl Pts',(-42.6384447339141,-28.9267589437008,-0.0540740101479163));
#9683=CARTESIAN_POINT('Ctrl Pts',(-42.0543315503421,-28.2435746787731,-0.107002249889811));
#9684=CARTESIAN_POINT('Ctrl Pts',(-40.6501999979751,-32.4320868020351,10.3210067496694));
#9685=CARTESIAN_POINT('Ctrl Pts',(-41.4590097705807,-32.2158576312381,10.2680785099275));
#9686=CARTESIAN_POINT('Ctrl Pts',(-42.8298464268025,-30.916095532839,10.1622220304438));
#9687=CARTESIAN_POINT('Ctrl Pts',(-42.3041005575764,-28.1141318078749,10.0034373112181));
#9688=CARTESIAN_POINT('Ctrl Pts',(-39.6648949252955,-27.0438513560076,9.84465259199239));
#9689=CARTESIAN_POINT('Ctrl Pts',(-37.3344970320025,-28.6773614467528,9.68586787276669));
#9690=CARTESIAN_POINT('Ctrl Pts',(-37.4433111886304,-31.5229768457881,9.52708315354102));
#9691=CARTESIAN_POINT('Ctrl Pts',(-39.8932382226691,-32.9737060147045,9.36829843431533));
#9692=CARTESIAN_POINT('Ctrl Pts',(-42.4406503065726,-31.7023698849862,9.20951371508964));
#9693=CARTESIAN_POINT('Ctrl Pts',(-42.753814324548,-28.8723853155873,9.05072899586397));
#9694=CARTESIAN_POINT('Ctrl Pts',(-40.545843244935,-27.0747919371282,8.89194427663828));
#9695=CARTESIAN_POINT('Ctrl Pts',(-37.838193522748,-27.9551388762876,8.7331595574126));
#9696=CARTESIAN_POINT('Ctrl Pts',(-37.1096259814502,-30.7075420930358,8.57437483818691));
#9697=CARTESIAN_POINT('Ctrl Pts',(-39.0271560874564,-32.8121923488093,8.41559011896123));
#9698=CARTESIAN_POINT('Ctrl Pts',(-41.8353047292891,-32.3423319026381,8.25680539973555));
#9699=CARTESIAN_POINT('Ctrl Pts',(-42.9632642097323,-29.7281028204567,8.09802068050986));
#9700=CARTESIAN_POINT('Ctrl Pts',(-41.3784032552214,-27.3627923526256,7.93923596128418));
#9701=CARTESIAN_POINT('Ctrl Pts',(-38.5316373921794,-27.4118013015827,7.78045124205849));
#9702=CARTESIAN_POINT('Ctrl Pts',(-37.0291329893315,-29.8302637143654,7.62166652283281));
#9703=CARTESIAN_POINT('Ctrl Pts',(-38.2464083841756,-32.4041167373455,7.46288180360713));
#9704=CARTESIAN_POINT('Ctrl Pts',(-41.0690678724485,-32.7770406791433,7.30409708438144));
#9705=CARTESIAN_POINT('Ctrl Pts',(-42.9130134151458,-30.60762971468,7.14531236515577));
#9706=CARTESIAN_POINT('Ctrl Pts',(-42.0901432811058,-27.8819438034811,6.98652764593007));
#9707=CARTESIAN_POINT('Ctrl Pts',(-39.353781508581,-27.0953033418645,6.8277429267044));
#9708=CARTESIAN_POINT('Ctrl Pts',(-37.2090220859903,-28.9678646924366,6.66895820747871));
#9709=CARTESIAN_POINT('Ctrl Pts',(-37.6193568409732,-31.7853288645994,6.51017348825303));
#9710=CARTESIAN_POINT('Ctrl Pts',(-40.209131080766,-32.968353954627,6.35138876902734));
#9711=CARTESIAN_POINT('Ctrl Pts',(-42.6074492712894,-31.433900033371,6.19260404980166));
#9712=CARTESIAN_POINT('Ctrl Pts',(-42.6186907266382,-28.5867343187326,6.03381933057598));
#9713=CARTESIAN_POINT('Ctrl Pts',(-40.2325640805136,-27.0333899891419,5.87503461135029));
#9714=CARTESIAN_POINT('Ctrl Pts',(-37.6335288603857,-28.1959281185863,5.71624989212461));
#9715=CARTESIAN_POINT('Ctrl Pts',(-37.2009588764289,-31.0100642536271,5.55746517289893));
#9716=CARTESIAN_POINT('Ctrl Pts',(-39.3308648032049,-32.8995032499315,5.39868045367324));
#9717=CARTESIAN_POINT('Ctrl Pts',(-42.0733529490857,-32.1344949183462,5.23989573444756));
#9718=CARTESIAN_POINT('Ctrl Pts',(-42.917720720178,-29.4153917491414,5.08111101522188));
#9719=CARTESIAN_POINT('Ctrl Pts',(-41.0909633703201,-27.2314877763366,4.92232629599619));
#9720=CARTESIAN_POINT('Ctrl Pts',(-38.2654470767611,-27.5821110107408,4.76354157677051));
#9721=CARTESIAN_POINT('Ctrl Pts',(-37.0278853310234,-30.1462716732285,4.60475685754483));
#9722=CARTESIAN_POINT('Ctrl Pts',(-38.5112454678223,-32.5765230352142,4.44597213831914));
#9723=CARTESIAN_POINT('Ctrl Pts',(-41.3575357858092,-32.6480101204257,4.28718741909346));
#9724=CARTESIAN_POINT('Ctrl Pts',(-42.9610245172894,-30.2952876835567,4.12840269986777));
#9725=CARTESIAN_POINT('Ctrl Pts',(-41.8537442168751,-27.6722342499095,3.96961798064209));
#9726=CARTESIAN_POINT('Ctrl Pts',(-39.0493917083189,-27.1802119084619,3.81083326141641));
#9727=CARTESIAN_POINT('Ctrl Pts',(-37.1153053873985,-29.2696589826413,3.65204854219072));
#9728=CARTESIAN_POINT('Ctrl Pts',(-37.8221093317535,-32.0277211967132,3.49326382296504));
#9729=CARTESIAN_POINT('Ctrl Pts',(-40.5227362054164,-32.929438145227,3.33447910373936));
#9730=CARTESIAN_POINT('Ctrl Pts',(-42.7448067191771,-31.1493028762435,3.17569438451367));
#9731=CARTESIAN_POINT('Ctrl Pts',(-42.454052021547,-28.3169997845931,3.01690966528799));
#9732=CARTESIAN_POINT('Ctrl Pts',(-39.916653241041,-27.0254556383127,2.8581249460623));
#9733=CARTESIAN_POINT('Ctrl Pts',(-37.4555570337349,-28.4570576183267,2.69934022683662));
#9734=CARTESIAN_POINT('Ctrl Pts',(-37.3238563455092,-31.3011980598908,2.54055550761094));
#9735=CARTESIAN_POINT('Ctrl Pts',(-39.6421209341153,-32.9541127743498,2.38177078838525));
#9736=CARTESIAN_POINT('Ctrl Pts',(-42.288017957861,-31.9025868383414,2.22298606915957));
#9737=CARTESIAN_POINT('Ctrl Pts',(-42.8392722131655,-29.1092724934004,2.06420134993389));
#9738=CARTESIAN_POINT('Ctrl Pts',(-40.7912199078658,-27.1314076374864,1.9054166307082));
#9739=CARTESIAN_POINT('Ctrl Pts',(-38.0188183517463,-27.7796853697847,1.74663191148252));
#9740=CARTESIAN_POINT('Ctrl Pts',(-37.0601568566748,-30.4606371163975,1.58784719225684));
#9741=CARTESIAN_POINT('Ctrl Pts',(-38.792871219088,-32.7198579311106,1.42906247303115));
#9742=CARTESIAN_POINT('Ctrl Pts',(-41.6306959869831,-32.4891441920118,1.27027775380547));
#9743=CARTESIAN_POINT('Ctrl Pts',(-42.9756376328495,-29.9795592991651,1.11149303457979));
#9744=CARTESIAN_POINT('Ctrl Pts',(-41.5964479263253,-27.4888887803364,0.952708315354102));
#9745=CARTESIAN_POINT('Ctrl Pts',(-38.755705070619,-27.2966971535349,0.793923596128418));
#9746=CARTESIAN_POINT('Ctrl Pts',(-37.05415643862,-29.5801374905816,0.635138876902735));
#9747=CARTESIAN_POINT('Ctrl Pts',(-38.0493539639435,-32.2463504309186,0.47635415767705));
#9748=CARTESIAN_POINT('Ctrl Pts',(-40.8305797366192,-32.8592858406621,0.317569438451369));
#9749=CARTESIAN_POINT('Ctrl Pts',(-42.8509964848744,-30.8479863606262,0.158784719225683));
#9750=CARTESIAN_POINT('Ctrl Pts',(-42.4575265280738,-29.000351103447,0.0529282397418946));
#9751=CARTESIAN_POINT('Ctrl Pts',(-41.9134659966651,-28.364012796625,0.));
#9752=CARTESIAN_POINT('Ctrl Pts',(-41.9134659966651,-28.364012796625,0.));
#9753=CARTESIAN_POINT('Ctrl Pts',(-41.97507870596,-28.4219136142157,-2.29978767839653E-16));
#9754=CARTESIAN_POINT('Ctrl Pts',(-42.0333202365815,-28.4829649481258,-3.12714122755679E-15));
#9755=CARTESIAN_POINT('Ctrl Pts',(-42.0881937026029,-28.5467819994154,-2.99760216648792E-15));
#9756=CARTESIAN_POINT('Ctrl Pts',(-42.1445198537573,-28.6122885026088,-2.86463377095567E-15));
#9757=CARTESIAN_POINT('Ctrl Pts',(-42.1972976877423,-28.680709529004,1.07456140052229E-15));
#9758=CARTESIAN_POINT('Ctrl Pts',(-42.24650502312,-28.7516774566258,1.11022302462516E-16));
#9759=CARTESIAN_POINT('Ctrl Pts',(-42.2974066658948,-28.825088952545,-8.8569338215283E-16));
#9760=CARTESIAN_POINT('Ctrl Pts',(-42.3444882808169,-28.9012262809001,-8.80673490056425E-16));
#9761=CARTESIAN_POINT('Ctrl Pts',(-42.3876903859773,-28.97972651679,-1.16573417585641E-15));
#9762=CARTESIAN_POINT('Ctrl Pts',(-42.406591306985,-29.0140703699918,-1.29044822589391E-15));
#9763=CARTESIAN_POINT('Ctrl Pts',(-42.4247491715561,-29.0488670047462,-1.72595682164476E-16));
#9764=CARTESIAN_POINT('Ctrl Pts',(-42.442156553419,-29.0840881184884,-3.33066907387547E-16));
#9765=CARTESIAN_POINT('Ctrl Pts',(-42.4516647905079,-29.1033265486346,-4.20719287704412E-16));
#9766=CARTESIAN_POINT('Ctrl Pts',(-42.4609490902037,-29.1226916438214,-1.13385884475685E-15));
#9767=CARTESIAN_POINT('Ctrl Pts',(-42.4700080385928,-29.1421789203223,-1.33226762955019E-15));
#9768=CARTESIAN_POINT('Ctrl Pts',(-42.4786580277956,-29.1607864588671,-1.52171940391727E-15));
#9769=CARTESIAN_POINT('Ctrl Pts',(-42.4871050433881,-29.1795113953271,-3.9883529154072E-15));
#9770=CARTESIAN_POINT('Ctrl Pts',(-42.4953337543378,-29.1983170459912,-3.88578058618805E-15));
#9771=CARTESIAN_POINT('Ctrl Pts',(-42.5318945025042,-29.2818718897858,-3.43004443014503E-15));
#9772=CARTESIAN_POINT('Ctrl Pts',(-42.5641950342821,-29.3671101952375,-2.5754712386216E-15));
#9773=CARTESIAN_POINT('Ctrl Pts',(-42.5922110799965,-29.4536331140717,-2.35922392732846E-15));
#9774=CARTESIAN_POINT('Ctrl Pts',(-42.6206894211336,-29.5415837557814,-2.139408298678E-15));
#9775=CARTESIAN_POINT('Ctrl Pts',(-42.6447412041289,-29.6308625113997,-3.93501828575153E-15));
#9776=CARTESIAN_POINT('Ctrl Pts',(-42.6643018301641,-29.7210875893022,-5.10702591327572E-15));
#9777=CARTESIAN_POINT('Ctrl Pts',(-42.6835241892463,-29.8097523816524,-6.25876571049136E-15));
#9778=CARTESIAN_POINT('Ctrl Pts',(-42.6984096404725,-29.8993319586104,-3.13934285479542E-15));
#9779=CARTESIAN_POINT('Ctrl Pts',(-42.7088541783029,-29.9894868403159,-3.69149155687865E-15));
#9780=CARTESIAN_POINT('Ctrl Pts',(-42.7129843170356,-30.0251372611314,-3.90983063302867E-15));
#9781=CARTESIAN_POINT('Ctrl Pts',(-42.7164195379488,-30.0608778227311,-2.05747673366752E-15));
#9782=CARTESIAN_POINT('Ctrl Pts',(-42.7191513809188,-30.0966880684131,-1.99840144432528E-15));
#9783=CARTESIAN_POINT('Ctrl Pts',(-42.7207682803523,-30.1178831248609,-1.96343647638277E-15));
#9784=CARTESIAN_POINT('Ctrl Pts',(-42.7221387557394,-30.1391025965479,-2.80327539784527E-15));
#9785=CARTESIAN_POINT('Ctrl Pts',(-42.7232608505681,-30.1603422648391,-3.08086889333481E-15));
#9786=CARTESIAN_POINT('Ctrl Pts',(-42.72400775337,-30.1744800786414,-3.26564414962369E-15));
#9787=CARTESIAN_POINT('Ctrl Pts',(-42.7246445276711,-30.1886268373637,-4.89221388773611E-16));
#9788=CARTESIAN_POINT('Ctrl Pts',(-42.7251702454122,-30.2027667406769,-6.10622663543836E-16));
#9789=CARTESIAN_POINT('Ctrl Pts',(-42.7287089699826,-30.2979456158974,-1.42780199830197E-15));
#9790=CARTESIAN_POINT('Ctrl Pts',(-42.7272289680734,-30.3929754547405,1.61702128845623E-15));
#9791=CARTESIAN_POINT('Ctrl Pts',(-42.7206715932526,-30.4874575333237,1.08246744900953E-15));
#9792=CARTESIAN_POINT('Ctrl Pts',(-42.7141367060633,-30.5816155983765,5.49746789773547E-16));
#9793=CARTESIAN_POINT('Ctrl Pts',(-42.7025595698505,-30.675230607113,-3.71437912378399E-15));
#9794=CARTESIAN_POINT('Ctrl Pts',(-42.6858341417982,-30.7679258265936,-4.91273688396632E-15));
#9795=CARTESIAN_POINT('Ctrl Pts',(-42.6838972772188,-30.7786602656003,-5.05151101230811E-15));
#9796=CARTESIAN_POINT('Ctrl Pts',(-42.6818913149789,-30.7893823802406,-1.99705768075859E-15));
#9797=CARTESIAN_POINT('Ctrl Pts',(-42.6798160451629,-30.8000915919209,-1.99840144432528E-15));
#9798=CARTESIAN_POINT('Ctrl Pts',(-42.662271111955,-30.8906303749705,-2.01079479026814E-15));
#9799=CARTESIAN_POINT('Ctrl Pts',(-42.639776801042,-30.9802472256389,-1.59062155688729E-16));
#9800=CARTESIAN_POINT('Ctrl Pts',(-42.6126084037943,-31.0687042177952,1.11022302462516E-15));
#9801=CARTESIAN_POINT('Ctrl Pts',(-42.6018601180323,-31.1036993270272,1.61237409769298E-15));
#9802=CARTESIAN_POINT('Ctrl Pts',(-42.5903796970892,-31.1385128525821,-4.92893737492136E-16));
#9803=CARTESIAN_POINT('Ctrl Pts',(-42.5781819927525,-31.1731297199112,-6.66133814775094E-16));
#9804=CARTESIAN_POINT('Ctrl Pts',(-42.5722275134488,-31.190028425961,-7.50703371986377E-16));
#9805=CARTESIAN_POINT('Ctrl Pts',(-42.5661020845814,-31.2068802633122,-2.00401734812381E-15));
#9806=CARTESIAN_POINT('Ctrl Pts',(-42.5598073328338,-31.2236834501749,-2.02615701994091E-15));
#9807=CARTESIAN_POINT('Ctrl Pts',(-42.5545628516665,-31.2376830486637,-2.04460271828635E-15));
#9808=CARTESIAN_POINT('Ctrl Pts',(-42.5492037320733,-31.2516410674552,2.43968211885899E-16));
#9809=CARTESIAN_POINT('Ctrl Pts',(-42.5437331875382,-31.2655519281032,1.38777878078145E-16));
#9810=CARTESIAN_POINT('Ctrl Pts',(-42.5095085757547,-31.3525805231897,-5.19309870738232E-16));
#9811=CARTESIAN_POINT('Ctrl Pts',(-42.4709055243979,-31.4378209883345,4.76536274428084E-16));
#9812=CARTESIAN_POINT('Ctrl Pts',(-42.4282565184601,-31.5210414522706,3.33066907387547E-16));
#9813=CARTESIAN_POINT('Ctrl Pts',(-42.3840273012413,-31.6073453624215,1.84281779585565E-16));
#9814=CARTESIAN_POINT('Ctrl Pts',(-42.3354466279213,-31.6914775359273,4.72784736073334E-16));
#9815=CARTESIAN_POINT('Ctrl Pts',(-42.2828293656982,-31.7731758332943,4.85722573273506E-16));
#9816=CARTESIAN_POINT('Ctrl Pts',(-42.229634476967,-31.8557710055697,4.98802440625183E-16));
#9817=CARTESIAN_POINT('Ctrl Pts',(-42.1723134681871,-31.9358793885275,-6.12161291006381E-16));
#9818=CARTESIAN_POINT('Ctrl Pts',(-42.1111400734139,-32.0132147571248,-4.85722573273506E-16));
#9819=CARTESIAN_POINT('Ctrl Pts',(-42.0873228863003,-32.0433244306392,-4.36495051900537E-16));
#9820=CARTESIAN_POINT('Ctrl Pts',(-42.0629212212804,-32.0730135273603,-5.06570471742106E-15));
#9821=CARTESIAN_POINT('Ctrl Pts',(-42.0379493675179,-32.1022641150462,-5.35682609381638E-15));
#9822=CARTESIAN_POINT('Ctrl Pts',(-42.0179603023369,-32.1256781518813,-5.58985821965319E-15));
#9823=CARTESIAN_POINT('Ctrl Pts',(-41.997605872731,-32.1488112067583,-9.77501083290033E-16));
#9824=CARTESIAN_POINT('Ctrl Pts',(-41.9768929709471,-32.1716537402857,-1.08246744900953E-15));
#9825=CARTESIAN_POINT('Ctrl Pts',(-41.9653469750443,-32.184386857126,-1.14097886576662E-15));
#9826=CARTESIAN_POINT('Ctrl Pts',(-41.9536946662295,-32.1970240341331,-1.52433067033023E-15));
#9827=CARTESIAN_POINT('Ctrl Pts',(-41.9419422851552,-32.2095588617621,-1.346145417358E-15));
#9828=CARTESIAN_POINT('Ctrl Pts',(-41.8728869093774,-32.2832117859446,-2.99153363207995E-16));
#9829=CARTESIAN_POINT('Ctrl Pts',(-41.8003309454798,-32.3533872730139,-3.08633678840453E-15));
#9830=CARTESIAN_POINT('Ctrl Pts',(-41.7245863310056,-32.4197964723545,-1.84574577843932E-15));
#9831=CARTESIAN_POINT('Ctrl Pts',(-41.6603355224085,-32.4761284609128,-7.93407257979879E-16));
#9832=CARTESIAN_POINT('Ctrl Pts',(-41.5937892971726,-32.5297504849909,-1.35961820572097E-15));
#9833=CARTESIAN_POINT('Ctrl Pts',(-41.5251131887883,-32.5804713188053,-2.43555176027144E-15));
#9834=CARTESIAN_POINT('Ctrl Pts',(-41.502422805649,-32.5972293323193,-2.79103702522908E-15));
#9835=CARTESIAN_POINT('Ctrl Pts',(-41.4794997526171,-32.6136705085288,1.28421174174714E-15));
#9836=CARTESIAN_POINT('Ctrl Pts',(-41.456349528936,-32.6297875098032,1.76941794549634E-15));
#9837=CARTESIAN_POINT('Ctrl Pts',(-41.4397562694643,-32.6413396048385,2.11719654785573E-15));
#9838=CARTESIAN_POINT('Ctrl Pts',(-41.4230453329585,-32.6527256775375,-2.01867653155568E-16));
#9839=CARTESIAN_POINT('Ctrl Pts',(-41.4062333015004,-32.663933539865,-3.33066907387547E-16));
#9840=CARTESIAN_POINT('Ctrl Pts',(-41.3198795013252,-32.721501925115,-1.00696251668964E-15));
#9841=CARTESIAN_POINT('Ctrl Pts',(-41.2307763067095,-32.7744320587763,-3.13830639635427E-15));
#9842=CARTESIAN_POINT('Ctrl Pts',(-41.139232260598,-32.8224024784536,-3.40005801291454E-15));
#9843=CARTESIAN_POINT('Ctrl Pts',(-41.0476882144866,-32.870372898131,-3.66180962947481E-15));
#9844=CARTESIAN_POINT('Ctrl Pts',(-40.9537026715522,-32.9133845145118,-1.77753300593033E-15));
#9845=CARTESIAN_POINT('Ctrl Pts',(-40.857546131199,-32.9510751186699,-1.72127936903799E-15));
#9846=CARTESIAN_POINT('Ctrl Pts',(-40.8369781689331,-32.9591371695845,-1.70558910776797E-15));
#9847=CARTESIAN_POINT('Ctrl Pts',(-40.8163107577518,-32.966955588126,-7.07161017401445E-17));
#9848=CARTESIAN_POINT('Ctrl Pts',(-40.7955478019229,-32.974531551058,2.77555756156289E-17));
#9849=CARTESIAN_POINT('Ctrl Pts',(-42.5142225916618,-29.9985870806183,9.11258330249199));
#9850=CARTESIAN_POINT('Ctrl Pts',(-42.5159019272474,-29.6714493029011,9.09196520028265));
#9851=CARTESIAN_POINT('Ctrl Pts',(-42.4566449317272,-29.3448946486763,9.07134709807331));
#9852=CARTESIAN_POINT('Ctrl Pts',(-42.3336251416166,-29.0444505140773,9.05072899586397));
#9853=CARTESIAN_POINT('Ctrl Pts',(-42.017823964677,-28.2731875227676,8.99780075612208));
#9854=CARTESIAN_POINT('Ctrl Pts',(-41.281833604806,-27.6739897299479,8.94487251638018));
#9855=CARTESIAN_POINT('Ctrl Pts',(-40.4625634711727,-27.521115323398,8.89194427663829));
#9856=CARTESIAN_POINT('Ctrl Pts',(-39.6432933375393,-27.368240916848,8.83901603689639));
#9857=CARTESIAN_POINT('Ctrl Pts',(-38.7407434301437,-27.6616898965678,8.7860877971545));
#9858=CARTESIAN_POINT('Ctrl Pts',(-38.1680405528962,-28.2671482558857,8.7331595574126));
#9859=CARTESIAN_POINT('Ctrl Pts',(-37.5953376756488,-28.8726066152036,8.68023131767071));
#9860=CARTESIAN_POINT('Ctrl Pts',(-37.3524818285495,-29.7900743541197,8.62730307792881));
#9861=CARTESIAN_POINT('Ctrl Pts',(-37.5506422560009,-30.5995832662067,8.57437483818692));
#9862=CARTESIAN_POINT('Ctrl Pts',(-37.7488026834523,-31.4090921782936,8.52144659844502));
#9863=CARTESIAN_POINT('Ctrl Pts',(-38.3879793854543,-32.1106422635514,8.46851835870313));
#9864=CARTESIAN_POINT('Ctrl Pts',(-39.1755925100941,-32.3831072318185,8.41559011896124));
#9865=CARTESIAN_POINT('Ctrl Pts',(-39.963205634734,-32.6555722000855,8.36266187921934));
#9866=CARTESIAN_POINT('Ctrl Pts',(-40.8992551820115,-32.4989520513618,8.30973363947745));
#9867=CARTESIAN_POINT('Ctrl Pts',(-41.5552732023909,-31.9849371299697,8.25680539973555));
#9868=CARTESIAN_POINT('Ctrl Pts',(-42.1511258460839,-31.518064055916,8.20873136732103));
#9869=CARTESIAN_POINT('Ctrl Pts',(-42.5159566006121,-30.7563455532992,8.16065733490651));
#9870=CARTESIAN_POINT('Ctrl Pts',(-42.5208030005754,-29.9986726513939,8.11258330249199));
#9871=CARTESIAN_POINT('Ctrl Pts',(-40.7937992825329,-32.9692229537457,10.));
#9872=CARTESIAN_POINT('Ctrl Pts',(-40.8868533728222,-32.935183351848,10.));
#9873=CARTESIAN_POINT('Ctrl Pts',(-40.9778402395471,-32.8963743016634,10.));
#9874=CARTESIAN_POINT('Ctrl Pts',(-41.0665521014268,-32.8531245323668,10.));
#9875=CARTESIAN_POINT('Ctrl Pts',(-41.1572337566638,-32.8089144280433,10.));
#9876=CARTESIAN_POINT('Ctrl Pts',(-41.245538922155,-32.7600635910313,10.));
#9877=CARTESIAN_POINT('Ctrl Pts',(-41.3312167295181,-32.7068775848614,10.));
#9878=CARTESIAN_POINT('Ctrl Pts',(-41.414166125894,-32.6553852878102,10.));
#9879=CARTESIAN_POINT('Ctrl Pts',(-41.4946531615533,-32.5998286696066,10.));
#9880=CARTESIAN_POINT('Ctrl Pts',(-41.5724164694193,-32.540454332485,10.));
#9881=CARTESIAN_POINT('Ctrl Pts',(-41.6404593638021,-32.4885017875035,10.));
#9882=CARTESIAN_POINT('Ctrl Pts',(-41.706416607328,-32.4336255845195,10.));
#9883=CARTESIAN_POINT('Ctrl Pts',(-41.7700878401902,-32.375977951992,10.));
#9884=CARTESIAN_POINT('Ctrl Pts',(-41.7834304287881,-32.3638976354993,10.));
#9885=CARTESIAN_POINT('Ctrl Pts',(-41.7966744017855,-32.3516937148243,10.));
#9886=CARTESIAN_POINT('Ctrl Pts',(-41.8098007360623,-32.3393838948222,10.));
#9887=CARTESIAN_POINT('Ctrl Pts',(-41.8822283307573,-32.2714616070702,10.));
#9888=CARTESIAN_POINT('Ctrl Pts',(-41.9511902075176,-32.2002181058656,10.));
#9889=CARTESIAN_POINT('Ctrl Pts',(-42.0164470228621,-32.125944563464,10.));
#9890=CARTESIAN_POINT('Ctrl Pts',(-42.081342504664,-32.0520822811284,10.));
#9891=CARTESIAN_POINT('Ctrl Pts',(-42.142574327181,-31.9752226218996,10.));
#9892=CARTESIAN_POINT('Ctrl Pts',(-42.199863486846,-31.8956252027112,10.));
#9893=CARTESIAN_POINT('Ctrl Pts',(-42.2557185827112,-31.8180202682806,10.));
#9894=CARTESIAN_POINT('Ctrl Pts',(-42.3078262008549,-31.7378121817919,10.));
#9895=CARTESIAN_POINT('Ctrl Pts',(-42.3558809073996,-31.6552274273718,10.));
#9896=CARTESIAN_POINT('Ctrl Pts',(-42.3766084917365,-31.6196058913086,10.));
#9897=CARTESIAN_POINT('Ctrl Pts',(-42.3965814143594,-31.5835420633842,10.));
#9898=CARTESIAN_POINT('Ctrl Pts',(-42.4157721815743,-31.5470537860881,10.));
#9899=CARTESIAN_POINT('Ctrl Pts',(-42.4294375496695,-31.5210712010862,10.));
#9900=CARTESIAN_POINT('Ctrl Pts',(-42.4427062812236,-31.4948733921638,10.));
#9901=CARTESIAN_POINT('Ctrl Pts',(-42.4555678526521,-31.4684667979364,10.));
#9902=CARTESIAN_POINT('Ctrl Pts',(-42.4611833574038,-31.4569373859838,10.));
#9903=CARTESIAN_POINT('Ctrl Pts',(-42.4667203177096,-31.4453699707948,10.));
#9904=CARTESIAN_POINT('Ctrl Pts',(-42.4721741634146,-31.4337733648849,10.));
#9905=CARTESIAN_POINT('Ctrl Pts',(-42.5124020023045,-31.3482362192731,10.));
#9906=CARTESIAN_POINT('Ctrl Pts',(-42.5481738032464,-31.2609859402736,10.));
#9907=CARTESIAN_POINT('Ctrl Pts',(-42.5792385873022,-31.1722598487437,10.));
#9908=CARTESIAN_POINT('Ctrl Pts',(-42.6096166607224,-31.085495114827,10.));
#9909=CARTESIAN_POINT('Ctrl Pts',(-42.6354937388761,-30.997318420516,10.));
#9910=CARTESIAN_POINT('Ctrl Pts',(-42.6565860035544,-30.9079428775445,10.));
#9911=CARTESIAN_POINT('Ctrl Pts',(-42.6603146693337,-30.8921431740198,10.));
#9912=CARTESIAN_POINT('Ctrl Pts',(-42.6638936748766,-30.8763059973636,10.));
#9913=CARTESIAN_POINT('Ctrl Pts',(-42.6673212800257,-30.8604325193031,10.));
#9914=CARTESIAN_POINT('Ctrl Pts',(-42.6874321817243,-30.7672975335032,10.));
#9915=CARTESIAN_POINT('Ctrl Pts',(-42.7023351154996,-30.6729118079479,10.));
#9916=CARTESIAN_POINT('Ctrl Pts',(-42.7121085725822,-30.5776842387582,10.));
#9917=CARTESIAN_POINT('Ctrl Pts',(-42.7153864632551,-30.5457461478441,10.));
#9918=CARTESIAN_POINT('Ctrl Pts',(-42.7180869507972,-30.5137134838219,10.));
#9919=CARTESIAN_POINT('Ctrl Pts',(-42.7202117715535,-30.4816021420478,10.));
#9920=CARTESIAN_POINT('Ctrl Pts',(-42.7214003930878,-30.4636391057704,10.));
#9921=CARTESIAN_POINT('Ctrl Pts',(-42.7224088624834,-30.4456514543982,10.));
#9922=CARTESIAN_POINT('Ctrl Pts',(-42.723237404335,-30.427642015416,10.));
#9923=CARTESIAN_POINT('Ctrl Pts',(-42.7238116710756,-30.4151595779797,10.));
#9924=CARTESIAN_POINT('Ctrl Pts',(-42.7242993863234,-30.4026682033291,10.));
#9925=CARTESIAN_POINT('Ctrl Pts',(-42.7247004999338,-30.3901783131038,10.));
#9926=CARTESIAN_POINT('Ctrl Pts',(-42.7276933286286,-30.296987504066,10.));
#9927=CARTESIAN_POINT('Ctrl Pts',(-42.7258765702513,-30.2037322455153,10.));
#9928=CARTESIAN_POINT('Ctrl Pts',(-42.7193893277119,-30.1107876657792,10.));
#9929=CARTESIAN_POINT('Ctrl Pts',(-42.7128891265852,-30.0176574246571,10.));
#9930=CARTESIAN_POINT('Ctrl Pts',(-42.70169938016,-29.9248381231515,10.));
#9931=CARTESIAN_POINT('Ctrl Pts',(-42.6859089810961,-29.8327191439709,10.));
#9932=CARTESIAN_POINT('Ctrl Pts',(-42.6703416896879,-29.7419017436428,10.));
#9933=CARTESIAN_POINT('Ctrl Pts',(-42.6503023675462,-29.6517641681989,10.));
#9934=CARTESIAN_POINT('Ctrl Pts',(-42.625833145288,-29.5627046786781,10.));
#9935=CARTESIAN_POINT('Ctrl Pts',(-42.6163194806669,-29.5280782362974,10.));
#9936=CARTESIAN_POINT('Ctrl Pts',(-42.6061357356979,-29.4936151031392,10.));
#9937=CARTESIAN_POINT('Ctrl Pts',(-42.5952828198538,-29.4593401489932,10.));
#9938=CARTESIAN_POINT('Ctrl Pts',(-42.5894786042462,-29.4410096628213,10.));
#9939=CARTESIAN_POINT('Ctrl Pts',(-42.5834829790806,-29.422733014913,10.));
#9940=CARTESIAN_POINT('Ctrl Pts',(-42.5772959877695,-29.4045141238123,10.));
#9941=CARTESIAN_POINT('Ctrl Pts',(-42.5718473975396,-29.3884696092719,10.));
#9942=CARTESIAN_POINT('Ctrl Pts',(-42.566249914374,-29.3724688136786,10.));
#9943=CARTESIAN_POINT('Ctrl Pts',(-42.560509689398,-29.3565308232038,10.));
#9944=CARTESIAN_POINT('Ctrl Pts',(-42.528084217673,-29.2665000558295,10.));
#9945=CARTESIAN_POINT('Ctrl Pts',(-42.4910677016941,-29.1783480221378,10.));
#9946=CARTESIAN_POINT('Ctrl Pts',(-42.4495331756161,-29.0925192906336,10.));
#9947=CARTESIAN_POINT('Ctrl Pts',(-42.4183822810576,-29.0281477420054,10.));
#9948=CARTESIAN_POINT('Ctrl Pts',(-42.3846888574719,-28.965083587818,10.));
#9949=CARTESIAN_POINT('Ctrl Pts',(-42.3484663478005,-28.9035315373059,10.));
#9950=CARTESIAN_POINT('Ctrl Pts',(-42.3335345656046,-28.8781583144039,10.));
#9951=CARTESIAN_POINT('Ctrl Pts',(-42.3181728564796,-28.8530422408006,10.));
#9952=CARTESIAN_POINT('Ctrl Pts',(-42.3023815042107,-28.8281985617541,10.));
#9953=CARTESIAN_POINT('Ctrl Pts',(-42.2929488646612,-28.813358700953,10.));
#9954=CARTESIAN_POINT('Ctrl Pts',(-42.2833676059461,-28.7986234509943,10.));
#9955=CARTESIAN_POINT('Ctrl Pts',(-42.2736397669503,-28.7839981335806,10.));
#9956=CARTESIAN_POINT('Ctrl Pts',(-42.2261110872739,-28.7125411505014,10.));
#9957=CARTESIAN_POINT('Ctrl Pts',(-42.1750736185291,-28.6436861425009,10.));
#9958=CARTESIAN_POINT('Ctrl Pts',(-42.1205617426708,-28.5777858210467,10.));
#9959=CARTESIAN_POINT('Ctrl Pts',(-42.0689757131425,-28.5154226043176,10.));
#9960=CARTESIAN_POINT('Ctrl Pts',(-42.0142777437963,-28.4557051898554,10.));
#9961=CARTESIAN_POINT('Ctrl Pts',(-41.9564731814538,-28.3989683641584,10.));
#9962=CARTESIAN_POINT('Ctrl Pts',(-41.9435072079919,-28.3862418916018,10.));
#9963=CARTESIAN_POINT('Ctrl Pts',(-41.9303848447124,-28.3736655421759,10.));
#9964=CARTESIAN_POINT('Ctrl Pts',(-41.9171093217587,-28.3612406458478,10.));
#9965=CARTESIAN_POINT('Origin',(0.,0.,10.));
#9966=CARTESIAN_POINT('',(-60.,50.,10.));
#9967=CARTESIAN_POINT('',(-60.,-50.,10.));
#9968=CARTESIAN_POINT('',(-60.,50.,10.));
#9969=CARTESIAN_POINT('',(60.,-50.,10.));
#9970=CARTESIAN_POINT('',(-60.,-50.,10.));
#9971=CARTESIAN_POINT('',(60.,50.,10.));
#9972=CARTESIAN_POINT('',(60.,-50.,10.));
#9973=CARTESIAN_POINT('',(60.,50.,10.));
#9974=CARTESIAN_POINT('Ctrl Pts',(41.9134659966651,-28.364012796625,10.));
#9975=CARTESIAN_POINT('Ctrl Pts',(41.9750786768602,-28.4219135868691,10.));
#9976=CARTESIAN_POINT('Ctrl Pts',(42.0333201769005,-28.4829648953928,10.));
#9977=CARTESIAN_POINT('Ctrl Pts',(42.0881936118187,-28.5467819227993,10.));
#9978=CARTESIAN_POINT('Ctrl Pts',(42.1445197342576,-28.612288405212,10.));
#9979=CARTESIAN_POINT('Ctrl Pts',(42.1972975385705,-28.6807094127424,10.));
#9980=CARTESIAN_POINT('Ctrl Pts',(42.2465048443317,-28.7516773228468,10.));
#9981=CARTESIAN_POINT('Ctrl Pts',(42.2974064829938,-28.8250888388982,10.));
#9982=CARTESIAN_POINT('Ctrl Pts',(42.3444880898825,-28.901226191665,10.));
#9983=CARTESIAN_POINT('Ctrl Pts',(42.3876901841144,-28.9797264550545,10.));
#9984=CARTESIAN_POINT('Ctrl Pts',(42.4065911003408,-29.0140703202873,10.));
#9985=CARTESIAN_POINT('Ctrl Pts',(42.4247489595759,-29.0488669676648,10.));
#9986=CARTESIAN_POINT('Ctrl Pts',(42.442156335631,-29.0840880945258,10.));
#9987=CARTESIAN_POINT('Ctrl Pts',(42.4516645839391,-29.1033265609567,10.));
#9988=CARTESIAN_POINT('Ctrl Pts',(42.4609488940356,-29.1226916929596,10.));
#9989=CARTESIAN_POINT('Ctrl Pts',(42.4700078520136,-29.1421790067722,10.));
#9990=CARTESIAN_POINT('Ctrl Pts',(42.4786578515885,-29.1607865835603,10.));
#9991=CARTESIAN_POINT('Ctrl Pts',(42.4871048767656,-29.1795115587778,10.));
#9992=CARTESIAN_POINT('Ctrl Pts',(42.4953335964791,-29.1983172485575,10.));
#9993=CARTESIAN_POINT('Ctrl Pts',(42.5318943081609,-29.2818720937771,10.));
#9994=CARTESIAN_POINT('Ctrl Pts',(42.5641948048895,-29.3671104009095,10.));
#9995=CARTESIAN_POINT('Ctrl Pts',(42.592210818053,-29.4536333209677,10.));
#9996=CARTESIAN_POINT('Ctrl Pts',(42.6206891306107,-29.5415839778454,10.));
#9997=CARTESIAN_POINT('Ctrl Pts',(42.644740886205,-29.6308627485803,10.));
#9998=CARTESIAN_POINT('Ctrl Pts',(42.6643014871103,-29.7210878406195,10.));
#9999=CARTESIAN_POINT('Ctrl Pts',(42.6835238259951,-29.8097526676095,10.));
#10000=CARTESIAN_POINT('Ctrl Pts',(42.698409257187,-29.89933227869,10.));
#10001=CARTESIAN_POINT('Ctrl Pts',(42.7088537761227,-29.9894871928845,10.));
#10002=CARTESIAN_POINT('Ctrl Pts',(42.7129839090531,-30.0251376409564,10.));
#10003=CARTESIAN_POINT('Ctrl Pts',(42.7164191237806,-30.0608782296299,10.));
#10004=CARTESIAN_POINT('Ctrl Pts',(42.7191509602312,-30.0966885021091,10.));
#10005=CARTESIAN_POINT('Ctrl Pts',(42.7207678549321,-30.1178835629617,10.));
#10006=CARTESIAN_POINT('Ctrl Pts',(42.7221383257361,-30.1391030389302,10.));
#10007=CARTESIAN_POINT('Ctrl Pts',(42.7232604161444,-30.1603427113668,10.));
#10008=CARTESIAN_POINT('Ctrl Pts',(42.7240073161938,-30.1744805315225,10.));
#10009=CARTESIAN_POINT('Ctrl Pts',(42.7246440877591,-30.1886272965526,10.));
#10010=CARTESIAN_POINT('Ctrl Pts',(42.7251698027865,-30.2027672061038,10.));
#10011=CARTESIAN_POINT('Ctrl Pts',(42.7287085081136,-30.2979460970433,10.));
#10012=CARTESIAN_POINT('Ctrl Pts',(42.7272284907081,-30.3929759486328,10.));
#10013=CARTESIAN_POINT('Ctrl Pts',(42.7206711052329,-30.4874580359568,10.));
#10014=CARTESIAN_POINT('Ctrl Pts',(42.714136206117,-30.5816161285794,10.));
#10015=CARTESIAN_POINT('Ctrl Pts',(42.7025590607659,-30.6752311606915,10.));
#10016=CARTESIAN_POINT('Ctrl Pts',(42.6858336273981,-30.7679263980985,10.));
#10017=CARTESIAN_POINT('Ctrl Pts',(42.6838967626779,-30.7786608365503,10.));
#10018=CARTESIAN_POINT('Ctrl Pts',(42.6818908003822,-30.7893829505687,10.));
#10019=CARTESIAN_POINT('Ctrl Pts',(42.6798155305974,-30.8000921615584,10.));
#10020=CARTESIAN_POINT('Ctrl Pts',(42.6622705920295,-30.8906309677886,10.));
#10021=CARTESIAN_POINT('Ctrl Pts',(42.6397762787909,-30.9802478361479,10.));
#10022=CARTESIAN_POINT('Ctrl Pts',(42.6126078815683,-31.0687048411986,10.));
#10023=CARTESIAN_POINT('Ctrl Pts',(42.6018595917985,-31.1036999686133,10.));
#10024=CARTESIAN_POINT('Ctrl Pts',(42.5903791666683,-31.1385135114639,10.));
#10025=CARTESIAN_POINT('Ctrl Pts',(42.5781814579395,-31.173130395225,10.));
#10026=CARTESIAN_POINT('Ctrl Pts',(42.5722268554977,-31.1900294526755,10.));
#10027=CARTESIAN_POINT('Ctrl Pts',(42.5661012964961,-31.2068816393169,10.));
#10028=CARTESIAN_POINT('Ctrl Pts',(42.5598064077136,-31.223685173253,10.));
#10029=CARTESIAN_POINT('Ctrl Pts',(42.5545620438917,-31.237684442899,10.));
#10030=CARTESIAN_POINT('Ctrl Pts',(42.549203047486,-31.2516421336463,10.));
#10031=CARTESIAN_POINT('Ctrl Pts',(42.5437326312534,-31.265552668785,10.));
#10032=CARTESIAN_POINT('Ctrl Pts',(42.5095080157812,-31.3525812779227,10.));
#10033=CARTESIAN_POINT('Ctrl Pts',(42.4709049618174,-31.4378217521669,10.));
#10034=CARTESIAN_POINT('Ctrl Pts',(42.4282559537337,-31.5210422209145,10.));
#10035=CARTESIAN_POINT('Ctrl Pts',(42.3840267420549,-31.6073461209027,10.));
#10036=CARTESIAN_POINT('Ctrl Pts',(42.335446076298,-31.6914782803964,10.));
#10037=CARTESIAN_POINT('Ctrl Pts',(42.2828288228026,-31.7731765607072,10.));
#10038=CARTESIAN_POINT('Ctrl Pts',(42.2296339485798,-31.8557717069121,10.));
#10039=CARTESIAN_POINT('Ctrl Pts',(42.1723129563808,-31.9358800612183,10.));
#10040=CARTESIAN_POINT('Ctrl Pts',(42.1111395793052,-32.013215399448,10.));
#10041=CARTESIAN_POINT('Ctrl Pts',(42.087322330385,-32.0433251479856,10.));
#10042=CARTESIAN_POINT('Ctrl Pts',(42.0629206003569,-32.0730143170435,10.));
#10043=CARTESIAN_POINT('Ctrl Pts',(42.0379486784512,-32.1022649742732,10.));
#10044=CARTESIAN_POINT('Ctrl Pts',(42.0179581141926,-32.1256807588157,10.));
#10045=CARTESIAN_POINT('Ctrl Pts',(41.9976021306956,-32.1488155190018,10.));
#10046=CARTESIAN_POINT('Ctrl Pts',(41.9768876217174,-32.1716597133009,10.));
#10047=CARTESIAN_POINT('Ctrl Pts',(41.9653431028421,-32.1843911390157,10.));
#10048=CARTESIAN_POINT('Ctrl Pts',(41.9536923027656,-32.1970266455306,10.));
#10049=CARTESIAN_POINT('Ctrl Pts',(41.9419414550198,-32.2095598310127,10.));
#10050=CARTESIAN_POINT('Ctrl Pts',(41.8728860824193,-32.2832127122403,10.));
#10051=CARTESIAN_POINT('Ctrl Pts',(41.8003301222597,-32.3533881546089,10.));
#10052=CARTESIAN_POINT('Ctrl Pts',(41.7245855110489,-32.4197973083236,10.));
#10053=CARTESIAN_POINT('Ctrl Pts',(41.6603347701438,-32.4761292012575,10.));
#10054=CARTESIAN_POINT('Ctrl Pts',(41.593788616895,-32.5297511345173,10.));
#10055=CARTESIAN_POINT('Ctrl Pts',(41.5251125836829,-32.5804718833742,10.));
#10056=CARTESIAN_POINT('Ctrl Pts',(41.5024215392248,-32.5972303755792,10.));
#10057=CARTESIAN_POINT('Ctrl Pts',(41.4794978111518,-32.6136720119584,10.));
#10058=CARTESIAN_POINT('Ctrl Pts',(41.4563468991644,-32.6297894542513,10.));
#10059=CARTESIAN_POINT('Ctrl Pts',(41.4397544793987,-32.6413409373297,10.));
#10060=CARTESIAN_POINT('Ctrl Pts',(41.4230443952104,-32.6527264145468,10.));
#10061=CARTESIAN_POINT('Ctrl Pts',(41.406233226403,-32.6639336995976,10.));
#10062=CARTESIAN_POINT('Ctrl Pts',(41.3198794645924,-32.7215020480517,10.));
#10063=CARTESIAN_POINT('Ctrl Pts',(41.2307763069737,-32.7744321483762,10.));
#10064=CARTESIAN_POINT('Ctrl Pts',(41.1392322953199,-32.8224025393254,10.));
#10065=CARTESIAN_POINT('Ctrl Pts',(41.0476882836661,-32.8703729302747,10.));
#10066=CARTESIAN_POINT('Ctrl Pts',(40.9537027726528,-32.9133845225335,10.));
#10067=CARTESIAN_POINT('Ctrl Pts',(40.8575462605233,-32.95107510836,10.));
#10068=CARTESIAN_POINT('Ctrl Pts',(40.8369783011898,-32.9591371565704,10.));
#10069=CARTESIAN_POINT('Ctrl Pts',(40.8163108927417,-32.9669555725993,10.));
#10070=CARTESIAN_POINT('Ctrl Pts',(40.795547939453,-32.9745315332036,10.));
#10071=CARTESIAN_POINT('Ctrl Pts',(39.2062007174671,-32.9692229537457,10.));
#10072=CARTESIAN_POINT('Ctrl Pts',(39.1131464644267,-32.9351832923129,10.));
#10073=CARTESIAN_POINT('Ctrl Pts',(39.0221594360209,-32.8963742052227,10.));
#10074=CARTESIAN_POINT('Ctrl Pts',(38.9334474159654,-32.8531244154564,10.));
#10075=CARTESIAN_POINT('Ctrl Pts',(38.8427656811494,-32.8089143302392,10.));
#10076=CARTESIAN_POINT('Ctrl Pts',(38.7544604354353,-32.7600635379137,10.));
#10077=CARTESIAN_POINT('Ctrl Pts',(38.6687825492772,-32.7068775946067,10.));
#10078=CARTESIAN_POINT('Ctrl Pts',(38.5858331739442,-32.6553854188348,10.));
#10079=CARTESIAN_POINT('Ctrl Pts',(38.5053461548915,-32.5998289484912,10.));
#10080=CARTESIAN_POINT('Ctrl Pts',(38.4275828602563,-32.5404547782488,10.));
#10081=CARTESIAN_POINT('Ctrl Pts',(38.3595399774506,-32.4885023792867,10.));
#10082=CARTESIAN_POINT('Ctrl Pts',(38.293582742916,-32.4336263368915,10.));
#10083=CARTESIAN_POINT('Ctrl Pts',(38.2299115171604,-32.3759788744261,10.));
#10084=CARTESIAN_POINT('Ctrl Pts',(38.2165690420241,-32.3638986949496,10.));
#10085=CARTESIAN_POINT('Ctrl Pts',(38.2033251808735,-32.3516949139002,10.));
#10086=CARTESIAN_POINT('Ctrl Pts',(38.190198956418,-32.3393852356562,10.));
#10087=CARTESIAN_POINT('Ctrl Pts',(38.1177713352618,-32.2714631370029,10.));
#10088=CARTESIAN_POINT('Ctrl Pts',(38.0488094314203,-32.2002198323416,10.));
#10089=CARTESIAN_POINT('Ctrl Pts',(37.9835525897255,-32.1259464860604,10.));
#10090=CARTESIAN_POINT('Ctrl Pts',(37.9186571141777,-32.0520844357027,10.));
#10091=CARTESIAN_POINT('Ctrl Pts',(37.8574252949744,-31.9752250110449,10.));
#10092=CARTESIAN_POINT('Ctrl Pts',(37.8001361365983,-31.8956278208525,10.));
#10093=CARTESIAN_POINT('Ctrl Pts',(37.7442810137189,-31.8180230704062,10.));
#10094=CARTESIAN_POINT('Ctrl Pts',(37.6921733704247,-31.7378151599815,10.));
#10095=CARTESIAN_POINT('Ctrl Pts',(37.6441186418705,-31.6552305662644,10.));
#10096=CARTESIAN_POINT('Ctrl Pts',(37.6233910600879,-31.6196091202224,10.));
#10097=CARTESIAN_POINT('Ctrl Pts',(37.6034181397275,-31.5835453799715,10.));
#10098=CARTESIAN_POINT('Ctrl Pts',(37.5842273745413,-31.5470571873502,10.));
#10099=CARTESIAN_POINT('Ctrl Pts',(37.5705621606998,-31.5210749531859,10.));
#10100=CARTESIAN_POINT('Ctrl Pts',(37.5572935744113,-31.4948774983938,10.));
#10101=CARTESIAN_POINT('Ctrl Pts',(37.544432138925,-31.4684712611331,10.));
#10102=CARTESIAN_POINT('Ctrl Pts',(37.5388166989825,-31.4569420162363,10.));
#10103=CARTESIAN_POINT('Ctrl Pts',(37.5332798012255,-31.4453747680287,10.));
#10104=CARTESIAN_POINT('Ctrl Pts',(37.5278260160845,-31.4337783295543,10.));
#10105=CARTESIAN_POINT('Ctrl Pts',(37.4875981325696,-31.3482413741973,10.));
#10106=CARTESIAN_POINT('Ctrl Pts',(37.4518262853914,-31.2609912635665,10.));
#10107=CARTESIAN_POINT('Ctrl Pts',(37.4207614540347,-31.1722653110286,10.));
#10108=CARTESIAN_POINT('Ctrl Pts',(37.3903833312938,-31.0855007042761,10.));
#10109=CARTESIAN_POINT('Ctrl Pts',(37.3645062037076,-30.9973241087638,10.));
#10110=CARTESIAN_POINT('Ctrl Pts',(37.3434138900069,-30.9079486289182,10.));
#10111=CARTESIAN_POINT('Ctrl Pts',(37.3396850724138,-30.8921483299862,10.));
#10112=CARTESIAN_POINT('Ctrl Pts',(37.3361059265609,-30.8763105539293,10.));
#10113=CARTESIAN_POINT('Ctrl Pts',(37.3326781928098,-30.8604364725678,10.));
#10114=CARTESIAN_POINT('Ctrl Pts',(37.3125672988369,-30.7673014771556,10.));
#10115=CARTESIAN_POINT('Ctrl Pts',(37.2976643807312,-30.6729157024642,10.));
#10116=CARTESIAN_POINT('Ctrl Pts',(37.2878909459398,-30.5776880515643,10.));
#10117=CARTESIAN_POINT('Ctrl Pts',(37.2846130657184,-30.5457499622357,10.));
#10118=CARTESIAN_POINT('Ctrl Pts',(37.2819125883248,-30.5137172963057,10.));
#10119=CARTESIAN_POINT('Ctrl Pts',(37.2797877773691,-30.4816059493477,10.));
#10120=CARTESIAN_POINT('Ctrl Pts',(37.2785991601696,-30.4636428928259,10.));
#10121=CARTESIAN_POINT('Ctrl Pts',(37.2775906953478,-30.4456552201366,10.));
#10122=CARTESIAN_POINT('Ctrl Pts',(37.2767621583002,-30.4276457588107,10.));
#10123=CARTESIAN_POINT('Ctrl Pts',(37.2761878954323,-30.4151633176917,10.));
#10124=CARTESIAN_POINT('Ctrl Pts',(37.2757001840025,-30.402671938853,10.));
#10125=CARTESIAN_POINT('Ctrl Pts',(37.2752990741519,-30.3901820439812,10.));
#10126=CARTESIAN_POINT('Ctrl Pts',(37.2723062709527,-30.2969911206636,10.));
#10127=CARTESIAN_POINT('Ctrl Pts',(37.2741230598307,-30.2037357219583,10.));
#10128=CARTESIAN_POINT('Ctrl Pts',(37.2806103365498,-30.1107909830603,10.));
#10129=CARTESIAN_POINT('Ctrl Pts',(37.2871105716039,-30.0176605870496,10.));
#10130=CARTESIAN_POINT('Ctrl Pts',(37.2983003551911,-29.9248411115275,10.));
#10131=CARTESIAN_POINT('Ctrl Pts',(37.3140907933662,-29.832721945892,10.));
#10132=CARTESIAN_POINT('Ctrl Pts',(37.3296581165649,-29.7419044012272,10.));
#10133=CARTESIAN_POINT('Ctrl Pts',(37.3496974685084,-29.6517666687559,10.));
#10134=CARTESIAN_POINT('Ctrl Pts',(37.3741667173832,-29.5627070154397,10.));
#10135=CARTESIAN_POINT('Ctrl Pts',(37.3836803734301,-29.5280805782472,10.));
#10136=CARTESIAN_POINT('Ctrl Pts',(37.393864106677,-29.4936174486057,10.));
#10137=CARTESIAN_POINT('Ctrl Pts',(37.4047170075811,-29.4593424965086,10.));
#10138=CARTESIAN_POINT('Ctrl Pts',(37.4105212308036,-29.4410119621504,10.));
#10139=CARTESIAN_POINT('Ctrl Pts',(37.4165168636927,-29.4227352659255,10.));
#10140=CARTESIAN_POINT('Ctrl Pts',(37.4227038628238,-29.4045163264401,10.));
#10141=CARTESIAN_POINT('Ctrl Pts',(37.4281525019749,-29.3884716455105,10.));
#10142=CARTESIAN_POINT('Ctrl Pts',(37.433750036472,-29.3724706840406,10.));
#10143=CARTESIAN_POINT('Ctrl Pts',(37.4394903150468,-29.3565325286955,10.));
#10144=CARTESIAN_POINT('Ctrl Pts',(37.4719158315028,-29.266501546456,10.));
#10145=CARTESIAN_POINT('Ctrl Pts',(37.508932391867,-29.178349298418,10.));
#10146=CARTESIAN_POINT('Ctrl Pts',(37.5504669605507,-29.0925203605859,10.));
#10147=CARTESIAN_POINT('Ctrl Pts',(37.5816178870634,-29.0281486572119,10.));
#10148=CARTESIAN_POINT('Ctrl Pts',(37.6153113416024,-28.9650843527885,10.));
#10149=CARTESIAN_POINT('Ctrl Pts',(37.6515338806021,-28.9035321598138,10.));
#10150=CARTESIAN_POINT('Ctrl Pts',(37.6664656394419,-28.8781589384178,10.));
#10151=CARTESIAN_POINT('Ctrl Pts',(37.6818273228934,-28.8530428664222,10.));
#10152=CARTESIAN_POINT('Ctrl Pts',(37.6976186471279,-28.8281991892111,10.));
#10153=CARTESIAN_POINT('Ctrl Pts',(37.707051317448,-28.8133592547514,10.));
#10154=CARTESIAN_POINT('Ctrl Pts',(37.7166326076961,-28.7986239321154,10.));
#10155=CARTESIAN_POINT('Ctrl Pts',(37.7263604788376,-28.7839985432967,10.));
#10156=CARTESIAN_POINT('Ctrl Pts',(37.7738891331826,-28.7125414855586,10.));
#10157=CARTESIAN_POINT('Ctrl Pts',(37.8249265653207,-28.6436864116098,10.));
#10158=CARTESIAN_POINT('Ctrl Pts',(37.8794383922861,-28.5777860374312,10.));
#10159=CARTESIAN_POINT('Ctrl Pts',(37.9310245147155,-28.5154226025628,10.));
#10160=CARTESIAN_POINT('Ctrl Pts',(37.9857225827401,-28.4557049960579,10.));
#10161=CARTESIAN_POINT('Ctrl Pts',(38.0435272485066,-28.3989680111034,10.));
#10162=CARTESIAN_POINT('Ctrl Pts',(38.0564932251206,-28.3862415225005,10.));
#10163=CARTESIAN_POINT('Ctrl Pts',(38.0696155913077,-28.3736651582161,10.));
#10164=CARTESIAN_POINT('Ctrl Pts',(38.0828911169303,-28.3612402481786,10.));
#10165=CARTESIAN_POINT('Ctrl Pts',(-38.0865340033349,31.635987203375,10.));
#10166=CARTESIAN_POINT('Ctrl Pts',(-38.0249212302155,31.5780863258049,10.));
#10167=CARTESIAN_POINT('Ctrl Pts',(-37.9666796325226,31.517034936212,10.));
#10168=CARTESIAN_POINT('Ctrl Pts',(-37.9118060982863,31.4532178325339,10.));
#10169=CARTESIAN_POINT('Ctrl Pts',(-37.855479884161,31.387711283764,10.));
#10170=CARTESIAN_POINT('Ctrl Pts',(-37.802701985108,31.3192902159922,10.));
#10171=CARTESIAN_POINT('Ctrl Pts',(-37.7534945847852,31.2483222499473,10.));
#10172=CARTESIAN_POINT('Ctrl Pts',(-37.7025929329964,31.1749107981721,10.));
#10173=CARTESIAN_POINT('Ctrl Pts',(-37.6555113004629,31.0987735233447,10.));
#10174=CARTESIAN_POINT('Ctrl Pts',(-37.6123091713429,31.0202733477527,10.));
#10175=CARTESIAN_POINT('Ctrl Pts',(-37.5934082398529,30.9859295209312,10.));
#10176=CARTESIAN_POINT('Ctrl Pts',(-37.5752503635828,30.9511329138551,10.));
#10177=CARTESIAN_POINT('Ctrl Pts',(-37.5578429689868,30.915911828878,10.));
#10178=CARTESIAN_POINT('Ctrl Pts',(-37.5483347565091,30.8966734783134,10.));
#10179=CARTESIAN_POINT('Ctrl Pts',(-37.5390504796292,30.8773084638734,10.));
#10180=CARTESIAN_POINT('Ctrl Pts',(-37.5299915522756,30.8578212692062,10.));
#10181=CARTESIAN_POINT('Ctrl Pts',(-37.5213415858625,30.8392138146172,10.));
#10182=CARTESIAN_POINT('Ctrl Pts',(-37.5128945913309,30.8204889632415,10.));
#10183=CARTESIAN_POINT('Ctrl Pts',(-37.5046658996397,30.801683398448,10.));
#10184=CARTESIAN_POINT('Ctrl Pts',(-37.4681050714562,30.7181285577627,10.));
#10185=CARTESIAN_POINT('Ctrl Pts',(-37.4358044628107,30.6328902559792,10.));
#10186=CARTESIAN_POINT('Ctrl Pts',(-37.4077883457094,30.5463673398094,10.));
#10187=CARTESIAN_POINT('Ctrl Pts',(-37.3793099418999,30.4584167313599,10.));
#10188=CARTESIAN_POINT('Ctrl Pts',(-37.3552580988168,30.3691380088872,10.));
#10189=CARTESIAN_POINT('Ctrl Pts',(-37.3356974176737,30.2789129619801,10.));
#10190=CARTESIAN_POINT('Ctrl Pts',(-37.3164750142936,30.1902482455546,10.));
#10191=CARTESIAN_POINT('Ctrl Pts',(-37.3015895191302,30.1006687433848,10.));
#10192=CARTESIAN_POINT('Ctrl Pts',(-37.2911449398656,30.0105139328834,10.));
#10193=CARTESIAN_POINT('Ctrl Pts',(-37.287014788403,29.9748635717711,10.));
#10194=CARTESIAN_POINT('Ctrl Pts',(-37.2835795539213,29.9391230694737,10.));
#10195=CARTESIAN_POINT('Ctrl Pts',(-37.2808476966539,29.9033128824872,10.));
#10196=CARTESIAN_POINT('Ctrl Pts',(-37.2792307868413,29.8821178356521,10.));
#10197=CARTESIAN_POINT('Ctrl Pts',(-37.2778603014039,29.8608983733072,10.));
#10198=CARTESIAN_POINT('Ctrl Pts',(-37.2767381968828,29.8396587140598,10.));
#10199=CARTESIAN_POINT('Ctrl Pts',(-37.2759912880507,29.825520914251,10.));
#10200=CARTESIAN_POINT('Ctrl Pts',(-37.2753545077548,29.8113741694225,10.));
#10201=CARTESIAN_POINT('Ctrl Pts',(-37.2748287840665,29.79723427985,10.));
#10202=CARTESIAN_POINT('Ctrl Pts',(-37.2712900173062,29.7020554390877,10.));
#10203=CARTESIAN_POINT('Ctrl Pts',(-37.2727699852428,29.6070256281828,10.));
#10204=CARTESIAN_POINT('Ctrl Pts',(-37.2793273367095,29.5125435687522,10.));
#10205=CARTESIAN_POINT('Ctrl Pts',(-37.2858621977529,29.418385564165,10.));
#10206=CARTESIAN_POINT('Ctrl Pts',(-37.2974393139327,29.3247706066949,10.));
#10207=CARTESIAN_POINT('Ctrl Pts',(-37.3141647303328,29.2320754265285,10.));
#10208=CARTESIAN_POINT('Ctrl Pts',(-37.3161015946175,29.2213409862291,10.));
#10209=CARTESIAN_POINT('Ctrl Pts',(-37.3181075567504,29.2106188701492,10.));
#10210=CARTESIAN_POINT('Ctrl Pts',(-37.3201828266509,29.1999096568791,10.));
#10211=CARTESIAN_POINT('Ctrl Pts',(-37.33772774812,29.1093709246518,10.));
#10212=CARTESIAN_POINT('Ctrl Pts',(-37.360222053948,29.0197541127662,10.));
#10213=CARTESIAN_POINT('Ctrl Pts',(-37.3873904512652,28.9312971488731,10.));
#10214=CARTESIAN_POINT('Ctrl Pts',(-37.3981387282381,28.8963020795282,10.));
#10215=CARTESIAN_POINT('Ctrl Pts',(-37.4096191399982,28.8614885919146,10.));
#10216=CARTESIAN_POINT('Ctrl Pts',(-37.4218168347016,28.826871760633,10.));
#10217=CARTESIAN_POINT('Ctrl Pts',(-37.4277710430044,28.8099738279297,10.));
#10218=CARTESIAN_POINT('Ctrl Pts',(-37.4338961854739,28.7931227592818,10.));
#10219=CARTESIAN_POINT('Ctrl Pts',(-37.4401906356363,28.7763203362452,10.));
#10220=CARTESIAN_POINT('Ctrl Pts',(-37.4454353749813,28.7623200142288,10.));
#10221=CARTESIAN_POINT('Ctrl Pts',(-37.4507947656063,28.7483612736679,10.));
#10222=CARTESIAN_POINT('Ctrl Pts',(-37.4562655924271,28.7344496968282,10.));
#10223=CARTESIAN_POINT('Ctrl Pts',(-37.4904901961104,28.6474211324931,10.));
#10224=CARTESIAN_POINT('Ctrl Pts',(-37.5290932417427,28.5621806872409,10.));
#10225=CARTESIAN_POINT('Ctrl Pts',(-37.5717422429702,28.4789602337942,10.));
#10226=CARTESIAN_POINT('Ctrl Pts',(-37.6159714723182,28.3926563013224,10.));
#10227=CARTESIAN_POINT('Ctrl Pts',(-37.6645521622043,28.3085240970534,10.));
#10228=CARTESIAN_POINT('Ctrl Pts',(-37.7171694435466,28.2268257622467,10.));
#10229=CARTESIAN_POINT('Ctrl Pts',(-37.770364364078,28.1442305327571,10.));
#10230=CARTESIAN_POINT('Ctrl Pts',(-37.8276854092032,28.0641220869244,10.));
#10231=CARTESIAN_POINT('Ctrl Pts',(-37.8888588427698,27.9867866516892,10.));
#10232=CARTESIAN_POINT('Ctrl Pts',(-37.9126758941047,27.9566771429758,10.));
#10233=CARTESIAN_POINT('Ctrl Pts',(-37.9370774163132,27.9269882051562,10.));
#10234=CARTESIAN_POINT('Ctrl Pts',(-37.9620491203782,27.8977377702384,10.));
#10235=CARTESIAN_POINT('Ctrl Pts',(-37.982034894532,27.8743275702518,10.));
#10236=CARTESIAN_POINT('Ctrl Pts',(-38.0023859127899,27.8511982591558,10.));
#10237=CARTESIAN_POINT('Ctrl Pts',(-38.0230952862197,27.8283593716466,10.));
#10238=CARTESIAN_POINT('Ctrl Pts',(-38.0346445261292,27.8156225405686,10.));
#10239=CARTESIAN_POINT('Ctrl Pts',(-38.0463001486068,27.8029816946559,10.));
#10240=CARTESIAN_POINT('Ctrl Pts',(-38.0580558973667,27.7904432603858,10.));
#10241=CARTESIAN_POINT('Ctrl Pts',(-38.1271112801678,27.716790242111,10.));
#10242=CARTESIAN_POINT('Ctrl Pts',(-38.1996672523087,27.6466146571222,10.));
#10243=CARTESIAN_POINT('Ctrl Pts',(-38.2754118739757,27.5802053578348,10.));
#10244=CARTESIAN_POINT('Ctrl Pts',(-38.3396628308816,27.5238731598152,10.));
#10245=CARTESIAN_POINT('Ctrl Pts',(-38.4062092138265,27.470250936803,10.));
#10246=CARTESIAN_POINT('Ctrl Pts',(-38.4748854868873,27.419529916892,10.));
#10247=CARTESIAN_POINT('Ctrl Pts',(-38.4975744224142,27.4027729512132,10.));
#10248=CARTESIAN_POINT('Ctrl Pts',(-38.5204959977952,27.3863327822983,10.));
#10249=CARTESIAN_POINT('Ctrl Pts',(-38.5436447147886,27.3702167463987,10.));
#10250=CARTESIAN_POINT('Ctrl Pts',(-38.5602398136962,27.3586633108528,10.));
#10251=CARTESIAN_POINT('Ctrl Pts',(-38.5769526172639,27.3472759337365,10.));
#10252=CARTESIAN_POINT('Ctrl Pts',(-38.5937665384207,27.3360668068749,10.));
#10253=CARTESIAN_POINT('Ctrl Pts',(-38.6801204221607,27.2784983415061,10.));
#10254=CARTESIAN_POINT('Ctrl Pts',(-38.7692236972918,27.2255681352496,10.));
#10255=CARTESIAN_POINT('Ctrl Pts',(-38.8607678183074,27.1775976530154,10.));
#10256=CARTESIAN_POINT('Ctrl Pts',(-38.952311939323,27.1296271707811,10.));
#10257=CARTESIAN_POINT('Ctrl Pts',(-39.0462975515555,27.0866155018757,10.));
#10258=CARTESIAN_POINT('Ctrl Pts',(-39.1424541530616,27.0489248578152,10.));
#10259=CARTESIAN_POINT('Ctrl Pts',(-39.1630221217565,27.0408628009727,10.));
#10260=CARTESIAN_POINT('Ctrl Pts',(-39.1836895389297,27.0330443769238,10.));
#10261=CARTESIAN_POINT('Ctrl Pts',(-39.2044525003272,27.0254684088901,10.));
#10262=CARTESIAN_POINT('Ctrl Pts',(-40.7937992825329,27.0307770462543,10.));
#10263=CARTESIAN_POINT('Ctrl Pts',(-40.8868534224289,27.0648166662984,10.));
#10264=CARTESIAN_POINT('Ctrl Pts',(-40.9778403384339,27.1036257277316,10.));
#10265=CARTESIAN_POINT('Ctrl Pts',(-41.0665522485249,27.1468755032666,10.));
#10266=CARTESIAN_POINT('Ctrl Pts',(-41.1572339280192,27.1910856017668,10.));
#10267=CARTESIAN_POINT('Ctrl Pts',(-41.2455391179634,27.2399364251585,10.));
#10268=CARTESIAN_POINT('Ctrl Pts',(-41.3312169493438,27.2931224121673,10.));
#10269=CARTESIAN_POINT('Ctrl Pts',(-41.414166339304,27.3446146722506,10.));
#10270=CARTESIAN_POINT('Ctrl Pts',(-41.4946533698995,27.4001712453837,10.));
#10271=CARTESIAN_POINT('Ctrl Pts',(-41.5724166737304,27.459545531637,10.));
#10272=CARTESIAN_POINT('Ctrl Pts',(-41.6404595645825,27.5114980321086,10.));
#10273=CARTESIAN_POINT('Ctrl Pts',(-41.7064168053658,27.5663741861413,10.));
#10274=CARTESIAN_POINT('Ctrl Pts',(-41.7700880360598,27.6240217668293,10.));
#10275=CARTESIAN_POINT('Ctrl Pts',(-41.7834305900767,27.6361020415607,10.));
#10276=CARTESIAN_POINT('Ctrl Pts',(-41.7966745289852,27.6483059196791,10.));
#10277=CARTESIAN_POINT('Ctrl Pts',(-41.8098008297905,27.6606156964746,10.));
#10278=CARTESIAN_POINT('Ctrl Pts',(-41.8822284325512,27.7285379265867,10.));
#10279=CARTESIAN_POINT('Ctrl Pts',(-41.9511903175657,27.7997813678814,10.));
#10280=CARTESIAN_POINT('Ctrl Pts',(-42.0164471409414,27.8740548505011,10.));
#10281=CARTESIAN_POINT('Ctrl Pts',(-42.0813426208374,27.947917062126,10.));
#10282=CARTESIAN_POINT('Ctrl Pts',(-42.1425744423444,28.0247766498528,10.));
#10283=CARTESIAN_POINT('Ctrl Pts',(-42.1998636016162,28.1043739992373,10.));
#10284=CARTESIAN_POINT('Ctrl Pts',(-42.2557187057104,28.1819788775774,10.));
#10285=CARTESIAN_POINT('Ctrl Pts',(-42.3078263315155,28.2621869103881,10.));
#10286=CARTESIAN_POINT('Ctrl Pts',(-42.3558810447646,28.3447716158106,10.));
#10287=CARTESIAN_POINT('Ctrl Pts',(-42.3766086283242,28.3803931244337,10.));
#10288=CARTESIAN_POINT('Ctrl Pts',(-42.3965815502584,28.4164569256333,10.));
#10289=CARTESIAN_POINT('Ctrl Pts',(-42.4157723168559,28.4529451771185,10.));
#10290=CARTESIAN_POINT('Ctrl Pts',(-42.4294376380156,28.4789276553363,10.));
#10291=CARTESIAN_POINT('Ctrl Pts',(-42.4427063253691,28.5051253564734,10.));
#10292=CARTESIAN_POINT('Ctrl Pts',(-42.4555678554338,28.5315318420532,10.));
#10293=CARTESIAN_POINT('Ctrl Pts',(-42.4611833404534,28.5430612031361,10.));
#10294=CARTESIAN_POINT('Ctrl Pts',(-42.4667202817154,28.554628567478,10.));
#10295=CARTESIAN_POINT('Ctrl Pts',(-42.4721741089808,28.5662251224027,10.));
#10296=CARTESIAN_POINT('Ctrl Pts',(-42.512401961449,28.6517622100199,10.));
#10297=CARTESIAN_POINT('Ctrl Pts',(-42.54817377646,28.7390124376936,10.));
#10298=CARTESIAN_POINT('Ctrl Pts',(-42.5792385749088,28.8277384868494,10.));
#10299=CARTESIAN_POINT('Ctrl Pts',(-42.6096166633377,28.9145031819959,10.));
#10300=CARTESIAN_POINT('Ctrl Pts',(-42.6354937565339,29.0026798461803,10.));
#10301=CARTESIAN_POINT('Ctrl Pts',(-42.6565860361294,29.0920553698958,10.));
#10302=CARTESIAN_POINT('Ctrl Pts',(-42.6603147481206,29.1078552546589,10.));
#10303=CARTESIAN_POINT('Ctrl Pts',(-42.6638937963736,29.1236926137693,10.));
#10304=CARTESIAN_POINT('Ctrl Pts',(-42.6673214406689,29.1395662754716,10.));
#10305=CARTESIAN_POINT('Ctrl Pts',(-42.6874323400132,29.232701264176,10.));
#10306=CARTESIAN_POINT('Ctrl Pts',(-42.7023352690137,29.3270870046807,10.));
#10307=CARTESIAN_POINT('Ctrl Pts',(-42.7121087193039,29.4223145987471,10.));
#10308=CARTESIAN_POINT('Ctrl Pts',(-42.7153866067918,29.4542526891688,10.));
#10309=CARTESIAN_POINT('Ctrl Pts',(-42.7180870912415,29.4862853537632,10.));
#10310=CARTESIAN_POINT('Ctrl Pts',(-42.7202119090113,29.5183966971079,10.));
#10311=CARTESIAN_POINT('Ctrl Pts',(-42.7214005292254,29.5363597395597,10.));
#10312=CARTESIAN_POINT('Ctrl Pts',(-42.7224089972278,29.5543473974331,10.));
#10313=CARTESIAN_POINT('Ctrl Pts',(-42.7232375376159,29.5723568432295,10.));
#10314=CARTESIAN_POINT('Ctrl Pts',(-42.7238118031779,29.5848392818196,10.));
#10315=CARTESIAN_POINT('Ctrl Pts',(-42.7242995172634,29.5973306577781,10.));
#10316=CARTESIAN_POINT('Ctrl Pts',(-42.7247006297286,29.609820549451,10.));
#10317=CARTESIAN_POINT('Ctrl Pts',(-42.7276934506505,29.7030113932964,10.));
#10318=CARTESIAN_POINT('Ctrl Pts',(-42.7258766829749,29.7962666945407,10.));
#10319=CARTESIAN_POINT('Ctrl Pts',(-42.7193894300159,29.8892113227638,10.));
#10320=CARTESIAN_POINT('Ctrl Pts',(-42.7128892185463,29.9823416110736,10.));
#10321=CARTESIAN_POINT('Ctrl Pts',(-42.701699460792,30.0751609655971,10.));
#10322=CARTESIAN_POINT('Ctrl Pts',(-42.6859090498045,30.1672800015875,10.));
#10323=CARTESIAN_POINT('Ctrl Pts',(-42.6703417487034,30.2580974458921,10.));
#10324=CARTESIAN_POINT('Ctrl Pts',(-42.6503024174743,30.3482350691811,10.));
#10325=CARTESIAN_POINT('Ctrl Pts',(-42.6258331870985,30.4372946086112,10.));
#10326=CARTESIAN_POINT('Ctrl Pts',(-42.6163195250727,30.4719210494636,10.));
#10327=CARTESIAN_POINT('Ctrl Pts',(-42.606135783656,30.5063841816026,10.));
#10328=CARTESIAN_POINT('Ctrl Pts',(-42.5952828723427,30.5406591351763,10.));
#10329=CARTESIAN_POINT('Ctrl Pts',(-42.5894786544185,30.5589896360104,10.));
#10330=CARTESIAN_POINT('Ctrl Pts',(-42.5834830269037,30.5772662986208,10.));
#10331=CARTESIAN_POINT('Ctrl Pts',(-42.5772960332143,30.5954852044445,10.));
#10332=CARTESIAN_POINT('Ctrl Pts',(-42.5718474280992,30.6115297696157,10.));
#10333=CARTESIAN_POINT('Ctrl Pts',(-42.5662499293154,30.6275306156841,10.));
#10334=CARTESIAN_POINT('Ctrl Pts',(-42.5605096880314,30.6434686563279,10.));
#10335=CARTESIAN_POINT('Ctrl Pts',(-42.5280842026754,30.7334994891673,10.));
#10336=CARTESIAN_POINT('Ctrl Pts',(-42.4910676731712,30.8216515881688,10.));
#10337=CARTESIAN_POINT('Ctrl Pts',(-42.4495331341105,30.9074803825421,10.));
#10338=CARTESIAN_POINT('Ctrl Pts',(-42.418382229815,30.9718519783221,10.));
#10339=CARTESIAN_POINT('Ctrl Pts',(-42.3846887967975,31.0349161782887,10.));
#10340=CARTESIAN_POINT('Ctrl Pts',(-42.3484662781896,31.0964682722131,10.));
#10341=CARTESIAN_POINT('Ctrl Pts',(-42.3335345030887,31.1218414946943,10.));
#10342=CARTESIAN_POINT('Ctrl Pts',(-42.3181728017638,31.1469575678454,10.));
#10343=CARTESIAN_POINT('Ctrl Pts',(-42.3023814580131,31.1718012463697,10.));
#10344=CARTESIAN_POINT('Ctrl Pts',(-42.2929488091092,31.1866411295805,10.));
#10345=CARTESIAN_POINT('Ctrl Pts',(-42.2833675408082,31.2013764016503,9.99999999999999));
#10346=CARTESIAN_POINT('Ctrl Pts',(-42.2736396920405,31.2160017407882,9.99999999999999));
#10347=CARTESIAN_POINT('Ctrl Pts',(-42.2261110200766,31.2874587466322,9.99999999999999));
#10348=CARTESIAN_POINT('Ctrl Pts',(-42.1750735624793,31.3563137747452,10.));
#10349=CARTESIAN_POINT('Ctrl Pts',(-42.1205617015116,31.4222141122843,10.));
#10350=CARTESIAN_POINT('Ctrl Pts',(-42.0689756436836,31.4845773954821,10.));
#10351=CARTESIAN_POINT('Ctrl Pts',(-42.0142776442785,31.5442948684644,9.99999999999999));
#10352=CARTESIAN_POINT('Ctrl Pts',(-41.9564730504323,31.6010317426951,9.99999999999999));
#10353=CARTESIAN_POINT('Ctrl Pts',(-41.9435070760097,31.6137582201452,9.99999999999999));
#10354=CARTESIAN_POINT('Ctrl Pts',(-41.9303847118439,31.6263345741028,9.99999999999999));
#10355=CARTESIAN_POINT('Ctrl Pts',(-41.9171091880767,31.6387594746126,9.99999999999999));
#10356=CARTESIAN_POINT('Ctrl Pts',(41.9134659966651,31.6359872033749,10.));
#10357=CARTESIAN_POINT('Ctrl Pts',(41.9750786368702,31.5780864507117,10.));
#10358=CARTESIAN_POINT('Ctrl Pts',(42.0333200948858,31.5170351770757,10.));
#10359=CARTESIAN_POINT('Ctrl Pts',(42.0881934870624,31.4532181824915,10.));
#10360=CARTESIAN_POINT('Ctrl Pts',(42.1445195700427,31.3877117286362,10.));
#10361=CARTESIAN_POINT('Ctrl Pts',(42.1972973335829,31.3192907470308,10.));
#10362=CARTESIAN_POINT('Ctrl Pts',(42.2465045986483,31.2483228609998,10.));
#10363=CARTESIAN_POINT('Ctrl Pts',(42.2974062316616,31.1749113172842,10.));
#10364=CARTESIAN_POINT('Ctrl Pts',(42.344487827514,31.0987739309724,10.));
#10365=CARTESIAN_POINT('Ctrl Pts',(42.3876899067312,31.0202736297946,10.));
#10366=CARTESIAN_POINT('Ctrl Pts',(42.4065908163888,30.9859297480294,10.));
#10367=CARTESIAN_POINT('Ctrl Pts',(42.4247486682925,30.951133083306,10.));
#10368=CARTESIAN_POINT('Ctrl Pts',(42.4421560363682,30.9159119384179,10.));
#10369=CARTESIAN_POINT('Ctrl Pts',(42.4516643000981,30.8966734221178,10.));
#10370=CARTESIAN_POINT('Ctrl Pts',(42.4609486244912,30.8773082395153,10.));
#10371=CARTESIAN_POINT('Ctrl Pts',(42.4700075956502,30.8578208744221,10.));
#10372=CARTESIAN_POINT('Ctrl Pts',(42.4786576094824,30.8392132450731,10.));
#10373=CARTESIAN_POINT('Ctrl Pts',(42.4871046478346,30.8204882165881,10.));
#10374=CARTESIAN_POINT('Ctrl Pts',(42.4953333795948,30.8016824730484,10.));
#10375=CARTESIAN_POINT('Ctrl Pts',(42.5318940411399,30.7181276258749,10.));
#10376=CARTESIAN_POINT('Ctrl Pts',(42.5641944897046,30.6328893164368,10.));
#10377=CARTESIAN_POINT('Ctrl Pts',(42.5922104581374,30.5463663947005,10.));
#10378=CARTESIAN_POINT('Ctrl Pts',(42.6206887314238,30.458415716977,10.));
#10379=CARTESIAN_POINT('Ctrl Pts',(42.6447404493657,30.3691369254667,10.));
#10380=CARTESIAN_POINT('Ctrl Pts',(42.6643010157385,30.2789118139978,10.));
#10381=CARTESIAN_POINT('Ctrl Pts',(42.6835233268679,30.1902469394079,10.));
#10382=CARTESIAN_POINT('Ctrl Pts',(42.698408730528,30.1006672814378,10.));
#10383=CARTESIAN_POINT('Ctrl Pts',(42.7088532234977,30.0105123225977,10.));
#10384=CARTESIAN_POINT('Ctrl Pts',(42.7129833484531,29.9748618370792,10.));
#10385=CARTESIAN_POINT('Ctrl Pts',(42.7164185546788,29.9391212112098,10.));
#10386=CARTESIAN_POINT('Ctrl Pts',(42.7191503821694,29.9033109019147,10.));
#10387=CARTESIAN_POINT('Ctrl Pts',(42.7207672703654,29.8821158350244,10.));
#10388=CARTESIAN_POINT('Ctrl Pts',(42.7221377348703,29.8608963531876,10.));
#10389=CARTESIAN_POINT('Ctrl Pts',(42.7232598192034,29.8396566750697,10.));
#10390=CARTESIAN_POINT('Ctrl Pts',(42.7240067154734,29.8255188461256,10.));
#10391=CARTESIAN_POINT('Ctrl Pts',(42.7246434832814,29.8113720723697,10.));
#10392=CARTESIAN_POINT('Ctrl Pts',(42.7251691945808,29.7972321541886,10.));
#10393=CARTESIAN_POINT('Ctrl Pts',(42.7287078734581,29.7020532416424,10.));
#10394=CARTESIAN_POINT('Ctrl Pts',(42.7272278347504,29.6070233725301,10.));
#10395=CARTESIAN_POINT('Ctrl Pts',(42.7206704346253,29.5125412731866,10.));
#10396=CARTESIAN_POINT('Ctrl Pts',(42.7141355191106,29.4183831426661,10.));
#10397=CARTESIAN_POINT('Ctrl Pts',(42.7025583611906,29.3247680784185,10.));
#10398=CARTESIAN_POINT('Ctrl Pts',(42.6858329205046,29.2320728163631,10.));
#10399=CARTESIAN_POINT('Ctrl Pts',(42.6838960555975,29.2213383787185,10.));
#10400=CARTESIAN_POINT('Ctrl Pts',(42.6818900932326,29.2106162655995,10.));
#10401=CARTESIAN_POINT('Ctrl Pts',(42.6798148234985,29.1999070556032,10.));
#10402=CARTESIAN_POINT('Ctrl Pts',(42.6622698775574,29.1093682175089,10.));
#10403=CARTESIAN_POINT('Ctrl Pts',(42.6397755611135,29.0197513248276,10.));
#10404=CARTESIAN_POINT('Ctrl Pts',(42.6126071639148,28.931294302045,10.));
#10405=CARTESIAN_POINT('Ctrl Pts',(42.6018588686328,28.8962991496375,10.));
#10406=CARTESIAN_POINT('Ctrl Pts',(42.5903784377438,28.861485583013,10.));
#10407=CARTESIAN_POINT('Ctrl Pts',(42.5781807229744,28.8268686766644,10.));
#10408=CARTESIAN_POINT('Ctrl Pts',(42.5722259508754,28.8099691350719,10.));
#10409=CARTESIAN_POINT('Ctrl Pts',(42.5661002125772,28.7931164671958,10.));
#10410=CARTESIAN_POINT('Ctrl Pts',(42.5598051349902,28.7763124550784,10.));
#10411=CARTESIAN_POINT('Ctrl Pts',(42.5545609327821,28.7623136383469,10.));
#10412=CARTESIAN_POINT('Ctrl Pts',(42.5492021060364,28.7483563994138,10.));
#10413=CARTESIAN_POINT('Ctrl Pts',(42.543731866508,28.7344463125978,10.));
#10414=CARTESIAN_POINT('Ctrl Pts',(42.5095072459392,28.6474176841639,10.));
#10415=CARTESIAN_POINT('Ctrl Pts',(42.4709041883668,28.5621771974268,10.));
#10416=CARTESIAN_POINT('Ctrl Pts',(42.4282551773101,28.4789567220783,10.));
#10417=CARTESIAN_POINT('Ctrl Pts',(42.384025973209,28.3926528360469,10.));
#10418=CARTESIAN_POINT('Ctrl Pts',(42.33544531781,28.3085206957999,10.));
#10419=CARTESIAN_POINT('Ctrl Pts',(42.2828280762731,28.2268224389197,10.));
#10420=CARTESIAN_POINT('Ctrl Pts',(42.2296332219524,28.144227328533,10.));
#10421=CARTESIAN_POINT('Ctrl Pts',(42.172312252504,28.0641190135926,10.));
#10422=CARTESIAN_POINT('Ctrl Pts',(42.111138899714,27.9867837170881,10.));
#10423=CARTESIAN_POINT('Ctrl Pts',(42.0873215657202,27.9566738652924,10.));
#10424=CARTESIAN_POINT('Ctrl Pts',(42.0629197462126,27.9269845966725,10.));
#10425=CARTESIAN_POINT('Ctrl Pts',(42.0379477305135,27.8977338437241,10.));
#10426=CARTESIAN_POINT('Ctrl Pts',(42.0179551026749,27.8743156533487,10.));
#10427=CARTESIAN_POINT('Ctrl Pts',(41.9975969801375,27.8511785456982,10.));
#10428=CARTESIAN_POINT('Ctrl Pts',(41.9768802587376,27.8283320652486,10.));
#10429=CARTESIAN_POINT('Ctrl Pts',(41.9653377723937,27.8156029666857,10.));
#10430=CARTESIAN_POINT('Ctrl Pts',(41.9536890484812,27.802969758936,10.));
#10431=CARTESIAN_POINT('Ctrl Pts',(41.9419403107313,27.7904388332169,10.));
#10432=CARTESIAN_POINT('Ctrl Pts',(41.8728849423382,27.7167860110788,10.));
#10433=CARTESIAN_POINT('Ctrl Pts',(41.8003289871598,27.6466106302074,10.));
#10434=CARTESIAN_POINT('Ctrl Pts',(41.7245843802806,27.580201539271,10.));
#10435=CARTESIAN_POINT('Ctrl Pts',(41.6603337326078,27.5238697781091,10.));
#10436=CARTESIAN_POINT('Ctrl Pts',(41.5937876785201,27.4702479699947,10.));
#10437=CARTESIAN_POINT('Ctrl Pts',(41.5251117488698,27.419527338206,10.));
#10438=CARTESIAN_POINT('Ctrl Pts',(41.5024197920256,27.4027681855666,10.));
#10439=CARTESIAN_POINT('Ctrl Pts',(41.4794951326352,27.3863259143062,10.));
#10440=CARTESIAN_POINT('Ctrl Pts',(41.4563432710306,27.3702078635546,10.));
#10441=CARTESIAN_POINT('Ctrl Pts',(41.439752008952,27.3586572241813,10.));
#10442=CARTESIAN_POINT('Ctrl Pts',(41.4230430998386,27.3472725679575,10.));
#10443=CARTESIAN_POINT('Ctrl Pts',(41.4062331203527,27.3360660788018,10.));
#10444=CARTESIAN_POINT('Ctrl Pts',(41.3198794116228,27.278497781277,10.));
#10445=CARTESIAN_POINT('Ctrl Pts',(41.2307763052375,27.2255677270881,10.));
#10446=CARTESIAN_POINT('Ctrl Pts',(41.1392323413556,27.177597375897,10.));
#10447=CARTESIAN_POINT('Ctrl Pts',(41.0476883774738,27.1296270247058,10.));
#10448=CARTESIAN_POINT('Ctrl Pts',(40.9537029107743,27.0866154658313,10.));
#10449=CARTESIAN_POINT('Ctrl Pts',(40.8575464379022,27.0489249053832,10.));
#10450=CARTESIAN_POINT('Ctrl Pts',(40.8369784825986,27.0408628608893,10.));
#10451=CARTESIAN_POINT('Ctrl Pts',(40.8163110779066,27.0330444483139,10.));
#10452=CARTESIAN_POINT('Ctrl Pts',(40.7955481281091,27.0254684909089,10.));
#10453=CARTESIAN_POINT('Ctrl Pts',(39.2062007174671,27.0307770462543,10.));
#10454=CARTESIAN_POINT('Ctrl Pts',(39.1131465233113,27.0648166861469,10.));
#10455=CARTESIAN_POINT('Ctrl Pts',(39.0221595534034,27.1036257598841,10.));
#10456=CARTESIAN_POINT('Ctrl Pts',(38.9334475905781,27.1468755422436,10.));
#10457=CARTESIAN_POINT('Ctrl Pts',(38.8427658845523,27.1910856343743,10.));
#10458=CARTESIAN_POINT('Ctrl Pts',(38.754460667862,27.2399364428682,10.));
#10459=CARTESIAN_POINT('Ctrl Pts',(38.6687828102117,27.2931224089196,10.));
#10460=CARTESIAN_POINT('Ctrl Pts',(38.5858334272673,27.3446146285694,10.));
#10461=CARTESIAN_POINT('Ctrl Pts',(38.5053464022086,27.4001711524073,10.));
#10462=CARTESIAN_POINT('Ctrl Pts',(38.427583102789,27.4595453830244,10.));
#10463=CARTESIAN_POINT('Ctrl Pts',(38.3595402157968,27.5114978348144,10.));
#10464=CARTESIAN_POINT('Ctrl Pts',(38.2935829780114,27.5663739353082,10.));
#10465=CARTESIAN_POINT('Ctrl Pts',(38.229911749687,27.6240214592988,10.));
#10466=CARTESIAN_POINT('Ctrl Pts',(38.2165692334771,27.6361016883684,10.));
#10467=CARTESIAN_POINT('Ctrl Pts',(38.2033253318375,27.6483055199554,10.));
#10468=CARTESIAN_POINT('Ctrl Pts',(38.1901990676262,27.6606152495089,10.));
#10469=CARTESIAN_POINT('Ctrl Pts',(38.1177714560464,27.7285374165783,10.));
#10470=CARTESIAN_POINT('Ctrl Pts',(38.0488095620059,27.7997807923481,10.));
#10471=CARTESIAN_POINT('Ctrl Pts',(37.983552729848,27.8740542095836,10.));
#10472=CARTESIAN_POINT('Ctrl Pts',(37.9186572520394,27.9479163438703,10.));
#10473=CARTESIAN_POINT('Ctrl Pts',(37.8574254316395,28.0247758533942,10.));
#10474=CARTESIAN_POINT('Ctrl Pts',(37.8001362727997,28.1043731264343,10.));
#10475=CARTESIAN_POINT('Ctrl Pts',(37.7442811597055,28.181977943431,10.));
#10476=CARTESIAN_POINT('Ctrl Pts',(37.6921735255212,28.2621859175384,10.));
#10477=CARTESIAN_POINT('Ctrl Pts',(37.6441188049395,28.3447705693782,10.));
#10478=CARTESIAN_POINT('Ctrl Pts',(37.6233912222305,28.3803920479923,10.));
#10479=CARTESIAN_POINT('Ctrl Pts',(37.6034183010496,28.4164558199656,10.));
#10480=CARTESIAN_POINT('Ctrl Pts',(37.5842275351277,28.4529440432242,10.));
#10481=CARTESIAN_POINT('Ctrl Pts',(37.5705622652714,28.4789264047118,10.));
#10482=CARTESIAN_POINT('Ctrl Pts',(37.557293626232,28.505123988025,10.));
#10483=CARTESIAN_POINT('Ctrl Pts',(37.5444321413805,28.5315303548389,10.));
#10484=CARTESIAN_POINT('Ctrl Pts',(37.5388166779207,28.5430596603322,10.));
#10485=CARTESIAN_POINT('Ctrl Pts',(37.5332797574667,28.5546269691094,10.));
#10486=CARTESIAN_POINT('Ctrl Pts',(37.5278259503489,28.5662234683187,10.));
#10487=CARTESIAN_POINT('Ctrl Pts',(37.4875980830446,28.6517604925136,10.));
#10488=CARTESIAN_POINT('Ctrl Pts',(37.4518262526605,28.7390106640601,10.));
#10489=CARTESIAN_POINT('Ctrl Pts',(37.4207614384841,28.8277366668812,10.));
#10490=CARTESIAN_POINT('Ctrl Pts',(37.3903833336519,28.9145013196402,10.));
#10491=CARTESIAN_POINT('Ctrl Pts',(37.3645062240159,29.0026779508926,10.));
#10492=CARTESIAN_POINT('Ctrl Pts',(37.3434139281184,29.092053453568,10.));
#10493=CARTESIAN_POINT('Ctrl Pts',(37.3396851656113,29.1078535364538,10.));
#10494=CARTESIAN_POINT('Ctrl Pts',(37.3361060706703,29.1236910950166,10.));
#10495=CARTESIAN_POINT('Ctrl Pts',(37.3326783835832,29.1395649574699,10.));
#10496=CARTESIAN_POINT('Ctrl Pts',(37.3125674868137,29.2326999493804,10.));
#10497=CARTESIAN_POINT('Ctrl Pts',(37.2976645630368,29.3270857062678,10.));
#10498=CARTESIAN_POINT('Ctrl Pts',(37.2878911201781,29.4223133275768,10.));
#10499=CARTESIAN_POINT('Ctrl Pts',(37.2846132361742,29.4542514174737,10.));
#10500=CARTESIAN_POINT('Ctrl Pts',(37.2819127551077,29.4862840827079,10.));
#10501=CARTESIAN_POINT('Ctrl Pts',(37.2797879406052,29.5183954277846,10.));
#10502=CARTESIAN_POINT('Ctrl Pts',(37.2785993218355,29.5363584769983,10.));
#10503=CARTESIAN_POINT('Ctrl Pts',(37.2775908553575,29.5543461419914,10.));
#10504=CARTESIAN_POINT('Ctrl Pts',(37.2767623165709,29.5723555952498,10.));
#10505=CARTESIAN_POINT('Ctrl Pts',(37.2761880522997,29.584838035077,10.));
#10506=CARTESIAN_POINT('Ctrl Pts',(37.2757003394872,29.5973294124411,10.));
#10507=CARTESIAN_POINT('Ctrl Pts',(37.2752992282755,29.6098193056725,10.));
#10508=CARTESIAN_POINT('Ctrl Pts',(37.2723064158566,29.7030101876157,10.));
#10509=CARTESIAN_POINT('Ctrl Pts',(37.2741231937037,29.7962655355841,10.));
#10510=CARTESIAN_POINT('Ctrl Pts',(37.2806104580608,29.889210216868,10.));
#10511=CARTESIAN_POINT('Ctrl Pts',(37.2871106808443,29.9823405568134,10.));
#10512=CARTESIAN_POINT('Ctrl Pts',(37.2983004509909,30.0751599693494,10.));
#10513=CARTESIAN_POINT('Ctrl Pts',(37.3140908750205,30.1672790674991,10.));
#10514=CARTESIAN_POINT('Ctrl Pts',(37.3296581867233,30.258096559923,10.));
#10515=CARTESIAN_POINT('Ctrl Pts',(37.3496975278913,30.3482342355622,10.));
#10516=CARTESIAN_POINT('Ctrl Pts',(37.3741667671441,30.4372938295988,10.));
#10517=CARTESIAN_POINT('Ctrl Pts',(37.3836804263222,30.4719202687557,10.));
#10518=CARTESIAN_POINT('Ctrl Pts',(37.3938641638431,30.5063833997562,10.));
#10519=CARTESIAN_POINT('Ctrl Pts',(37.4047170701892,30.5406583526803,10.));
#10520=CARTESIAN_POINT('Ctrl Pts',(37.4105212906447,30.5589888695513,10.));
#10521=CARTESIAN_POINT('Ctrl Pts',(37.4165169207267,30.5772655482422,10.));
#10522=CARTESIAN_POINT('Ctrl Pts',(37.4227039170148,30.5954844701692,10.));
#10523=CARTESIAN_POINT('Ctrl Pts',(37.4281525384222,30.6115290907587,10.));
#10524=CARTESIAN_POINT('Ctrl Pts',(37.4337500543009,30.6275299920748,10.));
#10525=CARTESIAN_POINT('Ctrl Pts',(37.4394903134347,30.6434680876312,10.));
#10526=CARTESIAN_POINT('Ctrl Pts',(37.4719158137031,30.7334989921067,10.));
#10527=CARTESIAN_POINT('Ctrl Pts',(37.5089323580049,30.8216511625714,10.));
#10528=CARTESIAN_POINT('Ctrl Pts',(37.5504669112701,30.9074800257348,10.));
#10529=CARTESIAN_POINT('Ctrl Pts',(37.5816178262191,30.9718516731074,10.));
#10530=CARTESIAN_POINT('Ctrl Pts',(37.6153112695565,31.0349159231632,10.));
#10531=CARTESIAN_POINT('Ctrl Pts',(37.6515337979429,31.0964680645853,10.));
#10532=CARTESIAN_POINT('Ctrl Pts',(37.6664655652351,31.1218412865275,10.));
#10533=CARTESIAN_POINT('Ctrl Pts',(37.6818272579777,31.1469573591066,10.));
#10534=CARTESIAN_POINT('Ctrl Pts',(37.6976185923575,31.1718010369838,10.));
#10535=CARTESIAN_POINT('Ctrl Pts',(37.7070512515414,31.1866409447872,10.));
#10536=CARTESIAN_POINT('Ctrl Pts',(37.7166325303773,31.2013762411221,10.));
#10537=CARTESIAN_POINT('Ctrl Pts',(37.7263603898849,31.2160016041003,10.));
#10538=CARTESIAN_POINT('Ctrl Pts',(37.7738890534039,31.2874586348368,10.));
#10539=CARTESIAN_POINT('Ctrl Pts',(37.8249264987974,31.3563136849385,10.));
#10540=CARTESIAN_POINT('Ctrl Pts',(37.8794383434655,31.4222140400578,10.));
#10541=CARTESIAN_POINT('Ctrl Pts',(37.9310244322697,31.4845773959873,10.));
#10542=CARTESIAN_POINT('Ctrl Pts',(37.9857224645776,31.5442949330007,10.));
#10543=CARTESIAN_POINT('Ctrl Pts',(38.0435270929093,31.6010318603323,10.));
#10544=CARTESIAN_POINT('Ctrl Pts',(38.0564930683829,31.6137583431323,10.));
#10545=CARTESIAN_POINT('Ctrl Pts',(38.069615433518,31.6263347020438,10.));
#10546=CARTESIAN_POINT('Ctrl Pts',(38.082890958175,31.6387596071244,10.));
#10547=CARTESIAN_POINT('Origin',(40.,-30.,12.2084234471775));
#10548=CARTESIAN_POINT('Ctrl Pts',(36.9237142109313,-29.9977821171135,9.70842344717746));
#10549=CARTESIAN_POINT('Ctrl Pts',(36.922516886621,-29.8529950058616,9.70090492237387));
#10550=CARTESIAN_POINT('Ctrl Pts',(36.9976394341993,-28.6901609317351,9.64045815782839));
#10551=CARTESIAN_POINT('Ctrl Pts',(38.4808974147036,-26.6996618505134,9.52708315354101));
#10552=CARTESIAN_POINT('Ctrl Pts',(41.9490299734334,-26.9342995801418,9.36829843431533));
#10553=CARTESIAN_POINT('Ctrl Pts',(43.6328192933167,-29.9750449290915,9.20951371508966));
#10554=CARTESIAN_POINT('Ctrl Pts',(41.9908418354334,-33.0388817878925,9.05072899586395));
#10555=CARTESIAN_POINT('Ctrl Pts',(38.5262719144904,-33.3205496312506,8.89194427663829));
#10556=CARTESIAN_POINT('Ctrl Pts',(37.0061629941113,-31.3385370033826,8.77784242707611));
#10557=CARTESIAN_POINT('Ctrl Pts',(36.9227280575122,-30.1612865754691,8.71666881725583));
#10558=CARTESIAN_POINT('Ctrl Pts',(36.9240972445879,-30.002414807271,8.70842344717746));
#10559=CARTESIAN_POINT('Ctrl Pts',(36.9295986129496,-30.0034658759783,9.79157655282254));
#10560=CARTESIAN_POINT('Ctrl Pts',(36.9349212216015,-29.2996636162424,9.75519455573124));
#10561=CARTESIAN_POINT('Ctrl Pts',(37.5227895751442,-27.5614666405174,9.66588431889804));
#10562=CARTESIAN_POINT('Ctrl Pts',(40.4091142364954,-26.3909769590634,9.52364584232295));
#10563=CARTESIAN_POINT('Ctrl Pts',(43.2541892892138,-28.3852504471766,9.36486112309727));
#10564=CARTESIAN_POINT('Ctrl Pts',(43.1213433300866,-31.8593327642316,9.20607640387157));
#10565=CARTESIAN_POINT('Ctrl Pts',(40.1303404283627,-33.6304598448459,9.04729168464591));
#10566=CARTESIAN_POINT('Ctrl Pts',(37.4241568402642,-32.2798861452479,8.90912506762956));
#10567=CARTESIAN_POINT('Ctrl Pts',(36.933714701829,-30.6241455749599,8.8238866903551));
#10568=CARTESIAN_POINT('Ctrl Pts',(36.9305018352452,-29.9982750548043,8.79157655282255));
#10569=CARTESIAN_POINT('Ctrl Pts',(41.9134659966651,-28.364012796625,10.));
#10570=CARTESIAN_POINT('Ctrl Pts',(42.4575265280738,-29.0003511034471,9.94707176025811));
#10571=CARTESIAN_POINT('Ctrl Pts',(42.8509955579937,-30.8479873408299,9.84121528077431));
#10572=CARTESIAN_POINT('Ctrl Pts',(40.8305801973719,-32.8592854911677,9.68243056154864));
#10573=CARTESIAN_POINT('Ctrl Pts',(38.0493536846231,-32.246350797925,9.52364584232294));
#10574=CARTESIAN_POINT('Ctrl Pts',(37.0541564286807,-29.5801373012942,9.36486112309728));
#10575=CARTESIAN_POINT('Ctrl Pts',(38.7557049752778,-27.2966971559029,9.20607640387158));
#10576=CARTESIAN_POINT('Ctrl Pts',(41.5964480097995,-27.4888886263241,9.04729168464589));
#10577=CARTESIAN_POINT('Ctrl Pts',(42.9756377325279,-29.9795593326787,8.88850696542022));
#10578=CARTESIAN_POINT('Ctrl Pts',(41.6306960535883,-32.489144265827,8.72972224619452));
#10579=CARTESIAN_POINT('Ctrl Pts',(38.7928711712151,-32.7198580434922,8.57093752696885));
#10580=CARTESIAN_POINT('Ctrl Pts',(37.0601567480849,-30.4606371277457,8.41215280774316));
#10581=CARTESIAN_POINT('Ctrl Pts',(38.0188182770251,-27.7796852899716,8.25336808851749));
#10582=CARTESIAN_POINT('Ctrl Pts',(40.7912199377621,-27.1314075284948,8.09458336929179));
#10583=CARTESIAN_POINT('Ctrl Pts',(42.8392723191738,-29.109272461031,7.93579865006612));
#10584=CARTESIAN_POINT('Ctrl Pts',(42.2880180434828,-31.9025869089777,7.77701393084043));
#10585=CARTESIAN_POINT('Ctrl Pts',(39.6421209206988,-32.9541128850707,7.61822921161475));
#10586=CARTESIAN_POINT('Ctrl Pts',(37.3238562454659,-31.3011981084002,7.45944449238906));
#10587=CARTESIAN_POINT('Ctrl Pts',(37.4555569385905,-28.4570575607117,7.30065977316338));
#10588=CARTESIAN_POINT('Ctrl Pts',(39.9166532379287,-27.0254555270554,7.14187505393769));
#10589=CARTESIAN_POINT('Ctrl Pts',(42.4540521133015,-28.316999721687,6.98309033471202));
#10590=CARTESIAN_POINT('Ctrl Pts',(42.7448068218058,-31.1493029192047,6.82430561548633));
#10591=CARTESIAN_POINT('Ctrl Pts',(40.522736224961,-32.9294382547638,6.66552089626065));
#10592=CARTESIAN_POINT('Ctrl Pts',(37.8221092503229,-32.0277212725262,6.50673617703495));
#10593=CARTESIAN_POINT('Ctrl Pts',(37.1153052795403,-29.2696589553355,6.34795145780928));
#10594=CARTESIAN_POINT('Ctrl Pts',(39.0493916727759,-27.1802118030299,6.18916673858359));
#10595=CARTESIAN_POINT('Ctrl Pts',(41.8537442861862,-27.6722341628753,6.03038201935791));
#10596=CARTESIAN_POINT('Ctrl Pts',(42.9610246280014,-30.2952876945972,5.87159730013222));
#10597=CARTESIAN_POINT('Ctrl Pts',(41.3575358365671,-32.6480102194343,5.71281258090655));
#10598=CARTESIAN_POINT('Ctrl Pts',(38.5112454121581,-32.5765231315497,5.55402786168086));
#10599=CARTESIAN_POINT('Ctrl Pts',(37.0278852198967,-30.1462716786976,5.39524314245518));
#10600=CARTESIAN_POINT('Ctrl Pts',(38.2654470119066,-27.5821109203365,5.23645842322949));
#10601=CARTESIAN_POINT('Ctrl Pts',(41.090963411111,-27.2314876728225,5.07767370400381));
#10602=CARTESIAN_POINT('Ctrl Pts',(42.917720829271,-29.415391727283,4.91888898477813));
#10603=CARTESIAN_POINT('Ctrl Pts',(42.0733530266078,-32.1344949981544,4.76010426555244));
#10604=CARTESIAN_POINT('Ctrl Pts',(39.3308647781861,-32.8995033583434,4.60131954632676));
#10605=CARTESIAN_POINT('Ctrl Pts',(37.2009587717734,-31.0100642913931,4.44253482710107));
#10606=CARTESIAN_POINT('Ctrl Pts',(37.6335287719039,-28.1959280511325,4.28375010787539));
#10607=CARTESIAN_POINT('Ctrl Pts',(40.2325640892091,-27.033389878221,4.12496538864971));
#10608=CARTESIAN_POINT('Ctrl Pts',(42.6186908245506,-28.5867342658908,3.96618066942403));
#10609=CARTESIAN_POINT('Ctrl Pts',(42.6074493687812,-31.4339000869844,3.80739595019834));
#10610=CARTESIAN_POINT('Ctrl Pts',(40.2091310885856,-32.9683540656127,3.64861123097266));
#10611=CARTESIAN_POINT('Ctrl Pts',(37.6193567519611,-31.7853289313531,3.48982651174698));
#10612=CARTESIAN_POINT('Ctrl Pts',(37.2090219816371,-28.9678646538439,3.33104179252129));
#10613=CARTESIAN_POINT('Ctrl Pts',(39.3537814844175,-27.0953032332612,3.17225707329561));
#10614=CARTESIAN_POINT('Ctrl Pts',(42.0901433592587,-27.8819437242824,3.01347235406992));
#10615=CARTESIAN_POINT('Ctrl Pts',(42.9130135240572,-30.6076297374087,2.85468763484424));
#10616=CARTESIAN_POINT('Ctrl Pts',(41.0690679124311,-32.7770407829578,2.69590291561856));
#10617=CARTESIAN_POINT('Ctrl Pts',(38.2464083185899,-32.4041168272699,2.53711819639287));
#10618=CARTESIAN_POINT('Ctrl Pts',(37.0291328782873,-29.8302637079522,2.37833347716719));
#10619=CARTESIAN_POINT('Ctrl Pts',(38.5316373372112,-27.4118012049374,2.21954875794151));
#10620=CARTESIAN_POINT('Ctrl Pts',(41.3784033068818,-27.3627922537806,2.06076403871582));
#10621=CARTESIAN_POINT('Ctrl Pts',(42.9632643203048,-29.7281028107449,1.90197931949014));
#10622=CARTESIAN_POINT('Ctrl Pts',(41.8353047983154,-32.3423319893612,1.74319460026446));
#10623=CARTESIAN_POINT('Ctrl Pts',(39.0271560503567,-32.812192455564,1.58440988103877));
#10624=CARTESIAN_POINT('Ctrl Pts',(37.1096258746627,-30.7075421164847,1.42562516181309));
#10625=CARTESIAN_POINT('Ctrl Pts',(37.838193439687,-27.9551388054256,1.2668404425874));
#10626=CARTESIAN_POINT('Ctrl Pts',(40.5458432691404,-27.0747918173971,1.10805572336172));
#10627=CARTESIAN_POINT('Ctrl Pts',(42.7538144212495,-28.872385292484,0.949271004136037));
#10628=CARTESIAN_POINT('Ctrl Pts',(42.4406504077013,-31.7023699138296,0.790486284910354));
#10629=CARTESIAN_POINT('Ctrl Pts',(39.8932382042214,-32.9737061889096,0.631701565684669));
#10630=CARTESIAN_POINT('Ctrl Pts',(37.4433111114008,-31.5229767898314,0.472916846458986));
#10631=CARTESIAN_POINT('Ctrl Pts',(37.3344969165913,-28.6773615971149,0.314132127233303));
#10632=CARTESIAN_POINT('Ctrl Pts',(39.6648949029946,-27.0438508953382,0.155347408007618));
#10633=CARTESIAN_POINT('Ctrl Pts',(42.3041007393156,-28.1141323568833,-0.00343731121806418));
#10634=CARTESIAN_POINT('Ctrl Pts',(42.8298462181864,-30.9160942000275,-0.162222030443749));
#10635=CARTESIAN_POINT('Ctrl Pts',(41.4590097705807,-32.2158576312381,-0.268078509927538));
#10636=CARTESIAN_POINT('Ctrl Pts',(40.6501999979751,-32.4320868020351,-0.321006749669432));
#10637=CARTESIAN_POINT('Ctrl Pts',(42.0543315503421,-28.2435746787731,10.1070022498898));
#10638=CARTESIAN_POINT('Ctrl Pts',(42.6384447339141,-28.9267589437008,10.0540740101479));
#10639=CARTESIAN_POINT('Ctrl Pts',(43.0608801697441,-30.9104144790625,9.94821753066413));
#10640=CARTESIAN_POINT('Ctrl Pts',(40.8917258563906,-33.0697803912789,9.78943281143844));
#10641=CARTESIAN_POINT('Ctrl Pts',(37.9057509899724,-32.4117226673253,9.63064809221276));
#10642=CARTESIAN_POINT('Ctrl Pts',(36.8372892951947,-29.5492278460832,9.47186337298707));
#10643=CARTESIAN_POINT('Ctrl Pts',(38.6641024550864,-27.0976853874398,9.3130786537614));
#10644=CARTESIAN_POINT('Ctrl Pts',(41.7139753310108,-27.30402561093,9.1542939345357));
#10645=CARTESIAN_POINT('Ctrl Pts',(43.1946982527908,-29.9780545314829,8.99550921531004));
#10646=CARTESIAN_POINT('Ctrl Pts',(41.7507446475367,-32.6723901065155,8.83672449608433));
#10647=CARTESIAN_POINT('Ctrl Pts',(38.7040047523069,-32.920088572745,8.67793977685867));
#10648=CARTESIAN_POINT('Ctrl Pts',(36.8437313461564,-30.4945483151706,8.51915505763297));
#10649=CARTESIAN_POINT('Ctrl Pts',(37.8729676265154,-27.6162301454795,8.3603703384073));
#10650=CARTESIAN_POINT('Ctrl Pts',(40.8494679729022,-26.9202274670375,8.2015856191816));
#10651=CARTESIAN_POINT('Ctrl Pts',(43.0482938894434,-29.0436988745806,8.04280089995593));
#10652=CARTESIAN_POINT('Ctrl Pts',(42.45645737247,-32.0426515658982,7.88401618073024));
#10653=CARTESIAN_POINT('Ctrl Pts',(39.6157745760326,-33.1715887889567,7.72523146150456));
#10654=CARTESIAN_POINT('Ctrl Pts',(37.126843875056,-31.3969897202202,7.56644674227887));
#10655=CARTESIAN_POINT('Ctrl Pts',(37.2682401107661,-28.3434692129799,7.40766202305318));
#10656=CARTESIAN_POINT('Ctrl Pts',(39.9105174153916,-26.8064754903845,7.24887730382751));
#10657=CARTESIAN_POINT('Ctrl Pts',(42.6347145396498,-28.193100594942,7.09009258460182));
#10658=CARTESIAN_POINT('Ctrl Pts',(42.9468740304021,-31.2339123098803,6.93130786537613));
#10659=CARTESIAN_POINT('Ctrl Pts',(40.561219024177,-33.1450976615362,6.77252314615046));
#10660=CARTESIAN_POINT('Ctrl Pts',(37.6617772732529,-32.1769980719337,6.61373842692477));
#10661=CARTESIAN_POINT('Ctrl Pts',(36.9029398026022,-29.2158927029908,6.45495370769909));
#10662=CARTESIAN_POINT('Ctrl Pts',(38.9794097820196,-26.9726246150106,6.2961689884734));
#10663=CARTESIAN_POINT('Ctrl Pts',(41.9902132465463,-27.5008686805263,6.13738426924773));
#10664=CARTESIAN_POINT('Ctrl Pts',(43.1790093606288,-30.3170261862484,5.97859955002204));
#10665=CARTESIAN_POINT('Ctrl Pts',(41.4574749196696,-32.8429514550524,5.81981483079635));
#10666=CARTESIAN_POINT('Ctrl Pts',(38.4016462660687,-32.7662016302113,5.66103011157067));
#10667=CARTESIAN_POINT('Ctrl Pts',(36.809084052371,-30.1570399082051,5.50224539234499));
#10668=CARTESIAN_POINT('Ctrl Pts',(38.1377526773975,-27.4041107444619,5.3434606731193));
#10669=CARTESIAN_POINT('Ctrl Pts',(41.1712779634549,-27.0276753121591,5.18467595389362));
#10670=CARTESIAN_POINT('Ctrl Pts',(43.1325176225281,-29.3723540312048,5.02589123466794));
#10671=CARTESIAN_POINT('Ctrl Pts',(42.2259891448195,-32.2916322664727,4.86710651544225));
#10672=CARTESIAN_POINT('Ctrl Pts',(39.2816043765537,-33.1129590176931,4.70832179621657));
#10673=CARTESIAN_POINT('Ctrl Pts',(36.9948989342501,-31.0844232117526,4.54953707699089));
#10674=CARTESIAN_POINT('Ctrl Pts',(37.4593138758004,-28.0631158692628,4.3907523577652));
#10675=CARTESIAN_POINT('Ctrl Pts',(40.2496849940221,-26.814993952672,4.23196763853952));
#10676=CARTESIAN_POINT('Ctrl Pts',(42.8114736247426,-28.4826924587852,4.07318291931384));
#10677=CARTESIAN_POINT('Ctrl Pts',(42.7994045954005,-31.5394609540302,3.91439820008815));
#10678=CARTESIAN_POINT('Ctrl Pts',(40.224526902588,-33.1868783768316,3.75561348086247));
#10679=CARTESIAN_POINT('Ctrl Pts',(37.4440985399902,-31.9167612896229,3.59682876163679));
#10680=CARTESIAN_POINT('Ctrl Pts',(37.0035557415564,-28.8918809064142,3.4380440424111));
#10681=CARTESIAN_POINT('Ctrl Pts',(39.3062081650313,-26.8814652455344,3.27925932318542));
#10682=CARTESIAN_POINT('Ctrl Pts',(42.2440155483017,-27.7260166419522,3.12047460395973));
#10683=CARTESIAN_POINT('Ctrl Pts',(43.1274637748849,-30.6523622278423,2.96168988473405));
#10684=CARTESIAN_POINT('Ctrl Pts',(41.1477705617938,-32.9814809915411,2.80290516550837));
#10685=CARTESIAN_POINT('Ctrl Pts',(38.1173123934176,-32.5811031173675,2.64412044628268));
#10686=CARTESIAN_POINT('Ctrl Pts',(36.8104235608861,-29.8177680603682,2.485335727057));
#10687=CARTESIAN_POINT('Ctrl Pts',(38.4235394040089,-27.2212631671942,2.32655100783132));
#10688=CARTESIAN_POINT('Ctrl Pts',(41.4798786115659,-27.1686462747144,2.16776628860563));
#10689=CARTESIAN_POINT('Ctrl Pts',(43.1814139346165,-29.7080862814863,2.00898156937995));
#10690=CARTESIAN_POINT('Ctrl Pts',(41.9704162803231,-32.5147698028117,1.85019685015426));
#10691=CARTESIAN_POINT('Ctrl Pts',(38.9555372173872,-33.0192204602371,1.69141213092858));
#10692=CARTESIAN_POINT('Ctrl Pts',(36.8968422912549,-30.7596299571687,1.5326274117029));
#10693=CARTESIAN_POINT('Ctrl Pts',(37.6790455485868,-27.804600199112,1.37384269247721));
#10694=CARTESIAN_POINT('Ctrl Pts',(40.586027162903,-26.8594438201078,1.21505797325153));
#10695=CARTESIAN_POINT('Ctrl Pts',(42.9565447513674,-28.7893725447344,1.05627325402585));
#10696=CARTESIAN_POINT('Ctrl Pts',(42.6203262271891,-31.8276949945432,0.897488534800166));
#10697=CARTESIAN_POINT('Ctrl Pts',(39.8853786135623,-33.1926245127803,0.738703815574479));
#10698=CARTESIAN_POINT('Ctrl Pts',(37.2550927701812,-31.6350953062361,0.579919096348798));
#10699=CARTESIAN_POINT('Ctrl Pts',(37.1382678911857,-28.5799915935394,0.421134377123113));
#10700=CARTESIAN_POINT('Ctrl Pts',(39.640225133523,-26.8262250890235,0.262349657897429));
#10701=CARTESIAN_POINT('Ctrl Pts',(42.4737240443217,-27.9752985389988,0.103564938671746));
#10702=CARTESIAN_POINT('Ctrl Pts',(43.0381738576848,-30.9835352295164,-0.0552197805539384));
#10703=CARTESIAN_POINT('Ctrl Pts',(41.5664191624963,-32.3789846544712,-0.161076260037727));
#10704=CARTESIAN_POINT('Ctrl Pts',(40.698066426161,-32.6111321859386,-0.214004499779622));
#10705=CARTESIAN_POINT('Ctrl Pts',(42.1951971040191,-28.1231365609212,10.2140044997796));
#10706=CARTESIAN_POINT('Ctrl Pts',(42.8193629397544,-28.8531667839546,10.1610762600377));
#10707=CARTESIAN_POINT('Ctrl Pts',(43.2707647814944,-30.9728416172951,10.0552197805539));
#10708=CARTESIAN_POINT('Ctrl Pts',(40.9528715154093,-33.28027529139,9.89643506132827));
#10709=CARTESIAN_POINT('Ctrl Pts',(37.7621482953217,-32.5770945367257,9.73765034210256));
#10710=CARTESIAN_POINT('Ctrl Pts',(36.6204221617086,-29.5183183908723,9.57886562287689));
#10711=CARTESIAN_POINT('Ctrl Pts',(38.572499934895,-26.8986736189766,9.4200809036512));
#10712=CARTESIAN_POINT('Ctrl Pts',(41.8315026522221,-27.1191625955359,9.26129618442551));
#10713=CARTESIAN_POINT('Ctrl Pts',(43.4137587730538,-29.9765497302872,9.10251146519984));
#10714=CARTESIAN_POINT('Ctrl Pts',(41.8707932414851,-32.855635947204,8.94372674597415));
#10715=CARTESIAN_POINT('Ctrl Pts',(38.6151383333986,-33.1203191019978,8.78494202674847));
#10716=CARTESIAN_POINT('Ctrl Pts',(36.6273059442279,-30.5284595025955,8.62615730752278));
#10717=CARTESIAN_POINT('Ctrl Pts',(37.7271169760057,-27.4527750009875,8.46737258829711));
#10718=CARTESIAN_POINT('Ctrl Pts',(40.9077160080424,-26.7090474055801,8.30858786907142));
#10719=CARTESIAN_POINT('Ctrl Pts',(43.2573154597129,-28.9781252881302,8.14980314984573));
#10720=CARTESIAN_POINT('Ctrl Pts',(42.6248967014573,-32.1827162228186,7.99101843062006));
#10721=CARTESIAN_POINT('Ctrl Pts',(39.5894282313664,-33.3890646928428,7.83223371139436));
#10722=CARTESIAN_POINT('Ctrl Pts',(36.9298315046461,-31.4927813320402,7.67344899216869));
#10723=CARTESIAN_POINT('Ctrl Pts',(37.0809232829417,-28.2298808652481,7.514664272943));
#10724=CARTESIAN_POINT('Ctrl Pts',(39.9043815928545,-26.5874954537136,7.35587955371732));
#10725=CARTESIAN_POINT('Ctrl Pts',(42.8153769659981,-28.069201468197,7.19709483449164));
#10726=CARTESIAN_POINT('Ctrl Pts',(43.1489412389985,-31.3185217005559,7.03831011526595));
#10727=CARTESIAN_POINT('Ctrl Pts',(40.5997018233928,-33.3607570683086,6.87952539604027));
#10728=CARTESIAN_POINT('Ctrl Pts',(37.501445296183,-32.326274871341,6.72074067681458));
#10729=CARTESIAN_POINT('Ctrl Pts',(36.690574325664,-29.1621264506462,6.5619559575889));
#10730=CARTESIAN_POINT('Ctrl Pts',(38.9094278912633,-26.7650374269914,6.40317123836322));
#10731=CARTESIAN_POINT('Ctrl Pts',(42.1266822069064,-27.3295031981772,6.24438651913754));
#10732=CARTESIAN_POINT('Ctrl Pts',(43.3969940932563,-30.3387646778996,6.08560179991185));
#10733=CARTESIAN_POINT('Ctrl Pts',(41.557414002772,-33.0378926906704,5.92681708068617));
#10734=CARTESIAN_POINT('Ctrl Pts',(38.2920471199794,-32.9558801288729,5.76803236146048));
#10735=CARTESIAN_POINT('Ctrl Pts',(36.5902828848454,-30.1678081377126,5.6092476422348));
#10736=CARTESIAN_POINT('Ctrl Pts',(38.0100583428884,-27.2261105685873,5.45046292300911));
#10737=CARTESIAN_POINT('Ctrl Pts',(41.2515925157989,-26.8238629514956,5.29167820378343));
#10738=CARTESIAN_POINT('Ctrl Pts',(43.3473144157852,-29.3293163351266,5.13289348455775));
#10739=CARTESIAN_POINT('Ctrl Pts',(42.3786252630313,-32.4487695347909,4.97410876533207));
#10740=CARTESIAN_POINT('Ctrl Pts',(39.2323439749213,-33.3264146770428,4.81532404610638));
#10741=CARTESIAN_POINT('Ctrl Pts',(36.788839096727,-31.158782132112,4.6565393268807));
#10742=CARTESIAN_POINT('Ctrl Pts',(37.285098979697,-27.9303036873932,4.49775460765501));
#10743=CARTESIAN_POINT('Ctrl Pts',(40.266805898835,-26.596598027123,4.33896988842933));
#10744=CARTESIAN_POINT('Ctrl Pts',(43.0042564249346,-28.3786506516797,4.18018516920364));
#10745=CARTESIAN_POINT('Ctrl Pts',(42.9913598220198,-31.645021821076,4.02140044997796));
#10746=CARTESIAN_POINT('Ctrl Pts',(40.2399227165905,-33.4054026880505,3.86261573075228));
#10747=CARTESIAN_POINT('Ctrl Pts',(37.2688403280194,-32.0481936478926,3.7038310115266));
#10748=CARTESIAN_POINT('Ctrl Pts',(36.7980895014757,-28.8158971589845,3.54504629230091));
#10749=CARTESIAN_POINT('Ctrl Pts',(39.2586348456451,-26.6676272578076,3.38626157307523));
#10750=CARTESIAN_POINT('Ctrl Pts',(42.3978877373448,-27.5700895596219,3.22747685384954));
#10751=CARTESIAN_POINT('Ctrl Pts',(43.3419140257126,-30.6970947182758,3.06869213462386));
#10752=CARTESIAN_POINT('Ctrl Pts',(41.2264732111564,-33.1859212001242,2.90990741539818));
#10753=CARTESIAN_POINT('Ctrl Pts',(37.9882164682452,-32.7580894074651,2.75112269617249));
#10754=CARTESIAN_POINT('Ctrl Pts',(36.591714243485,-29.8052724127842,2.59233797694681));
#10755=CARTESIAN_POINT('Ctrl Pts',(38.3154414708065,-27.0307251294511,2.43355325772113));
#10756=CARTESIAN_POINT('Ctrl Pts',(41.5813539162499,-26.9745002956481,2.27476853849544));
#10757=CARTESIAN_POINT('Ctrl Pts',(43.3995635489283,-29.6880697522276,2.11598381926976));
#10758=CARTESIAN_POINT('Ctrl Pts',(42.1055277623309,-32.6872076162622,1.95719910004408));
#10759=CARTESIAN_POINT('Ctrl Pts',(38.8839183844178,-33.2262484649101,1.79841438081839));
#10760=CARTESIAN_POINT('Ctrl Pts',(36.6840587078471,-30.8117177978527,1.63962966159271));
#10761=CARTESIAN_POINT('Ctrl Pts',(37.5198976574866,-27.6540615927984,1.48084494236703));
#10762=CARTESIAN_POINT('Ctrl Pts',(40.6262110566655,-26.6440958228186,1.32206022314134));
#10763=CARTESIAN_POINT('Ctrl Pts',(43.1592750814852,-28.7063597969847,1.16327550391566));
#10764=CARTESIAN_POINT('Ctrl Pts',(42.8000020466769,-31.9530200752568,1.00449078468998));
#10765=CARTESIAN_POINT('Ctrl Pts',(39.8775190229031,-33.411542836651,0.84570606546429));
#10766=CARTESIAN_POINT('Ctrl Pts',(37.0668744289616,-31.7472138226408,0.686921346238608));
#10767=CARTESIAN_POINT('Ctrl Pts',(36.9420388657802,-28.4826215899638,0.528136627012925));
#10768=CARTESIAN_POINT('Ctrl Pts',(39.6155553640513,-26.6085992827088,0.369351907787239));
#10769=CARTESIAN_POINT('Ctrl Pts',(42.6433473493279,-27.8364647211143,0.210567188561557));
#10770=CARTESIAN_POINT('Ctrl Pts',(43.2465014971832,-31.0509762590054,0.0517824693358723));
#10771=CARTESIAN_POINT('Ctrl Pts',(41.673828554412,-32.5421116777044,-0.0540740101479163));
#10772=CARTESIAN_POINT('Ctrl Pts',(40.7459328543469,-32.7901775698422,-0.107002249889811));
#10773=CARTESIAN_POINT('Ctrl Pts',(42.3360626576962,-28.0026984430693,10.3210067496694));
#10774=CARTESIAN_POINT('Ctrl Pts',(43.0002811455947,-28.7795746242084,10.2680785099275));
#10775=CARTESIAN_POINT('Ctrl Pts',(43.4806493932448,-31.0352687555276,10.1622220304437));
#10776=CARTESIAN_POINT('Ctrl Pts',(41.014017174428,-33.4907701915011,10.0034373112181));
#10777=CARTESIAN_POINT('Ctrl Pts',(37.6185456006709,-32.7424664061261,9.84465259199238));
#10778=CARTESIAN_POINT('Ctrl Pts',(36.4035550282225,-29.4874089356614,9.68586787276671));
#10779=CARTESIAN_POINT('Ctrl Pts',(38.4808974147036,-26.6996618505134,9.52708315354101));
#10780=CARTESIAN_POINT('Ctrl Pts',(41.9490299734334,-26.9342995801418,9.36829843431533));
#10781=CARTESIAN_POINT('Ctrl Pts',(43.6328192933167,-29.9750449290915,9.20951371508966));
#10782=CARTESIAN_POINT('Ctrl Pts',(41.9908418354334,-33.0388817878925,9.05072899586395));
#10783=CARTESIAN_POINT('Ctrl Pts',(38.5262719144904,-33.3205496312506,8.89194427663829));
#10784=CARTESIAN_POINT('Ctrl Pts',(36.4108805422994,-30.5623706900205,8.73315955741259));
#10785=CARTESIAN_POINT('Ctrl Pts',(37.5812663254961,-27.2893198564955,8.57437483818692));
#10786=CARTESIAN_POINT('Ctrl Pts',(40.9659640431824,-26.4978673441227,8.41559011896122));
#10787=CARTESIAN_POINT('Ctrl Pts',(43.4663370299824,-28.9125517016798,8.25680539973555));
#10788=CARTESIAN_POINT('Ctrl Pts',(42.7933360304446,-32.322780879739,8.09802068050986));
#10789=CARTESIAN_POINT('Ctrl Pts',(39.5630818867002,-33.6065405967288,7.93923596128418));
#10790=CARTESIAN_POINT('Ctrl Pts',(36.7328191342362,-31.5885729438602,7.7804512420585));
#10791=CARTESIAN_POINT('Ctrl Pts',(36.8936064551174,-28.1162925175164,7.62166652283281));
#10792=CARTESIAN_POINT('Ctrl Pts',(39.8982457703173,-26.3685154170426,7.46288180360713));
#10793=CARTESIAN_POINT('Ctrl Pts',(42.9960393923464,-27.9453023414519,7.30409708438144));
#10794=CARTESIAN_POINT('Ctrl Pts',(43.3510084475949,-31.4031310912316,7.14531236515576));
#10795=CARTESIAN_POINT('Ctrl Pts',(40.6381846226088,-33.576416475081,6.98652764593008));
#10796=CARTESIAN_POINT('Ctrl Pts',(37.3411133191131,-32.4755516707485,6.82774292670439));
#10797=CARTESIAN_POINT('Ctrl Pts',(36.4782088487258,-29.1083601983015,6.66895820747871));
#10798=CARTESIAN_POINT('Ctrl Pts',(38.8394460005071,-26.5574502389721,6.51017348825302));
#10799=CARTESIAN_POINT('Ctrl Pts',(42.2631511672664,-27.1581377158282,6.35138876902735));
#10800=CARTESIAN_POINT('Ctrl Pts',(43.6149788258837,-30.3605031695509,6.19260404980166));
#10801=CARTESIAN_POINT('Ctrl Pts',(41.6573530858745,-33.2328339262885,6.03381933057598));
#10802=CARTESIAN_POINT('Ctrl Pts',(38.1824479738899,-33.1455586275345,5.87503461135029));
#10803=CARTESIAN_POINT('Ctrl Pts',(36.3714817173198,-30.1785763672202,5.7162498921246));
#10804=CARTESIAN_POINT('Ctrl Pts',(37.8823640083793,-27.0481103927127,5.55746517289893));
#10805=CARTESIAN_POINT('Ctrl Pts',(41.3319070681429,-26.6200505908322,5.39868045367324));
#10806=CARTESIAN_POINT('Ctrl Pts',(43.5621112090423,-29.2862786390484,5.23989573444757));
#10807=CARTESIAN_POINT('Ctrl Pts',(42.531261381243,-32.6059068031093,5.08111101522187));
#10808=CARTESIAN_POINT('Ctrl Pts',(39.1830835732889,-33.5398703363926,4.92232629599619));
#10809=CARTESIAN_POINT('Ctrl Pts',(36.5827792592038,-31.2331410524714,4.76354157677051));
#10810=CARTESIAN_POINT('Ctrl Pts',(37.1108840835935,-27.7974915055236,4.60475685754483));
#10811=CARTESIAN_POINT('Ctrl Pts',(40.2839268036481,-26.3782021015739,4.44597213831914));
#10812=CARTESIAN_POINT('Ctrl Pts',(43.1970392251266,-28.2746088445741,4.28718741909346));
#10813=CARTESIAN_POINT('Ctrl Pts',(43.1833150486392,-31.7505826881217,4.12840269986777));
#10814=CARTESIAN_POINT('Ctrl Pts',(40.2553185305929,-33.6239269992694,3.9696179806421));
#10815=CARTESIAN_POINT('Ctrl Pts',(37.0935821160486,-32.1796260061624,3.8108332614164));
#10816=CARTESIAN_POINT('Ctrl Pts',(36.5926232613949,-28.7399134115548,3.65204854219073));
#10817=CARTESIAN_POINT('Ctrl Pts',(39.211061526259,-26.4537892700808,3.49326382296504));
#10818=CARTESIAN_POINT('Ctrl Pts',(42.5517599263879,-27.4141624772917,3.33447910373936));
#10819=CARTESIAN_POINT('Ctrl Pts',(43.5563642765403,-30.7418272087093,3.17569438451367));
#10820=CARTESIAN_POINT('Ctrl Pts',(41.3051758605191,-33.3903614087074,3.01690966528799));
#10821=CARTESIAN_POINT('Ctrl Pts',(37.8591205430729,-32.9350756975626,2.8581249460623));
#10822=CARTESIAN_POINT('Ctrl Pts',(36.3730049260838,-29.7927767652001,2.69934022683663));
#10823=CARTESIAN_POINT('Ctrl Pts',(38.2073435376042,-26.840187091708,2.54055550761094));
#10824=CARTESIAN_POINT('Ctrl Pts',(41.682829220934,-26.7803543165819,2.38177078838526));
#10825=CARTESIAN_POINT('Ctrl Pts',(43.61771316324,-29.668053222969,2.22298606915957));
#10826=CARTESIAN_POINT('Ctrl Pts',(42.2406392443386,-32.8596454297127,2.06420134993389));
#10827=CARTESIAN_POINT('Ctrl Pts',(38.8122995514484,-33.4332764695832,1.9054166307082));
#10828=CARTESIAN_POINT('Ctrl Pts',(36.4712751244393,-30.8638056385366,1.74663191148252));
#10829=CARTESIAN_POINT('Ctrl Pts',(37.3607497663865,-27.5035229864848,1.58784719225684));
#10830=CARTESIAN_POINT('Ctrl Pts',(40.6663949504281,-26.4287478255293,1.42906247303115));
#10831=CARTESIAN_POINT('Ctrl Pts',(43.362005411603,-28.6233470492352,1.27027775380547));
#10832=CARTESIAN_POINT('Ctrl Pts',(42.9796778661648,-32.0783451559703,1.11149303457979));
#10833=CARTESIAN_POINT('Ctrl Pts',(39.869659432244,-33.6304611605218,0.952708315354101));
#10834=CARTESIAN_POINT('Ctrl Pts',(36.878656087742,-31.8593323390454,0.793923596128419));
#10835=CARTESIAN_POINT('Ctrl Pts',(36.7458098403747,-28.3852515863884,0.635138876902735));
#10836=CARTESIAN_POINT('Ctrl Pts',(39.5908855945796,-26.390973476394,0.47635415767705));
#10837=CARTESIAN_POINT('Ctrl Pts',(42.8129706543341,-27.6976309032298,0.317569438451368));
#10838=CARTESIAN_POINT('Ctrl Pts',(43.4548291366816,-31.1184172884943,0.158784719225683));
#10839=CARTESIAN_POINT('Ctrl Pts',(41.7812379463276,-32.7052387009375,0.0529282397418946));
#10840=CARTESIAN_POINT('Ctrl Pts',(40.7937992825329,-32.9692229537457,0.));
#10841=CARTESIAN_POINT('Ctrl Pts',(40.7937992825329,-32.9692229537457,0.));
#10842=CARTESIAN_POINT('Ctrl Pts',(40.8868533414383,-32.9351833633283,-2.56313906977734E-16));
#10843=CARTESIAN_POINT('Ctrl Pts',(40.9778401769864,-32.8963743202609,7.1182815471101E-16));
#10844=CARTESIAN_POINT('Ctrl Pts',(41.0665520083656,-32.8531245549121,6.10622663543836E-16));
#10845=CARTESIAN_POINT('Ctrl Pts',(41.1572336482529,-32.8089144469075,5.07169947463599E-16));
#10846=CARTESIAN_POINT('Ctrl Pts',(41.2455387982709,-32.7600636012823,2.44567181551013E-15));
#10847=CARTESIAN_POINT('Ctrl Pts',(41.3312165904369,-32.7068775829945,2.72004641033163E-15));
#10848=CARTESIAN_POINT('Ctrl Pts',(41.4141659908734,-32.655385262557,2.98568360242218E-15));
#10849=CARTESIAN_POINT('Ctrl Pts',(41.4946530297383,-32.5998286158413,1.76977927080473E-15));
#10850=CARTESIAN_POINT('Ctrl Pts',(41.572416340159,-32.5404542465392,1.99840144432528E-15));
#10851=CARTESIAN_POINT('Ctrl Pts',(41.6404592367772,-32.4885016733999,2.19844584615577E-15));
#10852=CARTESIAN_POINT('Ctrl Pts',(41.7064164820401,-32.4336254394482,-4.49373757059322E-16));
#10853=CARTESIAN_POINT('Ctrl Pts',(41.7700877162758,-32.3759777741253,-5.55111512312578E-16));
#10854=CARTESIAN_POINT('Ctrl Pts',(41.7834303267024,-32.3638974312572,-5.7726936259868E-16));
#10855=CARTESIAN_POINT('Ctrl Pts',(41.796674321218,-32.3516934837044,-1.58746591514753E-15));
#10856=CARTESIAN_POINT('Ctrl Pts',(41.8098006766232,-32.3393836364141,-1.60982338570648E-15));
#10857=CARTESIAN_POINT('Ctrl Pts',(41.8822282662216,-32.2714613122024,-1.73318570922317E-15));
#10858=CARTESIAN_POINT('Ctrl Pts',(41.9511901377659,-32.2002177731016,-2.93438087003687E-15));
#10859=CARTESIAN_POINT('Ctrl Pts',(42.0164469480358,-32.1259441928838,-2.94209101525666E-15));
#10860=CARTESIAN_POINT('Ctrl Pts',(42.0813424310536,-32.0520818658139,-2.9497584693677E-15));
#10861=CARTESIAN_POINT('Ctrl Pts',(42.1425742542194,-31.9752221613491,-1.88528885175235E-15));
#10862=CARTESIAN_POINT('Ctrl Pts',(42.1998634141426,-31.8956246979978,-2.3037127760972E-15));
#10863=CARTESIAN_POINT('Ctrl Pts',(42.2557185048177,-31.8180197280708,-2.71166266166342E-15));
#10864=CARTESIAN_POINT('Ctrl Pts',(42.3078261181292,-31.7378116076102,2.65808508142602E-16));
#10865=CARTESIAN_POINT('Ctrl Pts',(42.3558808204457,-31.6552268221773,2.77555756156289E-16));
#10866=CARTESIAN_POINT('Ctrl Pts',(42.3766084052719,-31.6196052687622,2.8262273332898E-16));
#10867=CARTESIAN_POINT('Ctrl Pts',(42.396581328328,-31.5835414239387,-1.13197147658776E-15));
#10868=CARTESIAN_POINT('Ctrl Pts',(42.4157720959317,-31.5470531303214,-9.15933995315754E-16));
#10869=CARTESIAN_POINT('Ctrl Pts',(42.4294374934211,-31.5210704783355,-7.62097623829557E-16));
#10870=CARTESIAN_POINT('Ctrl Pts',(42.4427062526566,-31.494872601805,-2.6961316652602E-15));
#10871=CARTESIAN_POINT('Ctrl Pts',(42.4555678499899,-31.4684659394331,-2.85882428840978E-15));
#10872=CARTESIAN_POINT('Ctrl Pts',(42.461183367079,-31.4569364956189,-2.92985770532468E-15));
#10873=CARTESIAN_POINT('Ctrl Pts',(42.466720339292,-31.4453690485835,-5.42172902776515E-15));
#10874=CARTESIAN_POINT('Ctrl Pts',(42.4721741965263,-31.4337724107416,-5.32907051820075E-15));
#10875=CARTESIAN_POINT('Ctrl Pts',(42.5124020269377,-31.3482352284496,-4.64561830286583E-15));
#10876=CARTESIAN_POINT('Ctrl Pts',(42.5481738190905,-31.2609849169841,-3.53734486715838E-18));
#10877=CARTESIAN_POINT('Ctrl Pts',(42.5792385941522,-31.1722587986469,1.66533453693773E-16));
#10878=CARTESIAN_POINT('Ctrl Pts',(42.609616658182,-31.085494040215,3.32844704878679E-16));
#10879=CARTESIAN_POINT('Ctrl Pts',(42.6354937269254,-30.9973173268531,1.38062588022343E-15));
#10880=CARTESIAN_POINT('Ctrl Pts',(42.6565859822745,-30.907941771704,2.22044604925031E-15));
#10881=CARTESIAN_POINT('Ctrl Pts',(42.6603146190692,-30.8921421818565,2.36890738405432E-15));
#10882=CARTESIAN_POINT('Ctrl Pts',(42.6638935978244,-30.8763051196421,-1.87440975142009E-15));
#10883=CARTESIAN_POINT('Ctrl Pts',(42.6673211784214,-30.8604317567702,-1.99840144432528E-15));
#10884=CARTESIAN_POINT('Ctrl Pts',(42.6874320816035,-30.7672967728217,-2.78141844429488E-15));
#10885=CARTESIAN_POINT('Ctrl Pts',(42.7023350183962,-30.6729110567368,3.99432902596115E-17));
#10886=CARTESIAN_POINT('Ctrl Pts',(42.7121084797748,-30.5776835032973,-6.66133814775094E-16));
#10887=CARTESIAN_POINT('Ctrl Pts',(42.7153863724595,-30.5457454121019,-9.02942954116546E-16));
#10888=CARTESIAN_POINT('Ctrl Pts',(42.7180868619563,-30.513712748472,9.49954623796192E-16));
#10889=CARTESIAN_POINT('Ctrl Pts',(42.7202116846012,-30.4816014077219,1.11022302462516E-15));
#10890=CARTESIAN_POINT('Ctrl Pts',(42.7214003069685,-30.4636383753964,1.19987691006264E-15));
#10891=CARTESIAN_POINT('Ctrl Pts',(42.7224087772442,-30.4456507281831,-1.70559861591596E-15));
#10892=CARTESIAN_POINT('Ctrl Pts',(42.7232373200213,-30.4276412935577,-1.77635683940025E-15));
#10893=CARTESIAN_POINT('Ctrl Pts',(42.723811587505,-30.415158856935,-1.82539974710676E-15));
#10894=CARTESIAN_POINT('Ctrl Pts',(42.7242993034867,-30.4026674831952,1.16339523992486E-15));
#10895=CARTESIAN_POINT('Ctrl Pts',(42.7247004178212,-30.3901775939692,1.19348975147204E-15));
#10896=CARTESIAN_POINT('Ctrl Pts',(42.7276932514519,-30.2969868069435,1.41803387396094E-15));
#10897=CARTESIAN_POINT('Ctrl Pts',(42.7258764989753,-30.2037315753923,-4.64215791567553E-16));
#10898=CARTESIAN_POINT('Ctrl Pts',(42.7193892630461,-30.1107870263199,9.71445146547012E-17));
#10899=CARTESIAN_POINT('Ctrl Pts',(42.7128890684809,-30.0176568150351,6.59626171160253E-16));
#10900=CARTESIAN_POINT('Ctrl Pts',(42.7016993292407,-29.9248375470543,-1.8032818589036E-15));
#10901=CARTESIAN_POINT('Ctrl Pts',(42.6859089377377,-29.8327186037965,-2.88657986402541E-15));
#10902=CARTESIAN_POINT('Ctrl Pts',(42.6703416524813,-29.7419012312863,-3.95457169058614E-15));
#10903=CARTESIAN_POINT('Ctrl Pts',(42.6503023361097,-29.651763686107,1.83421046840484E-15));
#10904=CARTESIAN_POINT('Ctrl Pts',(42.6258331190092,-29.5627042281559,2.1094237467878E-15));
#10905=CARTESIAN_POINT('Ctrl Pts',(42.6163194528175,-29.5280777850343,2.21642705838946E-15));
#10906=CARTESIAN_POINT('Ctrl Pts',(42.6061357056814,-29.4936146514553,-2.51880313695631E-15));
#10907=CARTESIAN_POINT('Ctrl Pts',(42.5952827870604,-29.4593396971683,-2.66453525910038E-15));
#10908=CARTESIAN_POINT('Ctrl Pts',(42.5894785729062,-29.4410092202016,-2.74247378196201E-15));
#10909=CARTESIAN_POINT('Ctrl Pts',(42.5834829492134,-29.422732581524,4.35205348445305E-15));
#10910=CARTESIAN_POINT('Ctrl Pts',(42.5772959593921,-29.4045136996676,4.52415882534751E-15));
#10911=CARTESIAN_POINT('Ctrl Pts',(42.5718473784623,-29.388469216791,4.6757236259051E-15));
#10912=CARTESIAN_POINT('Ctrl Pts',(42.5662499050538,-29.3724684527645,-1.66194925938346E-15));
#10913=CARTESIAN_POINT('Ctrl Pts',(42.5605096902647,-29.3565304936658,-1.31838984174237E-15));
#10914=CARTESIAN_POINT('Ctrl Pts',(42.5280842271611,-29.2664997676932,6.22316844309968E-16));
#10915=CARTESIAN_POINT('Ctrl Pts',(42.4910677197366,-29.1783477753058,4.42868535318251E-15));
#10916=CARTESIAN_POINT('Ctrl Pts',(42.4495332018698,-29.0925190835637,6.48092690624935E-15));
#10917=CARTESIAN_POINT('Ctrl Pts',(42.4183823134697,-29.0281475647571,8.02010807104948E-15));
#10918=CARTESIAN_POINT('Ctrl Pts',(42.3846888958494,-28.965083439524,2.11771072648854E-15));
#10919=CARTESIAN_POINT('Ctrl Pts',(42.34846639183,-28.9035314164698,3.03229663600746E-15));
#10920=CARTESIAN_POINT('Ctrl Pts',(42.3335346051443,-28.8781581932981,3.40931092799006E-15));
#10921=CARTESIAN_POINT('Ctrl Pts',(42.3181728910835,-28.8530421194055,2.64502491527703E-15));
#10922=CARTESIAN_POINT('Ctrl Pts',(42.3023815334246,-28.8281984400257,2.37310171513627E-15));
#10923=CARTESIAN_POINT('Ctrl Pts',(42.2929488997925,-28.8133585934004,2.21067414061172E-15));
#10924=CARTESIAN_POINT('Ctrl Pts',(42.2833676471414,-28.7986233574288,4.22105548283075E-15));
#10925=CARTESIAN_POINT('Ctrl Pts',(42.2736398143272,-28.7839980537574,3.90659726789977E-15));
#10926=CARTESIAN_POINT('Ctrl Pts',(42.2261111297762,-28.7125410850842,2.37020313084679E-15));
#10927=CARTESIAN_POINT('Ctrl Pts',(42.1750736539845,-28.6436860898129,1.77149268136323E-15));
#10928=CARTESIAN_POINT('Ctrl Pts',(42.1205617687127,-28.5777857785416,2.25514051876985E-16));
#10929=CARTESIAN_POINT('Ctrl Pts',(42.0689757570806,-28.5154226038532,-1.23748564380198E-15));
#10930=CARTESIAN_POINT('Ctrl Pts',(42.014277806743,-28.4557052264058,-1.96483870085748E-15));
#10931=CARTESIAN_POINT('Ctrl Pts',(41.9564732643226,-28.3989684314093,-2.17707796235089E-15));
#10932=CARTESIAN_POINT('Ctrl Pts',(41.9435072914684,-28.3862419619494,-2.23121674702981E-15));
#10933=CARTESIAN_POINT('Ctrl Pts',(41.9303849287496,-28.3736656153915,-2.32254674784139E-15));
#10934=CARTESIAN_POINT('Ctrl Pts',(41.9171094063105,-28.36124072171,-2.27595720048157E-15));
#10935=CARTESIAN_POINT('Ctrl Pts',(37.4805319060517,-30.0019779656107,8.38741669750802));
#10936=CARTESIAN_POINT('Ctrl Pts',(37.4794104066332,-30.1321096319321,8.3956620675864));
#10937=CARTESIAN_POINT('Ctrl Pts',(37.4886219042959,-30.2620820392616,8.40390743766478));
#10938=CARTESIAN_POINT('Ctrl Pts',(37.5087194067633,-30.3903486407411,8.41215280774316));
#10939=CARTESIAN_POINT('Ctrl Pts',(37.6377282224616,-31.2137107663279,8.46508104748506));
#10940=CARTESIAN_POINT('Ctrl Pts',(38.2152996968383,-31.9667844049101,8.51800928722696));
#10941=CARTESIAN_POINT('Ctrl Pts',(38.9770562477556,-32.3048689279236,8.57093752696885));
#10942=CARTESIAN_POINT('Ctrl Pts',(39.7388127986728,-32.6429534509372,8.62386576671074));
#10943=CARTESIAN_POINT('Ctrl Pts',(40.6847544261306,-32.5660488583821,8.67679400645263));
#10944=CARTESIAN_POINT('Ctrl Pts',(41.3818821863494,-32.1093324065798,8.72972224619453));
#10945=CARTESIAN_POINT('Ctrl Pts',(42.0790099465682,-31.6526159547776,8.78265048593643));
#10946=CARTESIAN_POINT('Ctrl Pts',(42.5273238395481,-30.8160876437281,8.83557872567832));
#10947=CARTESIAN_POINT('Ctrl Pts',(42.5216158322499,-29.9827117038109,8.88850696542022));
#10948=CARTESIAN_POINT('Ctrl Pts',(42.5159078249518,-29.1493357638938,8.94143520516211));
#10949=CARTESIAN_POINT('Ctrl Pts',(42.0561779173756,-28.3191121951089,8.994363444904));
#10950=CARTESIAN_POINT('Ctrl Pts',(41.3528557911673,-27.8719684989796,9.0472916846459));
#10951=CARTESIAN_POINT('Ctrl Pts',(40.6495336649589,-27.4248248028504,9.10021992438779));
#10952=CARTESIAN_POINT('Ctrl Pts',(39.7026193201184,-27.3607609793766,9.15314816412968));
#10953=CARTESIAN_POINT('Ctrl Pts',(38.9455707232652,-27.709302425205,9.20607640387158));
#10954=CARTESIAN_POINT('Ctrl Pts',(38.1885221264121,-28.0578438710333,9.25900464361348));
#10955=CARTESIAN_POINT('Ctrl Pts',(37.6213392775464,-28.8189905861637,9.31193288335538));
#10956=CARTESIAN_POINT('Ctrl Pts',(37.5036140624373,-29.6439328598341,9.36486112309727));
#10957=CARTESIAN_POINT('Ctrl Pts',(37.486891043608,-29.7611169750883,9.37237964790086));
#10958=CARTESIAN_POINT('Ctrl Pts',(37.4792374368207,-29.8795883934461,9.37989817270444));
#10959=CARTESIAN_POINT('Ctrl Pts',(37.4802181636634,-29.9981833349058,9.38741669750803));
#10960=CARTESIAN_POINT('Ctrl Pts',(39.2062007174671,-32.9692229537457,10.));
#10961=CARTESIAN_POINT('Ctrl Pts',(38.2187620536724,-32.7052387009375,9.94707176025811));
#10962=CARTESIAN_POINT('Ctrl Pts',(36.5451692871586,-31.1184273543511,9.84121528077431));
#10963=CARTESIAN_POINT('Ctrl Pts',(37.1870307188556,-27.697626748216,9.68243056154864));
#10964=CARTESIAN_POINT('Ctrl Pts',(40.4091142364954,-26.3909769590634,9.52364584232295));
#10965=CARTESIAN_POINT('Ctrl Pts',(43.2541892892138,-28.3852504471766,9.36486112309727));
#10966=CARTESIAN_POINT('Ctrl Pts',(43.1213433300866,-31.8593327642316,9.20607640387157));
#10967=CARTESIAN_POINT('Ctrl Pts',(40.1303404283627,-33.6304598448459,9.04729168464591));
#10968=CARTESIAN_POINT('Ctrl Pts',(37.0203228967143,-32.0783449395581,8.88850696542022));
#10969=CARTESIAN_POINT('Ctrl Pts',(36.6379953175286,-28.6233472228274,8.72972224619453));
#10970=CARTESIAN_POINT('Ctrl Pts',(39.3336052322159,-26.4287487288557,8.57093752696886));
#10971=CARTESIAN_POINT('Ctrl Pts',(42.6392496071423,-27.5035235206868,8.41215280774315));
#10972=CARTESIAN_POINT('Ctrl Pts',(43.5287240702543,-30.8638054618116,8.25336808851749));
#10973=CARTESIAN_POINT('Ctrl Pts',(41.1877001687398,-33.4332756644217,8.09458336929179));
#10974=CARTESIAN_POINT('Ctrl Pts',(37.7593612762403,-32.8596447757211,7.93579865006612));
#10975=CARTESIAN_POINT('Ctrl Pts',(36.3822876706404,-29.6680532961916,7.77701393084043));
#10976=CARTESIAN_POINT('Ctrl Pts',(38.3171711686706,-26.7803550620374,7.61822921161474));
#10977=CARTESIAN_POINT('Ctrl Pts',(41.7926560478477,-26.8401878205589,7.45944449238907));
#10978=CARTESIAN_POINT('Ctrl Pts',(43.6269942364715,-29.7927768135681,7.30065977316338));
#10979=CARTESIAN_POINT('Ctrl Pts',(42.1408789623084,-32.935075019391,7.1418750539377));
#10980=CARTESIAN_POINT('Ctrl Pts',(38.6948244410116,-33.3903606257847,6.98309033471201));
#10981=CARTESIAN_POINT('Ctrl Pts',(36.4436365448214,-30.7418270372989,6.82430561548633));
#10982=CARTESIAN_POINT('Ctrl Pts',(37.4482406630067,-27.4141630745731,6.66552089626065));
#10983=CARTESIAN_POINT('Ctrl Pts',(40.7889382915105,-26.453790089119,6.50673617703496));
#10984=CARTESIAN_POINT('Ctrl Pts',(43.4073759516192,-28.7399137026036,6.34795145780928));
#10985=CARTESIAN_POINT('Ctrl Pts',(42.9064172126614,-32.1796255027351,6.18916673858359));
#10986=CARTESIAN_POINT('Ctrl Pts',(39.7446815283789,-33.6239261622643,6.03038201935791));
#10987=CARTESIAN_POINT('Ctrl Pts',(36.816685686601,-31.7505822837933,5.87159730013222));
#10988=CARTESIAN_POINT('Ctrl Pts',(36.8029615132848,-28.2746092430835,5.71281258090655));
#10989=CARTESIAN_POINT('Ctrl Pts',(39.7160732619294,-26.3782029380897,5.55402786168086));
#10990=CARTESIAN_POINT('Ctrl Pts',(42.8891152491159,-27.7974920142308,5.39524314245518));
#10991=CARTESIAN_POINT('Ctrl Pts',(43.4172199515306,-31.2331407676563,5.2364584232295));
#10992=CARTESIAN_POINT('Ctrl Pts',(40.8169162380303,-33.5398695187991,5.07767370400381));
#10993=CARTESIAN_POINT('Ctrl Pts',(37.4687392033951,-32.6059062012305,4.91888898477812));
#10994=CARTESIAN_POINT('Ctrl Pts',(36.4378896136882,-29.2862788038946,4.76010426555244));
#10995=CARTESIAN_POINT('Ctrl Pts',(38.6680932394838,-26.6200513714892,4.60131954632676));
#10996=CARTESIAN_POINT('Ctrl Pts',(42.1176355025165,-27.0481110745022,4.44253482710108));
#10997=CARTESIAN_POINT('Ctrl Pts',(43.6285174446119,-30.1785763259747,4.28375010787539));
#10998=CARTESIAN_POINT('Ctrl Pts',(41.8175516063153,-33.1455579010144,4.12496538864971));
#10999=CARTESIAN_POINT('Ctrl Pts',(38.3426472969195,-33.2328331796093,3.96618066942402));
#11000=CARTESIAN_POINT('Ctrl Pts',(36.3850220090575,-30.3605030862883,3.80739595019834));
#11001=CARTESIAN_POINT('Ctrl Pts',(37.7368493554468,-27.1581383722016,3.64861123097266));
#11002=CARTESIAN_POINT('Ctrl Pts',(41.1605537314434,-26.5574510340941,3.48982651174697));
#11003=CARTESIAN_POINT('Ctrl Pts',(43.5217903378555,-29.1083604042289,3.33104179252129));
#11004=CARTESIAN_POINT('Ctrl Pts',(42.6588860667731,-32.4755510990005,3.17225707329561));
#11005=CARTESIAN_POINT('Ctrl Pts',(39.3618155247875,-33.5764156490026,3.01347235406992));
#11006=CARTESIAN_POINT('Ctrl Pts',(36.6489923263848,-31.4031307672381,2.85468763484424));
#11007=CARTESIAN_POINT('Ctrl Pts',(37.0039612996256,-27.9453028158605,2.69590291561856));
#11008=CARTESIAN_POINT('Ctrl Pts',(40.1017542062109,-26.3685162560978,2.53711819639287));
#11009=CARTESIAN_POINT('Ctrl Pts',(43.1063928273453,-28.1162929520197,2.37833347716719));
#11010=CARTESIAN_POINT('Ctrl Pts',(43.2671801112825,-31.58857257803,2.2195487579415));
#11011=CARTESIAN_POINT('Ctrl Pts',(40.4369180121167,-33.6065397617092,2.06076403871582));
#11012=CARTESIAN_POINT('Ctrl Pts',(37.2066646152815,-32.3227803470516,1.90197931949014));
#11013=CARTESIAN_POINT('Ctrl Pts',(36.5336637694756,-28.9125519457581,1.74319460026446));
#11014=CARTESIAN_POINT('Ctrl Pts',(39.034036182301,-26.4978681661549,1.58440988103877));
#11015=CARTESIAN_POINT('Ctrl Pts',(42.4187331109537,-27.2893204582939,1.42562516181309));
#11016=CARTESIAN_POINT('Ctrl Pts',(43.5891186388302,-30.5623706046428,1.26684044258741));
#11017=CARTESIAN_POINT('Ctrl Pts',(41.4737277243454,-33.3205487833603,1.10805572336172));
#11018=CARTESIAN_POINT('Ctrl Pts',(38.0091586671154,-33.0388812318245,0.949271004136037));
#11019=CARTESIAN_POINT('Ctrl Pts',(36.3671814579584,-29.9750446753109,0.790486284910354));
#11020=CARTESIAN_POINT('Ctrl Pts',(38.0509706569457,-26.9343007433511,0.63170156568467));
#11021=CARTESIAN_POINT('Ctrl Pts',(41.5191018646847,-26.6996618298828,0.472916846458986));
#11022=CARTESIAN_POINT('Ctrl Pts',(43.5964448997665,-29.4874103675251,0.314132127233304));
#11023=CARTESIAN_POINT('Ctrl Pts',(42.3814522873891,-32.7424636317378,0.155347408007619));
#11024=CARTESIAN_POINT('Ctrl Pts',(38.9859863107926,-33.4907728378243,-0.00343731121806265));
#11025=CARTESIAN_POINT('Ctrl Pts',(36.5193436061198,-31.0352613530379,-0.162222030443749));
#11026=CARTESIAN_POINT('Ctrl Pts',(36.9997188544053,-28.7795746242084,-0.268078509927537));
#11027=CARTESIAN_POINT('Ctrl Pts',(37.6639373423039,-28.0026984430693,-0.321006749669432));
#11028=CARTESIAN_POINT('Ctrl Pts',(39.254067145653,-32.7901775698422,10.1070022498898));
#11029=CARTESIAN_POINT('Ctrl Pts',(38.326171445588,-32.5421116777044,10.0540740101479));
#11030=CARTESIAN_POINT('Ctrl Pts',(36.7534970217,-31.0509857178868,9.94821753066413));
#11031=CARTESIAN_POINT('Ctrl Pts',(37.3566539410579,-27.8364608166496,9.78943281143844));
#11032=CARTESIAN_POINT('Ctrl Pts',(40.3844444772099,-26.6086025553717,9.63064809221276));
#11033=CARTESIAN_POINT('Ctrl Pts',(43.0579603162945,-28.4826205194471,9.47186337298708));
#11034=CARTESIAN_POINT('Ctrl Pts',(42.9331250239721,-31.747214222188,9.31307865376139));
#11035=CARTESIAN_POINT('Ctrl Pts',(40.1224808461091,-33.411541600311,9.15429393453572));
#11036=CARTESIAN_POINT('Ctrl Pts',(37.1999986702002,-31.9530198718943,8.99550921531002));
#11037=CARTESIAN_POINT('Ctrl Pts',(36.8407256036794,-28.7063599601093,8.83672449608434));
#11038=CARTESIAN_POINT('Ctrl Pts',(39.373789114965,-26.644096671674,8.67793977685866));
#11039=CARTESIAN_POINT('Ctrl Pts',(42.4801017538186,-27.6540620947878,8.51915505763297));
#11040=CARTESIAN_POINT('Ctrl Pts',(43.3159405354069,-30.8117176317842,8.36037033840729));
#11041=CARTESIAN_POINT('Ctrl Pts',(41.1160813526431,-33.2262477083002,8.2015856191816));
#11042=CARTESIAN_POINT('Ctrl Pts',(37.8944727268569,-32.6872070017066,8.04280089995594));
#11043=CARTESIAN_POINT('Ctrl Pts',(36.6004372346688,-29.6880698210349,7.88401618073023));
#11044=CARTESIAN_POINT('Ctrl Pts',(38.4186464498613,-26.9745009961524,7.72523146150456));
#11045=CARTESIAN_POINT('Ctrl Pts',(41.6845581396429,-27.030725814352,7.56644674227887));
#11046=CARTESIAN_POINT('Ctrl Pts',(43.4082849695686,-29.8052724582355,7.40766202305319));
#11047=CARTESIAN_POINT('Ctrl Pts',(42.0117830669618,-32.7580887701874,7.24887730382751));
#11048=CARTESIAN_POINT('Ctrl Pts',(38.7735270721919,-33.185920464412,7.09009258460182));
#11049=CARTESIAN_POINT('Ctrl Pts',(36.6580867461206,-30.6970945572015,6.93130786537614));
#11050=CARTESIAN_POINT('Ctrl Pts',(37.6021128165091,-27.570090120887,6.77252314615045));
#11051=CARTESIAN_POINT('Ctrl Pts',(40.7413649831129,-26.6676280274574,6.61373842692477));
#11052=CARTESIAN_POINT('Ctrl Pts',(43.2019097589942,-28.815897432483,6.45495370769909));
#11053=CARTESIAN_POINT('Ctrl Pts',(42.7311590411695,-32.0481931748222,6.29616898847341));
#11054=CARTESIAN_POINT('Ctrl Pts',(39.7600773388253,-33.4054019015172,6.13738426924772));
#11055=CARTESIAN_POINT('Ctrl Pts',(37.0086408688851,-31.6450214411286,5.97859955002204));
#11056=CARTESIAN_POINT('Ctrl Pts',(36.9957442689502,-28.3786510261588,5.81981483079635));
#11057=CARTESIAN_POINT('Ctrl Pts',(39.7331941627881,-26.5965988131964,5.66103011157067));
#11058=CARTESIAN_POINT('Ctrl Pts',(42.7149003932503,-27.9303041654252,5.50224539234499));
#11059=CARTESIAN_POINT('Ctrl Pts',(43.2111601616005,-31.1587818644713,5.3434606731193));
#11060=CARTESIAN_POINT('Ctrl Pts',(40.7676558477754,-33.3264139087506,5.18467595389362));
#11061=CARTESIAN_POINT('Ctrl Pts',(37.6213752863529,-32.4487689692057,5.02589123466793));
#11062=CARTESIAN_POINT('Ctrl Pts',(36.6526863573343,-29.3293164900325,4.86710651544226));
#11063=CARTESIAN_POINT('Ctrl Pts',(38.7484077732778,-26.8238636850788,4.70832179621656));
#11064=CARTESIAN_POINT('Ctrl Pts',(41.9899411975006,-27.2261112092646,4.54953707699089));
#11065=CARTESIAN_POINT('Ctrl Pts',(43.4097163276221,-30.1678080989543,4.3907523577652));
#11066=CARTESIAN_POINT('Ctrl Pts',(41.7079524855398,-32.9558794461623,4.23196763853952));
#11067=CARTESIAN_POINT('Ctrl Pts',(38.4425863569393,-33.0378919890163,4.07318291931383));
#11068=CARTESIAN_POINT('Ctrl Pts',(36.6030066913377,-30.3387645996578,3.91439820008815));
#11069=CARTESIAN_POINT('Ctrl Pts',(37.8733182842871,-27.329503814971,3.75561348086247));
#11070=CARTESIAN_POINT('Ctrl Pts',(41.0905718568507,-26.7650381741672,3.59682876163679));
#11071=CARTESIAN_POINT('Ctrl Pts',(43.3094249099668,-29.1621266441561,3.4380440424111));
#11072=CARTESIAN_POINT('Ctrl Pts',(42.4985541267346,-32.3262743340697,3.27925932318542));
#11073=CARTESIAN_POINT('Ctrl Pts',(39.4002983151154,-33.3607562920431,3.12047460395974));
#11074=CARTESIAN_POINT('Ctrl Pts',(36.8510594883099,-31.3185213960994,2.96168988473405));
#11075=CARTESIAN_POINT('Ctrl Pts',(37.1846236842477,-28.0692019139985,2.80290516550837));
#11076=CARTESIAN_POINT('Ctrl Pts',(40.0956183850892,-26.5874962421734,2.64412044628268));
#11077=CARTESIAN_POINT('Ctrl Pts',(42.9190760427886,-28.2298812735507,2.485335727057));
#11078=CARTESIAN_POINT('Ctrl Pts',(43.0701677863682,-31.4927809882697,2.32655100783132));
#11079=CARTESIAN_POINT('Ctrl Pts',(40.4105716735518,-33.3890639081753,2.16776628860563));
#11080=CARTESIAN_POINT('Ctrl Pts',(37.3751039053313,-32.1827157222525,2.00898156937995));
#11081=CARTESIAN_POINT('Ctrl Pts',(36.7426852915375,-28.9781255174905,1.85019685015427));
#11082=CARTESIAN_POINT('Ctrl Pts',(39.0922842038443,-26.7090481780434,1.69141213092858));
#11083=CARTESIAN_POINT('Ctrl Pts',(42.2728824944264,-27.4527755664972,1.5326274117029));
#11084=CARTESIAN_POINT('Ctrl Pts',(43.3726932862799,-30.5284594223662,1.37384269247721));
#11085=CARTESIAN_POINT('Ctrl Pts',(41.3848613272155,-33.1203183052356,1.21505797325153));
#11086=CARTESIAN_POINT('Ctrl Pts',(38.1292072307599,-32.8556354246672,1.05627325402585));
#11087=CARTESIAN_POINT('Ctrl Pts',(36.5862419329191,-29.9765494918096,0.897488534800165));
#11088=CARTESIAN_POINT('Ctrl Pts',(38.1684979401449,-27.1191636886031,0.73870381557448));
#11089=CARTESIAN_POINT('Ctrl Pts',(41.4274993879465,-26.8986735995899,0.579919096348797));
#11090=CARTESIAN_POINT('Ctrl Pts',(43.3795777706227,-29.518319736394,0.421134377123114));
#11091=CARTESIAN_POINT('Ctrl Pts',(42.2378497200892,-32.5770919296341,0.26234965789743));
#11092=CARTESIAN_POINT('Ctrl Pts',(39.0471317596511,-33.2802777781389,0.103564938671748));
#11093=CARTESIAN_POINT('Ctrl Pts',(36.7292286400114,-30.9728346611785,-0.0552197805539377));
#11094=CARTESIAN_POINT('Ctrl Pts',(37.1806370602456,-28.8531667839546,-0.161076260037726));
#11095=CARTESIAN_POINT('Ctrl Pts',(37.8048028959809,-28.1231365609212,-0.214004499779622));
#11096=CARTESIAN_POINT('Ctrl Pts',(39.301933573839,-32.6111321859386,10.2140044997796));
#11097=CARTESIAN_POINT('Ctrl Pts',(38.4335808375037,-32.3789846544712,10.1610762600377));
#11098=CARTESIAN_POINT('Ctrl Pts',(36.9618247562416,-30.9835440814225,10.0552197805539));
#11099=CARTESIAN_POINT('Ctrl Pts',(37.5262771632602,-27.9752948850832,9.89643506132825));
#11100=CARTESIAN_POINT('Ctrl Pts',(40.3597747179245,-26.82622815168,9.73765034210258));
#11101=CARTESIAN_POINT('Ctrl Pts',(42.8617313433752,-28.5799905917176,9.57886562287688));
#11102=CARTESIAN_POINT('Ctrl Pts',(42.7449067178577,-31.6350956801444,9.42008090365121));
#11103=CARTESIAN_POINT('Ctrl Pts',(40.1146212638554,-33.1926233557761,9.26129618442551));
#11104=CARTESIAN_POINT('Ctrl Pts',(37.3796744436861,-31.8276948042305,9.10251146519985));
#11105=CARTESIAN_POINT('Ctrl Pts',(37.0434558898303,-28.7893726973912,8.94372674597414));
#11106=CARTESIAN_POINT('Ctrl Pts',(39.4139729977141,-26.8594446144923,8.78494202674848));
#11107=CARTESIAN_POINT('Ctrl Pts',(42.3209539004949,-27.8046006688888,8.62615730752278));
#11108=CARTESIAN_POINT('Ctrl Pts',(43.1031570005594,-30.7596298017569,8.46737258829711));
#11109=CARTESIAN_POINT('Ctrl Pts',(41.0444625365464,-33.0192197521787,8.30858786907141));
#11110=CARTESIAN_POINT('Ctrl Pts',(38.0295841774735,-32.514769227692,8.14980314984574));
#11111=CARTESIAN_POINT('Ctrl Pts',(36.8185867986972,-29.7080863458782,7.99101843062005));
#11112=CARTESIAN_POINT('Ctrl Pts',(38.5201217310521,-27.1686469302674,7.83223371139437));
#11113=CARTESIAN_POINT('Ctrl Pts',(41.5764602314379,-27.2212638081451,7.67344899216869));
#11114=CARTESIAN_POINT('Ctrl Pts',(43.1895757026657,-29.817768102903,7.514664272943));
#11115=CARTESIAN_POINT('Ctrl Pts',(41.8826871716151,-32.5811025209839,7.35587955371732));
#11116=CARTESIAN_POINT('Ctrl Pts',(38.8522297033722,-32.9814803030395,7.19709483449163));
#11117=CARTESIAN_POINT('Ctrl Pts',(36.8725369474198,-30.652362077104,7.03831011526595));
#11118=CARTESIAN_POINT('Ctrl Pts',(37.7559849700114,-27.726017167201,6.87952539604027));
#11119=CARTESIAN_POINT('Ctrl Pts',(40.6937916747153,-26.8814659657959,6.72074067681458));
#11120=CARTESIAN_POINT('Ctrl Pts',(42.996443566369,-28.8918811623623,6.56195595758891));
#11121=CARTESIAN_POINT('Ctrl Pts',(42.5559008696777,-31.9167608469093,6.40317123836321));
#11122=CARTESIAN_POINT('Ctrl Pts',(39.7754731492718,-33.18687764077,6.24438651913754));
#11123=CARTESIAN_POINT('Ctrl Pts',(37.200596051169,-31.539460598464,6.08560179991185));
#11124=CARTESIAN_POINT('Ctrl Pts',(37.1885270246158,-28.4826928092341,5.92681708068617));
#11125=CARTESIAN_POINT('Ctrl Pts',(39.7503150636467,-26.8149946883032,5.76803236146048));
#11126=CARTESIAN_POINT('Ctrl Pts',(42.5406855373847,-28.0631163166195,5.6092476422348));
#11127=CARTESIAN_POINT('Ctrl Pts',(43.0051003716703,-31.0844229612864,5.45046292300912));
#11128=CARTESIAN_POINT('Ctrl Pts',(40.7183954575206,-33.112958298702,5.29167820378343));
#11129=CARTESIAN_POINT('Ctrl Pts',(37.7740113693106,-32.291631737181,5.13289348455775));
#11130=CARTESIAN_POINT('Ctrl Pts',(36.8674831009805,-29.3723541761704,4.97410876533207));
#11131=CARTESIAN_POINT('Ctrl Pts',(38.8287223070717,-27.0276759986683,4.81532404610638));
#11132=CARTESIAN_POINT('Ctrl Pts',(41.8622468924847,-27.404111344027,4.6565393268807));
#11133=CARTESIAN_POINT('Ctrl Pts',(43.1909152106323,-30.1570398719339,4.49775460765501));
#11134=CARTESIAN_POINT('Ctrl Pts',(41.5983533647642,-32.7662009913101,4.33896988842933));
#11135=CARTESIAN_POINT('Ctrl Pts',(38.5425254169591,-32.8429507984234,4.18018516920365));
#11136=CARTESIAN_POINT('Ctrl Pts',(36.8209913736178,-30.3170261130273,4.02140044997796));
#11137=CARTESIAN_POINT('Ctrl Pts',(38.0097872131274,-27.5008692577405,3.86261573075228));
#11138=CARTESIAN_POINT('Ctrl Pts',(41.0205899822579,-26.9726253142402,3.7038310115266));
#11139=CARTESIAN_POINT('Ctrl Pts',(43.0970594820782,-29.2158928840833,3.54504629230091));
#11140=CARTESIAN_POINT('Ctrl Pts',(42.3382221866959,-32.1769975691389,3.38626157307523));
#11141=CARTESIAN_POINT('Ctrl Pts',(39.4387811054433,-33.1450969350836,3.22747685384954));
#11142=CARTESIAN_POINT('Ctrl Pts',(37.0531266502349,-31.2339120249606,3.06869213462386));
#11143=CARTESIAN_POINT('Ctrl Pts',(37.3652860688698,-28.1931010121365,2.90990741539817));
#11144=CARTESIAN_POINT('Ctrl Pts',(40.0894825639675,-26.8064762282489,2.7511226961725));
#11145=CARTESIAN_POINT('Ctrl Pts',(42.7317592582321,-28.3434695950818,2.59233797694681));
#11146=CARTESIAN_POINT('Ctrl Pts',(42.8731554614538,-31.3969893985094,2.43355325772113));
#11147=CARTESIAN_POINT('Ctrl Pts',(40.384225334987,-33.1715880546413,2.27476853849545));
#11148=CARTESIAN_POINT('Ctrl Pts',(37.543543195381,-32.0426510974533,2.11598381926976));
#11149=CARTESIAN_POINT('Ctrl Pts',(36.9517068135993,-29.0436990892229,1.95719910004408));
#11150=CARTESIAN_POINT('Ctrl Pts',(39.1505322253877,-26.9202281899319,1.79841438081839));
#11151=CARTESIAN_POINT('Ctrl Pts',(42.1270318778991,-27.6162306747005,1.63962966159271));
#11152=CARTESIAN_POINT('Ctrl Pts',(43.1562679337296,-30.4945482400896,1.48084494236703));
#11153=CARTESIAN_POINT('Ctrl Pts',(41.2959949300857,-32.920087827111,1.32206022314134));
#11154=CARTESIAN_POINT('Ctrl Pts',(38.2492557944043,-32.6723896175098,1.16327550391566));
#11155=CARTESIAN_POINT('Ctrl Pts',(36.8053024078799,-29.9780543083085,1.00449078468998));
#11156=CARTESIAN_POINT('Ctrl Pts',(38.286025223344,-27.3040266338552,0.845706065464291));
#11157=CARTESIAN_POINT('Ctrl Pts',(41.3358969112083,-27.0976853692971,0.686921346238607));
#11158=CARTESIAN_POINT('Ctrl Pts',(43.1627106414789,-29.549229105263,0.528136627012926));
#11159=CARTESIAN_POINT('Ctrl Pts',(42.0942471527894,-32.4117202275306,0.36935190778724));
#11160=CARTESIAN_POINT('Ctrl Pts',(39.1082772085095,-33.0697827184533,0.210567188561559));
#11161=CARTESIAN_POINT('Ctrl Pts',(36.939113673903,-30.9104079693192,0.0517824693358731));
#11162=CARTESIAN_POINT('Ctrl Pts',(37.3615552660859,-28.9267589437008,-0.0540740101479155));
#11163=CARTESIAN_POINT('Ctrl Pts',(37.9456684496579,-28.2435746787731,-0.107002249889811));
#11164=CARTESIAN_POINT('Ctrl Pts',(39.3498000020249,-32.4320868020351,10.3210067496694));
#11165=CARTESIAN_POINT('Ctrl Pts',(38.5409902294193,-32.2158576312381,10.2680785099275));
#11166=CARTESIAN_POINT('Ctrl Pts',(37.170152490783,-30.9161024449581,10.1622220304438));
#11167=CARTESIAN_POINT('Ctrl Pts',(37.6959003854625,-28.1141289535168,10.0034373112181));
#11168=CARTESIAN_POINT('Ctrl Pts',(40.335104958639,-27.0438537479883,9.84465259199239));
#11169=CARTESIAN_POINT('Ctrl Pts',(42.6655023704558,-28.6773606639881,9.6858678727667));
#11170=CARTESIAN_POINT('Ctrl Pts',(42.5566884117433,-31.5229771381009,9.52708315354101));
#11171=CARTESIAN_POINT('Ctrl Pts',(40.1067616816018,-32.9737051112411,9.36829843431534));
#11172=CARTESIAN_POINT('Ctrl Pts',(37.559350217172,-31.7023697365666,9.20951371508965));
#11173=CARTESIAN_POINT('Ctrl Pts',(37.2461861759812,-28.8723854346731,9.05072899586396));
#11174=CARTESIAN_POINT('Ctrl Pts',(39.4541568804632,-27.0747925573107,8.89194427663828));
#11175=CARTESIAN_POINT('Ctrl Pts',(42.1618060471712,-27.9551392429898,8.7331595574126));
#11176=CARTESIAN_POINT('Ctrl Pts',(42.8903734657118,-30.7075419717295,8.57437483818692));
#11177=CARTESIAN_POINT('Ctrl Pts',(40.9728437204498,-32.8121917960571,8.41559011896122));
#11178=CARTESIAN_POINT('Ctrl Pts',(38.1646956280901,-32.3423314536776,8.25680539973556));
#11179=CARTESIAN_POINT('Ctrl Pts',(37.0367363627256,-29.7281028707214,8.09802068050985));
#11180=CARTESIAN_POINT('Ctrl Pts',(38.6215970122427,-27.3627928643824,7.93923596128418));
#11181=CARTESIAN_POINT('Ctrl Pts',(41.468362323233,-27.4118018019382,7.7804512420585));
#11182=CARTESIAN_POINT('Ctrl Pts',(42.9708664357628,-29.8302637475704,7.62166652283281));
#11183=CARTESIAN_POINT('Ctrl Pts',(41.7535912762685,-32.4041162717803,7.46288180360713));
#11184=CARTESIAN_POINT('Ctrl Pts',(38.9309323345525,-32.7770401416668,7.30409708438144));
#11185=CARTESIAN_POINT('Ctrl Pts',(37.0869871487189,-30.6076295970066,7.14531236515576));
#11186=CARTESIAN_POINT('Ctrl Pts',(37.9098571235138,-27.8819442135148,6.98652764593008));
#11187=CARTESIAN_POINT('Ctrl Pts',(40.6462183663177,-27.0953039041344,6.82774292670439));
#11188=CARTESIAN_POINT('Ctrl Pts',(42.7909773737438,-28.9678648922416,6.66895820747872));
#11189=CARTESIAN_POINT('Ctrl Pts',(42.3806426981861,-31.7853285189965,6.51017348825302));
#11190=CARTESIAN_POINT('Ctrl Pts',(39.7908689597182,-32.9683533800229,6.35138876902734));
#11191=CARTESIAN_POINT('Ctrl Pts',(37.3925512334531,-31.4338997557994,6.19260404980166));
#11192=CARTESIAN_POINT('Ctrl Pts',(37.3813097802812,-28.5867345923093,6.03381933057598));
#11193=CARTESIAN_POINT('Ctrl Pts',(39.7674359645054,-27.03339056341,5.87503461135029));
#11194=CARTESIAN_POINT('Ctrl Pts',(42.3664706815192,-28.1959284678139,5.71624989212461));
#11195=CARTESIAN_POINT('Ctrl Pts',(42.7990405817402,-31.0100640581014,5.55746517289893));
#11196=CARTESIAN_POINT('Ctrl Pts',(40.6691350672658,-32.8995026886535,5.39868045367324));
#11197=CARTESIAN_POINT('Ctrl Pts',(37.9266474522684,-32.1344945051563,5.23989573444756));
#11198=CARTESIAN_POINT('Ctrl Pts',(37.0822798446267,-29.4153918623083,5.08111101522188));
#11199=CARTESIAN_POINT('Ctrl Pts',(38.9090368408656,-27.2314883122577,4.92232629599619));
#11200=CARTESIAN_POINT('Ctrl Pts',(41.7345525874688,-27.5821114787895,4.76354157677051));
#11201=CARTESIAN_POINT('Ctrl Pts',(42.9721140936425,-30.1462716449134,4.60475685754482));
#11202=CARTESIAN_POINT('Ctrl Pts',(41.4887542439886,-32.576522536458,4.44597213831914));
#11203=CARTESIAN_POINT('Ctrl Pts',(38.6424644769789,-32.6480096078303,4.28718741909346));
#11204=CARTESIAN_POINT('Ctrl Pts',(37.038976055898,-30.2952876263969,4.12840269986778));
#11205=CARTESIAN_POINT('Ctrl Pts',(38.1462561419676,-27.67223470051,3.96961798064208));
#11206=CARTESIAN_POINT('Ctrl Pts',(40.9506081076652,-27.1802124543133,3.81083326141641));
#11207=CARTESIAN_POINT('Ctrl Pts',(42.8846940541895,-29.2696591240105,3.65204854219072));
#11208=CARTESIAN_POINT('Ctrl Pts',(42.1778902466573,-32.0277208042081,3.49326382296504));
#11209=CARTESIAN_POINT('Ctrl Pts',(39.4772638957712,-32.929437578124,3.33447910373935));
#11210=CARTESIAN_POINT('Ctrl Pts',(37.25519381216,-31.149302653822,3.17569438451368));
#11211=CARTESIAN_POINT('Ctrl Pts',(37.5459484534919,-28.3170001102745,3.01690966528798));
#11212=CARTESIAN_POINT('Ctrl Pts',(40.0833467428457,-27.0254562143245,2.85812494606231));
#11213=CARTESIAN_POINT('Ctrl Pts',(42.5444424736755,-28.4570579166128,2.69934022683662));
#11214=CARTESIAN_POINT('Ctrl Pts',(42.6761431365394,-31.3011978087492,2.54055550761094));
#11215=CARTESIAN_POINT('Ctrl Pts',(40.3578789964222,-32.9541122011072,2.38177078838526));
#11216=CARTESIAN_POINT('Ctrl Pts',(37.7119824854307,-31.9025864726542,2.22298606915957));
#11217=CARTESIAN_POINT('Ctrl Pts',(37.1607283356612,-29.1092726609553,2.06420134993389));
#11218=CARTESIAN_POINT('Ctrl Pts',(39.208780246931,-27.1314082018204,1.9054166307082));
#11219=CARTESIAN_POINT('Ctrl Pts',(41.9811812613717,-27.7796857829038,1.74663191148252));
#11220=CARTESIAN_POINT('Ctrl Pts',(42.9398425811794,-30.460637057813,1.58784719225683));
#11221=CARTESIAN_POINT('Ctrl Pts',(41.2071285329557,-32.7198573489864,1.42906247303115));
#11222=CARTESIAN_POINT('Ctrl Pts',(38.3693043580489,-32.4891438103524,1.27027775380547));
#11223=CARTESIAN_POINT('Ctrl Pts',(37.0243628828405,-29.9795591248073,1.11149303457979));
#11224=CARTESIAN_POINT('Ctrl Pts',(38.4035525065433,-27.4888895791073,0.952708315354101));
#11225=CARTESIAN_POINT('Ctrl Pts',(41.24429443447,-27.2966971390043,0.793923596128418));
#11226=CARTESIAN_POINT('Ctrl Pts',(42.9458435123352,-29.5801384741319,0.635138876902737));
#11227=CARTESIAN_POINT('Ctrl Pts',(41.9506445854895,-32.246348525427,0.476354157677051));
#11228=CARTESIAN_POINT('Ctrl Pts',(39.169422657368,-32.8592876587678,0.31756943845137));
#11229=CARTESIAN_POINT('Ctrl Pts',(37.1489987077945,-30.8479812774599,0.158784719225684));
#11230=CARTESIAN_POINT('Ctrl Pts',(37.5424734719262,-29.0003511034471,0.0529282397418953));
#11231=CARTESIAN_POINT('Ctrl Pts',(38.0865340033349,-28.364012796625,0.));
#11232=CARTESIAN_POINT('Ctrl Pts',(38.0865340033349,-28.364012796625,5.55111512312578E-17));
#11233=CARTESIAN_POINT('Ctrl Pts',(38.0249211430992,-28.421913756063,2.3104639589866E-16));
#11234=CARTESIAN_POINT('Ctrl Pts',(37.9666794538551,-28.482965221658,1.28255707534279E-15));
#11235=CARTESIAN_POINT('Ctrl Pts',(37.9118058265048,-28.5467823968405,9.43689570931383E-16));
#11236=CARTESIAN_POINT('Ctrl Pts',(37.8554795264063,-28.6122890078363,5.95851207244836E-16));
#11237=CARTESIAN_POINT('Ctrl Pts',(37.8027015385178,-28.6807101321021,2.62784299857289E-16));
#11238=CARTESIAN_POINT('Ctrl Pts',(37.753494049528,-28.7516781506113,6.10622663543836E-16));
#11239=CARTESIAN_POINT('Ctrl Pts',(37.7025923854307,-28.8250895421285,9.7043682825834E-16));
#11240=CARTESIAN_POINT('Ctrl Pts',(37.6555107288522,-28.9012267438899,2.71054820682649E-15));
#11241=CARTESIAN_POINT('Ctrl Pts',(37.6123085670218,-28.9797268371754,2.99760216648792E-15));
#11242=CARTESIAN_POINT('Ctrl Pts',(37.593407621221,-29.0140706279878,3.1231882738398E-15));
#11243=CARTESIAN_POINT('Ctrl Pts',(37.5752497289795,-29.0488671972833,4.75485736688032E-16));
#11244=CARTESIAN_POINT('Ctrl Pts',(37.5578423170003,-29.0840882429965,4.44089209850063E-16));
#11245=CARTESIAN_POINT('Ctrl Pts',(37.5483341381148,-29.1033264849348,4.26939975149549E-16));
#11246=CARTESIAN_POINT('Ctrl Pts',(37.5390498923763,-29.122691389158,1.61863618687202E-15));
#11247=CARTESIAN_POINT('Ctrl Pts',(37.5299909937341,-29.142178472125,1.60982338570648E-15));
#11248=CARTESIAN_POINT('Ctrl Pts',(37.5213410583467,-29.1607858122899,1.60140843774476E-15));
#11249=CARTESIAN_POINT('Ctrl Pts',(37.5128940924849,-29.179510547703,9.17086461423256E-17));
#11250=CARTESIAN_POINT('Ctrl Pts',(37.5046654270074,-29.1983159954623,1.66533453693773E-16));
#11251=CARTESIAN_POINT('Ctrl Pts',(37.4681044896221,-29.2818708318945,4.98988954677069E-16));
#11252=CARTESIAN_POINT('Ctrl Pts',(37.4358037760726,-29.3671091286622,3.22759138281679E-15));
#11253=CARTESIAN_POINT('Ctrl Pts',(37.4077875615482,-29.4536320411872,2.91433543964104E-15));
#11254=CARTESIAN_POINT('Ctrl Pts',(37.3793090722073,-29.5415826042421,2.59591069203894E-15));
#11255=CARTESIAN_POINT('Ctrl Pts',(37.3552571471219,-29.6308612814779,2.04735700495589E-15));
#11256=CARTESIAN_POINT('Ctrl Pts',(37.3356963907766,-29.7210862860857,1.55431223447522E-15));
#11257=CARTESIAN_POINT('Ctrl Pts',(37.3164739269567,-29.809750898849,1.06979440219971E-15));
#11258=CARTESIAN_POINT('Ctrl Pts',(37.3015883718447,-29.8993302989097,-4.96142364632893E-16));
#11259=CARTESIAN_POINT('Ctrl Pts',(37.2911437360475,-29.9894850121972,1.38777878078145E-16));
#11260=CARTESIAN_POINT('Ctrl Pts',(37.2870135672285,-30.0251352917219,3.89847215477509E-16));
#11261=CARTESIAN_POINT('Ctrl Pts',(37.2835783142426,-30.0608757129787,-2.36101949319689E-15));
#11262=CARTESIAN_POINT('Ctrl Pts',(37.2808464374724,-30.0966858197535,-2.74780198594726E-15));
#11263=CARTESIAN_POINT('Ctrl Pts',(37.2792295134997,-30.1178808534167,-2.97672808230688E-15));
#11264=CARTESIAN_POINT('Ctrl Pts',(37.2778590143499,-30.139100302959,-1.71621991249039E-15));
#11265=CARTESIAN_POINT('Ctrl Pts',(37.2767368966041,-30.1603399498113,-1.85962356624714E-15));
#11266=CARTESIAN_POINT('Ctrl Pts',(37.275989979541,-30.1744777305437,-1.95507757389332E-15));
#11267=CARTESIAN_POINT('Ctrl Pts',(37.2753531910632,-30.1886244564323,2.6775874477929E-15));
#11268=CARTESIAN_POINT('Ctrl Pts',(37.2748274592582,-30.2027643272738,2.60902410786912E-15));
#11269=CARTESIAN_POINT('Ctrl Pts',(37.271288634922,-30.2979431210418,2.147508153176E-15));
#11270=CARTESIAN_POINT('Ctrl Pts',(37.2727685565052,-30.3929728938572,1.24544634177833E-15));
#11271=CARTESIAN_POINT('Ctrl Pts',(37.2793258761199,-30.4874549271961,1.83186799063151E-15));
#11272=CARTESIAN_POINT('Ctrl Pts',(37.2858607014982,-30.5816128492639,2.41627797801546E-15));
#11273=CARTESIAN_POINT('Ctrl Pts',(37.2974377903602,-30.6752277367775,4.55832449058614E-16));
#11274=CARTESIAN_POINT('Ctrl Pts',(37.3141631908863,-30.7679228633085,2.77555756156289E-16));
#11275=CARTESIAN_POINT('Ctrl Pts',(37.3161000547763,-30.7786573053969,2.56910648831923E-16));
#11276=CARTESIAN_POINT('Ctrl Pts',(37.3181060167709,-30.7893794234663,4.5835681127338E-16));
#11277=CARTESIAN_POINT('Ctrl Pts',(37.3201812867948,-30.8000886389312,4.16333634234434E-16));
#11278=CARTESIAN_POINT('Ctrl Pts',(37.3377261922751,-30.8906273018195,6.31236541414227E-17));
#11279=CARTESIAN_POINT('Ctrl Pts',(37.3602204912016,-30.9802440608068,2.25684169593055E-15));
#11280=CARTESIAN_POINT('Ctrl Pts',(37.387388888656,-31.0687009861654,3.05311331771918E-15));
#11281=CARTESIAN_POINT('Ctrl Pts',(37.3981371536463,-31.1036960010747,3.36813147105597E-15));
#11282=CARTESIAN_POINT('Ctrl Pts',(37.4096175528861,-31.1385094369092,4.01162441398018E-15));
#11283=CARTESIAN_POINT('Ctrl Pts',(37.4218152344547,-31.1731262189978,3.88578058618805E-15));
#11284=CARTESIAN_POINT('Ctrl Pts',(37.427769072972,-31.1900230964399,3.82435466480679E-15));
#11285=CARTESIAN_POINT('Ctrl Pts',(37.4338938246471,-31.2068731161624,3.27596104949439E-15));
#11286=CARTESIAN_POINT('Ctrl Pts',(37.4401878632928,-31.2236744969284,3.44169137633799E-15));
#11287=CARTESIAN_POINT('Ctrl Pts',(37.445432955005,-31.2376758064166,3.57980154894933E-15));
#11288=CARTESIAN_POINT('Ctrl Pts',(37.4507927155412,-31.251635532049,4.17563321267137E-15));
#11289=CARTESIAN_POINT('Ctrl Pts',(37.4562639276339,-31.2655480863479,4.08006961549745E-15));
#11290=CARTESIAN_POINT('Ctrl Pts',(37.4904885203169,-31.3525766087289,3.48228156904737E-15));
#11291=CARTESIAN_POINT('Ctrl Pts',(37.5290915581906,-31.4378170268534,4.25521230771052E-15));
#11292=CARTESIAN_POINT('Ctrl Pts',(37.5717405530417,-31.5210374660102,3.89965837399586E-15));
#11293=CARTESIAN_POINT('Ctrl Pts',(37.6159697990177,-31.607341429012,3.53093028446207E-15));
#11294=CARTESIAN_POINT('Ctrl Pts',(37.6645505115892,-31.691473675336,8.20810124271393E-16));
#11295=CARTESIAN_POINT('Ctrl Pts',(37.7171678191012,-31.7731720613104,1.9151347174784E-15));
#11296=CARTESIAN_POINT('Ctrl Pts',(37.7703627831117,-31.8557673689594,3.0214732989067E-15));
#11297=CARTESIAN_POINT('Ctrl Pts',(37.8276838779193,-31.9358759006778,2.22421601072444E-15));
#11298=CARTESIAN_POINT('Ctrl Pts',(37.8888573645074,-32.0132114269328,3.02535774210355E-15));
#11299=CARTESIAN_POINT('Ctrl Pts',(37.9126742306003,-32.0433207108035,3.33726877418507E-15));
#11300=CARTESIAN_POINT('Ctrl Pts',(37.9370755579706,-32.07300943183,1.70170386855551E-15));
#11301=CARTESIAN_POINT('Ctrl Pts',(37.9620470578005,-32.1022596583239,1.67921232474555E-15));
#11302=CARTESIAN_POINT('Ctrl Pts',(37.9820283447379,-32.1256646268897,1.66121540851732E-15));
#11303=CARTESIAN_POINT('Ctrl Pts',(38.0023747117564,-32.1487888334358,3.62130422901362E-15));
#11304=CARTESIAN_POINT('Ctrl Pts',(38.0230792744415,-32.171622749665,3.87190279838023E-15));
#11305=CARTESIAN_POINT('Ctrl Pts',(38.0346329406524,-32.1843646486566,4.01174309674448E-15));
#11306=CARTESIAN_POINT('Ctrl Pts',(38.0462930844947,-32.1970105005967,2.59157039562667E-15));
#11307=CARTESIAN_POINT('Ctrl Pts',(38.0580534283639,-32.2095538559179,2.42861286636753E-15));
#11308=CARTESIAN_POINT('Ctrl Pts',(38.1271088212578,-32.2832070024204,1.4717449096841E-15));
#11309=CARTESIAN_POINT('Ctrl Pts',(38.199664805144,-32.3533827208338,3.45538810407262E-15));
#11310=CARTESIAN_POINT('Ctrl Pts',(38.275409437109,-32.4197921562816,3.53883589099269E-15));
#11311=CARTESIAN_POINT('Ctrl Pts',(38.3396605957844,-32.4761246390439,3.60962132963588E-15));
#11312=CARTESIAN_POINT('Ctrl Pts',(38.4062071932438,-32.529747132498,5.98119156967079E-15));
#11313=CARTESIAN_POINT('Ctrl Pts',(38.4748836902505,-32.5804684054025,6.17561557447743E-15));
#11314=CARTESIAN_POINT('Ctrl Pts',(38.4975706616452,-32.5972239494044,6.23984266857442E-15));
#11315=CARTESIAN_POINT('Ctrl Pts',(38.5204902321351,-32.6136627516457,2.07827934435607E-15));
#11316=CARTESIAN_POINT('Ctrl Pts',(38.5436369048366,-32.6297774777457,1.62370117351429E-15));
#11317=CARTESIAN_POINT('Ctrl Pts',(38.5602345029377,-32.6413327345538,1.29774046708829E-15));
#11318=CARTESIAN_POINT('Ctrl Pts',(38.5769498432321,-32.6527218838852,5.07588258890606E-15));
#11319=CARTESIAN_POINT('Ctrl Pts',(38.5937663318716,-32.6639327287669,4.86416462663897E-15));
#11320=CARTESIAN_POINT('Ctrl Pts',(38.6801203281873,-32.7215013019905,3.77697618169038E-15));
#11321=CARTESIAN_POINT('Ctrl Pts',(38.7692237115985,-32.7744316059974,-2.13679161323202E-15));
#11322=CARTESIAN_POINT('Ctrl Pts',(38.8607679331194,-32.8224021724615,-2.24126273096203E-15));
#11323=CARTESIAN_POINT('Ctrl Pts',(38.9523121546403,-32.8703727389257,-2.34573384869205E-15));
#11324=CARTESIAN_POINT('Ctrl Pts',(39.0462978596107,-32.9133844785481,-2.61326211847443E-15));
#11325=CARTESIAN_POINT('Ctrl Pts',(39.1424545426358,-32.9510751762973,-3.60171961699685E-15));
#11326=CARTESIAN_POINT('Ctrl Pts',(39.1630225201047,-32.9591372412282,-3.77498740676788E-15));
#11327=CARTESIAN_POINT('Ctrl Pts',(39.1836899454549,-32.9669556727912,-2.23961353901364E-15));
#11328=CARTESIAN_POINT('Ctrl Pts',(39.2044529144508,-32.9745316477842,-2.27595720048157E-15));
#11329=CARTESIAN_POINT('Ctrl Pts',(37.4857778982365,-29.998587099551,9.11258330249199));
#11330=CARTESIAN_POINT('Ctrl Pts',(37.4840985574538,-29.6714493670241,9.09196520028265));
#11331=CARTESIAN_POINT('Ctrl Pts',(37.543355536012,-29.3448947567928,9.07134709807331));
#11332=CARTESIAN_POINT('Ctrl Pts',(37.66637530026,-29.044450672095,9.05072899586396));
#11333=CARTESIAN_POINT('Ctrl Pts',(37.9821764108085,-28.2731878088856,8.99780075612207));
#11334=CARTESIAN_POINT('Ctrl Pts',(38.7181666456359,-27.6739901830981,8.94487251638018));
#11335=CARTESIAN_POINT('Ctrl Pts',(39.5374366241675,-27.5211158178176,8.89194427663828));
#11336=CARTESIAN_POINT('Ctrl Pts',(40.3567066026992,-27.368241452537,8.83901603689639));
#11337=CARTESIAN_POINT('Ctrl Pts',(41.2592563249352,-27.6616903477634,8.78608779715449));
#11338=CARTESIAN_POINT('Ctrl Pts',(41.8319590891433,-28.2671485834999,8.7331595574126));
#11339=CARTESIAN_POINT('Ctrl Pts',(42.4046618533514,-28.8726068192364,8.68023131767071));
#11340=CARTESIAN_POINT('Ctrl Pts',(42.6475176595316,-29.7900743954829,8.62730307792881));
#11341=CARTESIAN_POINT('Ctrl Pts',(42.4493572717447,-30.5995831543275,8.57437483818692));
#11342=CARTESIAN_POINT('Ctrl Pts',(42.2511968839578,-31.409091913172,8.52144659844502));
#11343=CARTESIAN_POINT('Ctrl Pts',(41.6120203022038,-32.1106418546146,8.46851835870312));
#11344=CARTESIAN_POINT('Ctrl Pts',(40.8244073292669,-32.3831067682726,8.41559011896123));
#11345=CARTESIAN_POINT('Ctrl Pts',(40.0367943563299,-32.6555716819306,8.36266187921934));
#11346=CARTESIAN_POINT('Ctrl Pts',(39.10074499221,-32.4989515678041,8.30973363947745));
#11347=CARTESIAN_POINT('Ctrl Pts',(38.444727099256,-31.9849367469148,8.25680539973555));
#11348=CARTESIAN_POINT('Ctrl Pts',(37.8488745713017,-31.5180637641465,8.20873136732103));
#11349=CARTESIAN_POINT('Ctrl Pts',(37.4840438865339,-30.7563454071862,8.16065733490651));
#11350=CARTESIAN_POINT('Ctrl Pts',(37.4791974871636,-29.9986726512116,8.11258330249198));
#11351=CARTESIAN_POINT('Origin',(-40.,30.,12.2084234471774));
#11352=CARTESIAN_POINT('Ctrl Pts',(-43.0762854577871,30.0022177574501,9.70842344717746));
#11353=CARTESIAN_POINT('Ctrl Pts',(-43.0774828058572,30.147004819194,9.70090492237387));
#11354=CARTESIAN_POINT('Ctrl Pts',(-43.0023604322999,31.3098385439038,9.64045815782839));
#11355=CARTESIAN_POINT('Ctrl Pts',(-41.5191022135468,33.3003381593159,9.52708315354102));
#11356=CARTESIAN_POINT('Ctrl Pts',(-38.0509703519274,33.065699819527,9.36829843431533));
#11357=CARTESIAN_POINT('Ctrl Pts',(-36.3671810948824,30.024955201687,9.20951371508965));
#11358=CARTESIAN_POINT('Ctrl Pts',(-38.0091584240807,26.9611184995217,9.05072899586397));
#11359=CARTESIAN_POINT('Ctrl Pts',(-41.4737278989921,26.6794508066113,8.89194427663828));
#11360=CARTESIAN_POINT('Ctrl Pts',(-42.993836649437,28.661463151569,8.77784242707611));
#11361=CARTESIAN_POINT('Ctrl Pts',(-43.0772715769482,29.8387134364101,8.71666881725584));
#11362=CARTESIAN_POINT('Ctrl Pts',(-43.0759023900792,29.9975851856081,8.70842344717746));
#11363=CARTESIAN_POINT('Ctrl Pts',(-43.070401160077,29.9965365385191,9.79157655282254));
#11364=CARTESIAN_POINT('Ctrl Pts',(-43.0650787483756,30.7003379664639,9.75519455573124));
#11365=CARTESIAN_POINT('Ctrl Pts',(-42.4772111316602,32.4385313995888,9.66588431889804));
#11366=CARTESIAN_POINT('Ctrl Pts',(-39.5908856649077,33.609025071703,9.52364584232295));
#11367=CARTESIAN_POINT('Ctrl Pts',(-36.7458102038522,31.6147488878258,9.36486112309727));
#11368=CARTESIAN_POINT('Ctrl Pts',(-36.8786563309339,28.140667484321,9.20607640387158));
#11369=CARTESIAN_POINT('Ctrl Pts',(-39.869659490377,26.3695393883571,9.0472916846459));
#11370=CARTESIAN_POINT('Ctrl Pts',(-42.5758435358444,27.7201136457931,8.90912506762955));
#11371=CARTESIAN_POINT('Ctrl Pts',(-43.0662857206963,29.3758543810734,8.8238866903551));
#11372=CARTESIAN_POINT('Ctrl Pts',(-43.0694985803644,30.001724961275,8.79157655282254));
#11373=CARTESIAN_POINT('Ctrl Pts',(-38.0865340033349,31.635987203375,10.));
#11374=CARTESIAN_POINT('Ctrl Pts',(-37.5424734719262,30.999648896553,9.94707176025811));
#11375=CARTESIAN_POINT('Ctrl Pts',(-37.1490014826279,29.1520157886412,9.84121528077432));
#11376=CARTESIAN_POINT('Ctrl Pts',(-39.1694212746662,27.1407133917689,9.68243056154863));
#11377=CARTESIAN_POINT('Ctrl Pts',(-41.9506454231488,27.7536503742996,9.52364584232295));
#11378=CARTESIAN_POINT('Ctrl Pts',(-42.9458435401314,30.41986209395,9.36486112309726));
#11379=CARTESIAN_POINT('Ctrl Pts',(-41.2442947202227,32.7033028521483,9.20607640387159));
#11380=CARTESIAN_POINT('Ctrl Pts',(-38.4035522567032,32.5111108819453,9.0472916846459));
#11381=CARTESIAN_POINT('Ctrl Pts',(-37.0243625854454,30.0204407744419,8.88850696542021));
#11382=CARTESIAN_POINT('Ctrl Pts',(-38.3693041589794,27.5108559695935,8.72972224619454));
#11383=CARTESIAN_POINT('Ctrl Pts',(-41.2071286760087,27.2801423151599,8.57093752696885));
#11384=CARTESIAN_POINT('Ctrl Pts',(-42.9398429054373,29.5393629084276,8.41215280774317));
#11385=CARTESIAN_POINT('Ctrl Pts',(-41.9811814845473,32.2203144553808,8.25336808851748));
#11386=CARTESIAN_POINT('Ctrl Pts',(-39.2087801576347,32.8685921237222,8.09458336929179));
#11387=CARTESIAN_POINT('Ctrl Pts',(-37.1607280190766,30.8907274356912,7.93579865006612));
#11388=CARTESIAN_POINT('Ctrl Pts',(-37.7119822297206,28.0974133164057,7.77701393084042));
#11389=CARTESIAN_POINT('Ctrl Pts',(-40.3578790364915,27.0458874682206,7.61822921161475));
#11390=CARTESIAN_POINT('Ctrl Pts',(-42.6761434353152,28.6988020463829,7.45944449238906));
#11391=CARTESIAN_POINT('Ctrl Pts',(-42.5444427578219,31.5429422554505,7.30065977316338));
#11392=CARTESIAN_POINT('Ctrl Pts',(-40.0833467521405,32.9745441179435,7.1418750539377));
#11393=CARTESIAN_POINT('Ctrl Pts',(-37.5459481794697,31.683000077592,6.98309033471201));
#11394=CARTESIAN_POINT('Ctrl Pts',(-37.2551935056625,28.8506972178761,6.82430561548633));
#11395=CARTESIAN_POINT('Ctrl Pts',(-39.4772638374019,27.0705620947472,6.66552089626065));
#11396=CARTESIAN_POINT('Ctrl Pts',(-42.1778904898475,27.9722789693785,6.50673617703496));
#11397=CARTESIAN_POINT('Ctrl Pts',(-42.8846943763049,30.7303409575371,6.34795145780928));
#11398=CARTESIAN_POINT('Ctrl Pts',(-40.9506082138133,32.8197878605566,6.18916673858359));
#11399=CARTESIAN_POINT('Ctrl Pts',(-38.1462559349721,32.3277655594152,6.03038201935791));
#11400=CARTESIAN_POINT('Ctrl Pts',(-37.0389757252595,29.704712340631,5.87159730013223));
#11401=CARTESIAN_POINT('Ctrl Pts',(-38.6424643253917,27.3519900964832,5.71281258090655));
#11402=CARTESIAN_POINT('Ctrl Pts',(-41.4887544102281,27.4234771758386,5.55402786168086));
#11403=CARTESIAN_POINT('Ctrl Pts',(-42.9721144255193,29.8537283387532,5.39524314245518));
#11404=CARTESIAN_POINT('Ctrl Pts',(-41.734552781155,32.4178887912006,5.23645842322949));
#11405=CARTESIAN_POINT('Ctrl Pts',(-38.9090367190449,32.768511996884,5.07767370400381));
#11406=CARTESIAN_POINT('Ctrl Pts',(-37.0822795188237,30.5846082029712,4.91888898477813));
#11407=CARTESIAN_POINT('Ctrl Pts',(-37.9266472207506,27.8655052564986,4.76010426555244));
#11408=CARTESIAN_POINT('Ctrl Pts',(-40.6691351419837,27.1004969875778,4.60131954632676));
#11409=CARTESIAN_POINT('Ctrl Pts',(-42.7990408942909,28.9899358291112,4.44253482710108));
#11410=CARTESIAN_POINT('Ctrl Pts',(-42.3664709457677,31.8040717336351,4.28375010787539));
#11411=CARTESIAN_POINT('Ctrl Pts',(-39.7674359385366,32.9666097678519,4.12496538864971));
#11412=CARTESIAN_POINT('Ctrl Pts',(-37.3813094878688,31.4132655655012,3.96618066942403));
#11413=CARTESIAN_POINT('Ctrl Pts',(-37.3925509422966,28.5661000840857,3.80739595019834));
#11414=CARTESIAN_POINT('Ctrl Pts',(-39.7908689363652,27.0316462885214,3.64861123097266));
#11415=CARTESIAN_POINT('Ctrl Pts',(-42.3806429640183,28.2146712816453,3.48982651174698));
#11416=CARTESIAN_POINT('Ctrl Pts',(-42.7909776853917,31.0321352230143,3.33104179252129));
#11417=CARTESIAN_POINT('Ctrl Pts',(-40.6462184384815,32.9046964202063,3.17225707329561));
#11418=CARTESIAN_POINT('Ctrl Pts',(-37.9098568901123,32.1180560230099,3.01347235406992));
#11419=CARTESIAN_POINT('Ctrl Pts',(-37.0869868234582,29.3923703351144,2.85468763484424));
#11420=CARTESIAN_POINT('Ctrl Pts',(-38.9309322151455,27.2229595482945,2.69590291561856));
#11421=CARTESIAN_POINT('Ctrl Pts',(-41.7535914721387,27.5958834596619,2.53711819639287));
#11422=CARTESIAN_POINT('Ctrl Pts',(-42.9708667673923,30.1697362715842,2.37833347716719));
#11423=CARTESIAN_POINT('Ctrl Pts',(-41.4683624873955,32.5881984866867,2.2195487579415));
#11424=CARTESIAN_POINT('Ctrl Pts',(-38.6215968579575,32.6372074308222,2.06076403871582));
#11425=CARTESIAN_POINT('Ctrl Pts',(-37.0367360325092,30.27189715827,1.90197931949014));
#11426=CARTESIAN_POINT('Ctrl Pts',(-38.1646954219365,27.6576682873493,1.74319460026445));
#11427=CARTESIAN_POINT('Ctrl Pts',(-40.9728438312614,27.1878078850814,1.58440988103877));
#11428=CARTESIAN_POINT('Ctrl Pts',(-42.8903737846055,29.2924579583155,1.42562516181309));
#11429=CARTESIAN_POINT('Ctrl Pts',(-42.1618062952702,32.0448609685045,1.2668404425874));
#11430=CARTESIAN_POINT('Ctrl Pts',(-39.4541568081119,32.9252078004982,1.10805572336172));
#11431=CARTESIAN_POINT('Ctrl Pts',(-37.24618588728,31.1276146339126,0.949271004136038));
#11432=CARTESIAN_POINT('Ctrl Pts',(-37.5593499150186,28.2976301780055,0.790486284910354));
#11433=CARTESIAN_POINT('Ctrl Pts',(-40.1067617368674,27.0262943672847,0.63170156568467));
#11434=CARTESIAN_POINT('Ctrl Pts',(-42.556688642221,28.4770230310523,0.472916846458986));
#11435=CARTESIAN_POINT('Ctrl Pts',(-42.665502715148,31.3226388835994,0.314132127233303));
#11436=CARTESIAN_POINT('Ctrl Pts',(-40.3351050257151,32.9561476332342,0.155347408007618));
#11437=CARTESIAN_POINT('Ctrl Pts',(-37.695899841043,31.8858693975142,-0.00343731121806418));
#11438=CARTESIAN_POINT('Ctrl Pts',(-37.1701531156465,29.0839015446546,-0.162222030443749));
#11439=CARTESIAN_POINT('Ctrl Pts',(-38.5409902294193,27.7841423687619,-0.268078509927538));
#11440=CARTESIAN_POINT('Ctrl Pts',(-39.3498000020249,27.5679131979649,-0.321006749669432));
#11441=CARTESIAN_POINT('Ctrl Pts',(-37.9456684496579,31.7564253212269,10.1070022498898));
#11442=CARTESIAN_POINT('Ctrl Pts',(-37.3615552660859,31.0732410562992,10.0540740101479));
#11443=CARTESIAN_POINT('Ctrl Pts',(-36.939116653014,29.0895888807941,9.94821753066413));
#11444=CARTESIAN_POINT('Ctrl Pts',(-39.108275724016,26.9302184094218,9.78943281143844));
#11445=CARTESIAN_POINT('Ctrl Pts',(-42.0942480521154,27.5882785911961,9.63064809221277));
#11446=CARTESIAN_POINT('Ctrl Pts',(-43.1627106713215,30.45077150464,9.47186337298707));
#11447=CARTESIAN_POINT('Ctrl Pts',(-41.3358972179974,32.9023146212042,9.3130786537614));
#11448=CARTESIAN_POINT('Ctrl Pts',(-38.2860249551112,32.6959738611392,9.15429393453571));
#11449=CARTESIAN_POINT('Ctrl Pts',(-36.8053020885911,30.0219455835236,8.99550921531003));
#11450=CARTESIAN_POINT('Ctrl Pts',(-38.2492555806798,27.3276101462363,8.83672449608435));
#11451=CARTESIAN_POINT('Ctrl Pts',(-41.2959950836698,27.0799118123104,8.67793977685866));
#11452=CARTESIAN_POINT('Ctrl Pts',(-43.1562682818588,29.5054517236657,8.51915505763298));
#11453=CARTESIAN_POINT('Ctrl Pts',(-42.1270321175044,32.3837695811262,8.3603703384073));
#11454=CARTESIAN_POINT('Ctrl Pts',(-39.1505321295175,33.0797721595765,8.2015856191816));
#11455=CARTESIAN_POINT('Ctrl Pts',(-36.9517064737084,30.9563010145385,8.04280089995593));
#11456=CARTESIAN_POINT('Ctrl Pts',(-37.5435429208461,27.9573486760775,7.88401618073024));
#11457=CARTESIAN_POINT('Ctrl Pts',(-40.3842253780061,26.8284115903431,7.72523146150456));
#11458=CARTESIAN_POINT('Ctrl Pts',(-42.8731557822249,28.6030104459577,7.56644674227887));
#11459=CARTESIAN_POINT('Ctrl Pts',(-42.7317595632967,31.6565305896485,7.40766202305319));
#11460=CARTESIAN_POINT('Ctrl Pts',(-40.0894825739465,33.19352412848,7.2488773038275));
#11461=CARTESIAN_POINT('Ctrl Pts',(-37.3652857746746,31.8068991895604,7.09009258460182));
#11462=CARTESIAN_POINT('Ctrl Pts',(-37.0531263211737,28.7660878372921,6.93130786537614));
#11463=CARTESIAN_POINT('Ctrl Pts',(-39.438781042777,26.8549027137051,6.77252314615046));
#11464=CARTESIAN_POINT('Ctrl Pts',(-42.3382224477893,27.8230021877797,6.61373842692476));
#11465=CARTESIAN_POINT('Ctrl Pts',(-43.0970598279071,30.7841072034677,6.45495370769909));
#11466=CARTESIAN_POINT('Ctrl Pts',(-41.0205900962205,33.0273750238097,6.2961689884734));
#11467=CARTESIAN_POINT('Ctrl Pts',(-38.0097869908933,32.4991310213199,6.13738426924772));
#11468=CARTESIAN_POINT('Ctrl Pts',(-36.8209910186385,29.6829738515732,5.97859955002204));
#11469=CARTESIAN_POINT('Ctrl Pts',(-38.5425252542124,27.1570488841224,5.81981483079635));
#11470=CARTESIAN_POINT('Ctrl Pts',(-41.5983535432419,27.2337986998063,5.66103011157068));
#11471=CARTESIAN_POINT('Ctrl Pts',(-43.1909155669411,29.8429601105304,5.50224539234498));
#11472=CARTESIAN_POINT('Ctrl Pts',(-41.8622471004298,32.5958889458391,5.34346067311931));
#11473=CARTESIAN_POINT('Ctrl Pts',(-38.8287221762828,32.9723243332319,5.18467595389361));
#11474=CARTESIAN_POINT('Ctrl Pts',(-36.8674827511926,30.6276458939148,5.02589123466794));
#11475=CARTESIAN_POINT('Ctrl Pts',(-37.7740111207489,27.7083680069273,4.86710651544225));
#11476=CARTESIAN_POINT('Ctrl Pts',(-40.7183955377391,26.8870413536941,4.70832179621658));
#11477=CARTESIAN_POINT('Ctrl Pts',(-43.0051007072304,28.915576917623,4.54953707699088));
#11478=CARTESIAN_POINT('Ctrl Pts',(-42.5406858210866,31.9368838996598,4.3907523577652));
#11479=CARTESIAN_POINT('Ctrl Pts',(-39.7503150357662,33.1850056673455,4.23196763853952));
#11480=CARTESIAN_POINT('Ctrl Pts',(-37.1885267106766,31.5173073601942,4.07318291931384));
#11481=CARTESIAN_POINT('Ctrl Pts',(-37.2005957385781,28.4605392296337,3.91439820008815));
#11482=CARTESIAN_POINT('Ctrl Pts',(-39.7754731241996,26.8131220033732,3.75561348086247));
#11483=CARTESIAN_POINT('Ctrl Pts',(-42.5559011550801,28.0832389390561,3.59682876163678));
#11484=CARTESIAN_POINT('Ctrl Pts',(-42.9964439009598,31.1081189613785,3.4380440424111));
#11485=CARTESIAN_POINT('Ctrl Pts',(-40.6937917521916,33.1185343824222,3.27925932318542));
#11486=CARTESIAN_POINT('Ctrl Pts',(-37.7559847194274,32.2739830867363,3.12047460395973));
#11487=CARTESIAN_POINT('Ctrl Pts',(-36.8725365982139,29.3476378500199,2.96168988473406));
#11488=CARTESIAN_POINT('Ctrl Pts',(-38.8522295751747,27.0185193640974,2.80290516550837));
#11489=CARTESIAN_POINT('Ctrl Pts',(-41.8826873819049,27.4188971906877,2.64412044628269));
#11490=CARTESIAN_POINT('Ctrl Pts',(-43.1895760587091,30.1822319176617,2.485335727057));
#11491=CARTESIAN_POINT('Ctrl Pts',(-41.5764604076857,32.7787365017279,2.32655100783132));
#11492=CARTESIAN_POINT('Ctrl Pts',(-38.5201215654086,32.8313533866695,2.16776628860563));
#11493=CARTESIAN_POINT('Ctrl Pts',(-36.8185864441709,30.2919136852476,2.00898156937995));
#11494=CARTESIAN_POINT('Ctrl Pts',(-38.0295839561433,27.4852304942697,1.85019685015426));
#11495=CARTESIAN_POINT('Ctrl Pts',(-41.0444626555158,26.9807799054859,1.69141213092858));
#11496=CARTESIAN_POINT('Ctrl Pts',(-43.1031573429294,29.2403701231382,1.5326274117029));
#11497=CARTESIAN_POINT('Ctrl Pts',(-42.3209541668584,32.1953995581752,1.37384269247722));
#11498=CARTESIAN_POINT('Ctrl Pts',(-39.4139729200365,33.1405557696577,1.21505797325153));
#11499=CARTESIAN_POINT('Ctrl Pts',(-37.0434555798755,31.2106273762437,1.05627325402585));
#11500=CARTESIAN_POINT('Ctrl Pts',(-37.3796741192888,28.1723051040527,0.897488534800164));
#11501=CARTESIAN_POINT('Ctrl Pts',(-40.1146213231896,26.8073760843598,0.738703815574481));
#11502=CARTESIAN_POINT('Ctrl Pts',(-42.7449069653027,28.3649045014615,0.579919096348796));
#11503=CARTESIAN_POINT('Ctrl Pts',(-42.8617317134429,31.4200089225642,0.421134377123114));
#11504=CARTESIAN_POINT('Ctrl Pts',(-40.3597747899385,33.1737733312253,0.262349657897429));
#11505=CARTESIAN_POINT('Ctrl Pts',(-37.5262765787616,32.024703344554,0.103564938671747));
#11506=CARTESIAN_POINT('Ctrl Pts',(-36.9618254271062,29.0164602018976,-0.0552197805539385));
#11507=CARTESIAN_POINT('Ctrl Pts',(-38.4335808375036,27.6210153455288,-0.161076260037727));
#11508=CARTESIAN_POINT('Ctrl Pts',(-39.301933573839,27.3888678140614,-0.214004499779622));
#11509=CARTESIAN_POINT('Ctrl Pts',(-37.8048028959809,31.8768634390788,10.2140044997796));
#11510=CARTESIAN_POINT('Ctrl Pts',(-37.1806370602456,31.1468332160454,10.1610762600377));
#11511=CARTESIAN_POINT('Ctrl Pts',(-36.7292318234001,29.027161972947,10.0552197805539));
#11512=CARTESIAN_POINT('Ctrl Pts',(-39.0471301733659,26.7197234270748,9.89643506132826));
#11513=CARTESIAN_POINT('Ctrl Pts',(-42.2378506810821,27.4229068080925,9.73765034210257));
#11514=CARTESIAN_POINT('Ctrl Pts',(-43.3795778025116,30.4816809153299,9.57886562287688));
#11515=CARTESIAN_POINT('Ctrl Pts',(-41.4274997157721,33.10132639026,9.42008090365121));
#11516=CARTESIAN_POINT('Ctrl Pts',(-38.1684976535193,32.8808368403331,9.26129618442551));
#11517=CARTESIAN_POINT('Ctrl Pts',(-36.5862415917368,30.0234503926053,9.10251146519984));
#11518=CARTESIAN_POINT('Ctrl Pts',(-38.1292070023802,27.144364322879,8.94372674597416));
#11519=CARTESIAN_POINT('Ctrl Pts',(-41.384861491331,26.8796813094609,8.78494202674847));
#11520=CARTESIAN_POINT('Ctrl Pts',(-43.3726936582803,29.4715405389038,8.62615730752279));
#11521=CARTESIAN_POINT('Ctrl Pts',(-42.2728827504615,32.5472247068716,8.4673725882971));
#11522=CARTESIAN_POINT('Ctrl Pts',(-39.0922841014003,33.2909521954307,8.30858786907142));
#11523=CARTESIAN_POINT('Ctrl Pts',(-36.7426849283402,31.0218745933858,8.14980314984573));
#11524=CARTESIAN_POINT('Ctrl Pts',(-37.3751036119715,27.8172840357493,7.99101843062005));
#11525=CARTESIAN_POINT('Ctrl Pts',(-40.4105717195208,26.6109357124657,7.83223371139437));
#11526=CARTESIAN_POINT('Ctrl Pts',(-43.0701681291345,28.5072188455325,7.67344899216868));
#11527=CARTESIAN_POINT('Ctrl Pts',(-42.9190763687717,31.7701189238465,7.51466427294301));
#11528=CARTESIAN_POINT('Ctrl Pts',(-40.0956183957525,33.4125041390164,7.35587955371731));
#11529=CARTESIAN_POINT('Ctrl Pts',(-37.1846233698796,31.9307983015287,7.19709483449163));
#11530=CARTESIAN_POINT('Ctrl Pts',(-36.8510591366849,28.6814784567081,7.03831011526595));
#11531=CARTESIAN_POINT('Ctrl Pts',(-39.4002982481521,26.639243332663,6.87952539604027));
#11532=CARTESIAN_POINT('Ctrl Pts',(-42.4985544057311,27.6737254061808,6.72074067681458));
#11533=CARTESIAN_POINT('Ctrl Pts',(-43.3094252795093,30.8378734493983,6.56195595758889));
#11534=CARTESIAN_POINT('Ctrl Pts',(-41.0905719786276,33.2349621870629,6.40317123836322));
#11535=CARTESIAN_POINT('Ctrl Pts',(-37.8733180468145,32.6704964832245,6.24438651913753));
#11536=CARTESIAN_POINT('Ctrl Pts',(-36.6030063120174,29.6612353625154,6.08560179991185));
#11537=CARTESIAN_POINT('Ctrl Pts',(-38.442586183033,26.9621076717615,5.92681708068616));
#11538=CARTESIAN_POINT('Ctrl Pts',(-41.7079526762557,27.044120223774,5.76803236146049));
#11539=CARTESIAN_POINT('Ctrl Pts',(-43.409716708363,29.8321918823075,5.60924764223479));
#11540=CARTESIAN_POINT('Ctrl Pts',(-41.9899414197044,32.7738891004776,5.45046292300912));
#11541=CARTESIAN_POINT('Ctrl Pts',(-38.7484076335206,33.1761366695798,5.29167820378343));
#11542=CARTESIAN_POINT('Ctrl Pts',(-36.6526859835615,30.6706835848585,5.13289348455775));
#11543=CARTESIAN_POINT('Ctrl Pts',(-37.6213750207472,27.5512307573561,4.97410876533206));
#11544=CARTESIAN_POINT('Ctrl Pts',(-40.7676559334946,26.6735857198104,4.81532404610638));
#11545=CARTESIAN_POINT('Ctrl Pts',(-43.2111605201699,28.8412180061349,4.6565393268807));
#11546=CARTESIAN_POINT('Ctrl Pts',(-42.7149006964056,32.0696960656844,4.49775460765501));
#11547=CARTESIAN_POINT('Ctrl Pts',(-39.7331941329958,33.4034015668391,4.33896988842933));
#11548=CARTESIAN_POINT('Ctrl Pts',(-36.9957439334843,31.6213491548871,4.18018516920365));
#11549=CARTESIAN_POINT('Ctrl Pts',(-37.0086405348597,28.3549783751818,4.02140044997796));
#11550=CARTESIAN_POINT('Ctrl Pts',(-39.760077312034,26.594597718225,3.86261573075228));
#11551=CARTESIAN_POINT('Ctrl Pts',(-42.7311593461418,27.9518065964668,3.7038310115266));
#11552=CARTESIAN_POINT('Ctrl Pts',(-43.2019101165279,31.1841026997428,3.54504629230091));
#11553=CARTESIAN_POINT('Ctrl Pts',(-40.7413650659017,33.3323723446379,3.38626157307523));
#11554=CARTESIAN_POINT('Ctrl Pts',(-37.6021125487425,32.4299101504626,3.22747685384954));
#11555=CARTESIAN_POINT('Ctrl Pts',(-36.6580863729697,29.3029053649254,3.06869213462386));
#11556=CARTESIAN_POINT('Ctrl Pts',(-38.773526935204,26.8140791799003,2.90990741539818));
#11557=CARTESIAN_POINT('Ctrl Pts',(-42.011783291671,27.2419109217134,2.75112269617249));
#11558=CARTESIAN_POINT('Ctrl Pts',(-43.4082853500259,30.1947275637393,2.59233797694681));
#11559=CARTESIAN_POINT('Ctrl Pts',(-41.6845583279759,32.9692745167689,2.43355325772113));
#11560=CARTESIAN_POINT('Ctrl Pts',(-38.4186462728598,33.0254993425169,2.27476853849544));
#11561=CARTESIAN_POINT('Ctrl Pts',(-36.6004368558326,30.3119302122251,2.11598381926976));
#11562=CARTESIAN_POINT('Ctrl Pts',(-37.8944724903502,27.3127927011901,1.95719910004407));
#11563=CARTESIAN_POINT('Ctrl Pts',(-41.1160814797701,26.7737519258905,1.79841438081839));
#11564=CARTESIAN_POINT('Ctrl Pts',(-43.3159409012533,29.1882822879609,1.63962966159271));
#11565=CARTESIAN_POINT('Ctrl Pts',(-42.4801020384466,32.345938147846,1.48084494236703));
#11566=CARTESIAN_POINT('Ctrl Pts',(-39.373789031961,33.3559037388171,1.32206022314134));
#11567=CARTESIAN_POINT('Ctrl Pts',(-36.840725272471,31.2936401185748,1.16327550391566));
#11568=CARTESIAN_POINT('Ctrl Pts',(-37.199998323559,28.0469800300999,1.00449078468998));
#11569=CARTESIAN_POINT('Ctrl Pts',(-40.1224809095117,26.588457801435,0.845706065464291));
#11570=CARTESIAN_POINT('Ctrl Pts',(-42.9331252883845,28.2527859718707,0.686921346238608));
#11571=CARTESIAN_POINT('Ctrl Pts',(-43.0579607117377,31.5173789615289,0.528136627012924));
#11572=CARTESIAN_POINT('Ctrl Pts',(-40.384444554162,33.3913990292165,0.36935190778724));
#11573=CARTESIAN_POINT('Ctrl Pts',(-37.3566533164802,32.1635372915938,0.210567188561557));
#11574=CARTESIAN_POINT('Ctrl Pts',(-36.7534977385659,28.9490188591406,0.0517824693358725));
#11575=CARTESIAN_POINT('Ctrl Pts',(-38.326171445588,27.4578883222956,-0.0540740101479163));
#11576=CARTESIAN_POINT('Ctrl Pts',(-39.254067145653,27.2098224301578,-0.107002249889811));
#11577=CARTESIAN_POINT('Ctrl Pts',(-37.6639373423039,31.9973015569307,10.3210067496694));
#11578=CARTESIAN_POINT('Ctrl Pts',(-36.9997188544053,31.2204253757917,10.2680785099275));
#11579=CARTESIAN_POINT('Ctrl Pts',(-36.5193469937862,28.9647350650998,10.1622220304437));
#11580=CARTESIAN_POINT('Ctrl Pts',(-38.9859846227157,26.5092284447277,10.0034373112181));
#11581=CARTESIAN_POINT('Ctrl Pts',(-42.3814533100487,27.2575350249889,9.84465259199239));
#11582=CARTESIAN_POINT('Ctrl Pts',(-43.5964449337017,30.51259032602,9.6858678727667));
#11583=CARTESIAN_POINT('Ctrl Pts',(-41.5191022135468,33.3003381593159,9.52708315354102));
#11584=CARTESIAN_POINT('Ctrl Pts',(-38.0509703519274,33.065699819527,9.36829843431533));
#11585=CARTESIAN_POINT('Ctrl Pts',(-36.3671810948824,30.024955201687,9.20951371508965));
#11586=CARTESIAN_POINT('Ctrl Pts',(-38.0091584240807,26.9611184995217,9.05072899586397));
#11587=CARTESIAN_POINT('Ctrl Pts',(-41.4737278989921,26.6794508066113,8.89194427663828));
#11588=CARTESIAN_POINT('Ctrl Pts',(-43.5891190347018,29.4376293541419,8.7331595574126));
#11589=CARTESIAN_POINT('Ctrl Pts',(-42.4187333834185,32.7106798326169,8.57437483818692));
#11590=CARTESIAN_POINT('Ctrl Pts',(-39.0340360732831,33.502132231285,8.41559011896122));
#11591=CARTESIAN_POINT('Ctrl Pts',(-36.533663382972,31.0874481722331,8.25680539973555));
#11592=CARTESIAN_POINT('Ctrl Pts',(-37.2066643030969,27.6772193954211,8.09802068050986));
#11593=CARTESIAN_POINT('Ctrl Pts',(-40.4369180610355,26.3934598345883,7.93923596128418));
#11594=CARTESIAN_POINT('Ctrl Pts',(-43.2671804760441,28.4114272451073,7.7804512420585));
#11595=CARTESIAN_POINT('Ctrl Pts',(-43.1063931742466,31.8837072580445,7.62166652283282));
#11596=CARTESIAN_POINT('Ctrl Pts',(-40.1017542175585,33.6314841495529,7.46288180360712));
#11597=CARTESIAN_POINT('Ctrl Pts',(-37.0039609650845,32.0546974134971,7.30409708438145));
#11598=CARTESIAN_POINT('Ctrl Pts',(-36.6489919521961,28.596869076124,7.14531236515576));
#11599=CARTESIAN_POINT('Ctrl Pts',(-39.3618154535272,26.4235839516209,6.98652764593008));
#11600=CARTESIAN_POINT('Ctrl Pts',(-42.6588863636729,27.5244486245819,6.82774292670439));
#11601=CARTESIAN_POINT('Ctrl Pts',(-43.5217907311115,30.8916396953289,6.66895820747871));
#11602=CARTESIAN_POINT('Ctrl Pts',(-41.1605538610348,33.4425493503161,6.51017348825302));
#11603=CARTESIAN_POINT('Ctrl Pts',(-37.7368491027356,32.8418619451291,6.35138876902735));
#11604=CARTESIAN_POINT('Ctrl Pts',(-36.3850216053963,29.6394968734575,6.19260404980166));
#11605=CARTESIAN_POINT('Ctrl Pts',(-38.3426471118536,26.7671664594007,6.03381933057598));
#11606=CARTESIAN_POINT('Ctrl Pts',(-41.8175518092695,26.8544417477417,5.87503461135029));
#11607=CARTESIAN_POINT('Ctrl Pts',(-43.6285178497849,29.8214236540847,5.71624989212461));
#11608=CARTESIAN_POINT('Ctrl Pts',(-42.1176357389792,32.9518892551161,5.55746517289893));
#11609=CARTESIAN_POINT('Ctrl Pts',(-38.6680930907584,33.3799490059277,5.39868045367324));
#11610=CARTESIAN_POINT('Ctrl Pts',(-36.4378892159304,30.7137212758022,5.23989573444757));
#11611=CARTESIAN_POINT('Ctrl Pts',(-37.4687389207455,27.3940935077848,5.08111101522187));
#11612=CARTESIAN_POINT('Ctrl Pts',(-40.81691632925,26.4601300859267,4.92232629599619));
#11613=CARTESIAN_POINT('Ctrl Pts',(-43.4172203331094,28.7668590946468,4.76354157677051));
#11614=CARTESIAN_POINT('Ctrl Pts',(-42.8891155717247,32.2025082317091,4.60475685754482));
#11615=CARTESIAN_POINT('Ctrl Pts',(-39.7160732302253,33.6217974663328,4.44597213831914));
#11616=CARTESIAN_POINT('Ctrl Pts',(-36.802961156292,31.7253909495801,4.28718741909346));
#11617=CARTESIAN_POINT('Ctrl Pts',(-36.8166853311413,28.2494175207298,4.12840269986777));
#11618=CARTESIAN_POINT('Ctrl Pts',(-39.7446814998683,26.3760734330767,3.96961798064209));
#11619=CARTESIAN_POINT('Ctrl Pts',(-42.9064175372036,27.8203742538776,3.81083326141641));
#11620=CARTESIAN_POINT('Ctrl Pts',(-43.407376332096,31.260086438107,3.65204854219072));
#11621=CARTESIAN_POINT('Ctrl Pts',(-40.7889383796118,33.5462103068538,3.49326382296504));
#11622=CARTESIAN_POINT('Ctrl Pts',(-37.4482403780577,32.585837214189,3.33447910373935));
#11623=CARTESIAN_POINT('Ctrl Pts',(-36.4436361477254,29.2581728798308,3.17569438451368));
#11624=CARTESIAN_POINT('Ctrl Pts',(-38.6948242952332,26.6096389957033,3.01690966528799));
#11625=CARTESIAN_POINT('Ctrl Pts',(-42.1408792014373,27.0649246527392,2.85812494606231));
#11626=CARTESIAN_POINT('Ctrl Pts',(-43.6269946413426,30.2072232098169,2.69934022683662));
#11627=CARTESIAN_POINT('Ctrl Pts',(-41.7926562482662,33.15981253181,2.54055550761094));
#11628=CARTESIAN_POINT('Ctrl Pts',(-38.3171709803108,33.2196452983643,2.38177078838525));
#11629=CARTESIAN_POINT('Ctrl Pts',(-36.3822872674944,30.3319467392027,2.22298606915957));
#11630=CARTESIAN_POINT('Ctrl Pts',(-37.7593610245569,27.1403549081105,2.06420134993389));
#11631=CARTESIAN_POINT('Ctrl Pts',(-41.1877003040245,26.566723946295,1.9054166307082));
#11632=CARTESIAN_POINT('Ctrl Pts',(-43.5287244595771,29.1361944527836,1.74663191148252));
#11633=CARTESIAN_POINT('Ctrl Pts',(-42.6392499100348,32.4964767375168,1.58784719225684));
#11634=CARTESIAN_POINT('Ctrl Pts',(-39.3336051438857,33.5712517079766,1.42906247303115));
#11635=CARTESIAN_POINT('Ctrl Pts',(-36.6379949650665,31.3766528609059,1.27027775380547));
#11636=CARTESIAN_POINT('Ctrl Pts',(-37.0203225278291,27.921654956147,1.11149303457979));
#11637=CARTESIAN_POINT('Ctrl Pts',(-40.1303404958339,26.3695395185102,0.952708315354101));
#11638=CARTESIAN_POINT('Ctrl Pts',(-43.1213436114662,28.1406674422797,0.793923596128419));
#11639=CARTESIAN_POINT('Ctrl Pts',(-43.2541897100326,31.6147490004937,0.635138876902735));
#11640=CARTESIAN_POINT('Ctrl Pts',(-40.4091143183855,33.6090247272076,0.476354157677051));
#11641=CARTESIAN_POINT('Ctrl Pts',(-37.1870300541988,32.3023712386336,0.317569438451368));
#11642=CARTESIAN_POINT('Ctrl Pts',(-36.5451700500256,28.8815775163836,0.158784719225683));
#11643=CARTESIAN_POINT('Ctrl Pts',(-38.2187620536724,27.2947612990625,0.0529282397418946));
#11644=CARTESIAN_POINT('Ctrl Pts',(-39.2062007174671,27.0307770462543,0.));
#11645=CARTESIAN_POINT('Ctrl Pts',(-39.2062007174671,27.0307770462543,0.));
#11646=CARTESIAN_POINT('Ctrl Pts',(-39.1131465583677,27.0648166733231,1.22106756688211E-16));
#11647=CARTESIAN_POINT('Ctrl Pts',(-39.0221596232856,27.1036257391105,3.36163846929538E-15));
#11648=CARTESIAN_POINT('Ctrl Pts',(-38.9334476945311,27.1468755170602,3.10862446895044E-15));
#11649=CARTESIAN_POINT('Ctrl Pts',(-38.8427660056612,27.1910856132987,2.84999254446E-15));
#11650=CARTESIAN_POINT('Ctrl Pts',(-38.7544608062646,27.2399364314085,6.47647713978509E-16));
#11651=CARTESIAN_POINT('Ctrl Pts',(-38.6687829655995,27.2931224109893,1.0547118733939E-15));
#11652=CARTESIAN_POINT('Ctrl Pts',(-38.5858335781199,27.3446146567612,1.44881287344555E-15));
#11653=CARTESIAN_POINT('Ctrl Pts',(-38.5053465494816,27.4001712124465,-2.89463008805608E-16));
#11654=CARTESIAN_POINT('Ctrl Pts',(-38.4275832472096,27.4595454790079,-6.10622663543836E-16));
#11655=CARTESIAN_POINT('Ctrl Pts',(-38.3595403577215,27.5114979622491,-8.91637361439786E-16));
#11656=CARTESIAN_POINT('Ctrl Pts',(-38.2935831179973,27.5663740973322,-1.70865430175454E-16));
#11657=CARTESIAN_POINT('Ctrl Pts',(-38.2299118881401,27.6240216579528,-2.77555756156289E-16));
#11658=CARTESIAN_POINT('Ctrl Pts',(-38.2165693475258,27.6361019165031,-2.9991310673269E-16));
#11659=CARTESIAN_POINT('Ctrl Pts',(-38.2033254218291,27.6483057781323,-1.05728990982097E-15));
#11660=CARTESIAN_POINT('Ctrl Pts',(-38.1901991339964,27.6606155381867,-9.99200722162641E-16));
#11661=CARTESIAN_POINT('Ctrl Pts',(-38.1177715281097,27.7285377459838,-6.7867896889854E-16));
#11662=CARTESIAN_POINT('Ctrl Pts',(-38.0488096398962,27.7997811640852,-3.49414594253822E-15));
#11663=CARTESIAN_POINT('Ctrl Pts',(-37.9835528134077,27.8740546235615,-2.692290834716E-15));
#11664=CARTESIAN_POINT('Ctrl Pts',(-37.9186573342444,27.9479168078142,-1.89487584778096E-15));
#11665=CARTESIAN_POINT('Ctrl Pts',(-37.8574255131234,28.024776367863,5.29767817859097E-16));
#11666=CARTESIAN_POINT('Ctrl Pts',(-37.8001363539989,28.1043736902275,1.4432899320127E-15));
#11667=CARTESIAN_POINT('Ctrl Pts',(-37.7442812467117,28.1819785468598,2.33394492634393E-15));
#11668=CARTESIAN_POINT('Ctrl Pts',(-37.6921736179339,28.2621865588976,-1.21793505985174E-15));
#11669=CARTESIAN_POINT('Ctrl Pts',(-37.6441189020832,28.3447712453598,-1.49880108324396E-15));
#11670=CARTESIAN_POINT('Ctrl Pts',(-37.6233913188262,28.3803927433563,-1.61994785897366E-15));
#11671=CARTESIAN_POINT('Ctrl Pts',(-37.6034183971599,28.4164565342063,-1.75461794011481E-15));
#11672=CARTESIAN_POINT('Ctrl Pts',(-37.5842276308026,28.4529447756955,-2.08166817117217E-15));
#11673=CARTESIAN_POINT('Ctrl Pts',(-37.5705623279671,28.47892721228,-2.31455311003352E-15));
#11674=CARTESIAN_POINT('Ctrl Pts',(-37.5572936578702,28.5051248713913,-1.95119937827049E-15));
#11675=CARTESIAN_POINT('Ctrl Pts',(-37.5444321439544,28.531531314607,-2.13717932240343E-15));
#11676=CARTESIAN_POINT('Ctrl Pts',(-37.538816666632,28.543060655866,-2.21838019545243E-15));
#11677=CARTESIAN_POINT('Ctrl Pts',(-37.5332797327988,28.5546280003926,3.28930239803853E-15));
#11678=CARTESIAN_POINT('Ctrl Pts',(-37.5278259127264,28.5662245354477,3.1641356201817E-15));
#11679=CARTESIAN_POINT('Ctrl Pts',(-37.4875980549542,28.6517616005977,2.24089442948892E-15));
#11680=CARTESIAN_POINT('Ctrl Pts',(-37.4518262344481,28.7390118083874,-3.58197140345829E-15));
#11681=CARTESIAN_POINT('Ctrl Pts',(-37.4207614303772,28.8277378411266,-3.21964677141295E-15));
#11682=CARTESIAN_POINT('Ctrl Pts',(-37.3903833360849,28.9145025212636,-2.86533158527601E-15));
#11683=CARTESIAN_POINT('Ctrl Pts',(-37.3645062370121,29.0026791737866,-9.81657689619027E-16));
#11684=CARTESIAN_POINT('Ctrl Pts',(-37.3434139515882,29.0920546900511,2.77555756156289E-16));
#11685=CARTESIAN_POINT('Ctrl Pts',(-37.3396852215853,29.1078546454526,5.00161645507665E-16));
#11686=CARTESIAN_POINT('Ctrl Pts',(-37.3361061566853,29.1236920756746,-4.14690112491889E-16));
#11687=CARTESIAN_POINT('Ctrl Pts',(-37.3326784971319,29.1395658089505,-4.16333634234434E-16));
#11688=CARTESIAN_POINT('Ctrl Pts',(-37.3125675986992,29.2327007987852,-3.98220993782475E-16));
#11689=CARTESIAN_POINT('Ctrl Pts',(-37.2976646715474,29.3270865450837,4.99300212322796E-16));
#11690=CARTESIAN_POINT('Ctrl Pts',(-37.2878912238873,29.4223141487873,1.16573417585641E-15));
#11691=CARTESIAN_POINT('Ctrl Pts',(-37.2846133376322,29.4542522390242,1.38924739299596E-15));
#11692=CARTESIAN_POINT('Ctrl Pts',(-37.2819128543797,29.486284903846,-3.05311331771918E-16));
#11693=CARTESIAN_POINT('Ctrl Pts',(-37.279788037766,29.5183962478047,-3.05311331771918E-16));
#11694=CARTESIAN_POINT('Ctrl Pts',(-37.2785994180604,29.5363592926898,-3.05311331771918E-16));
#11695=CARTESIAN_POINT('Ctrl Pts',(-37.2775909505956,29.5543469531232,1.33873046221551E-15));
#11696=CARTESIAN_POINT('Ctrl Pts',(-37.2767624107733,29.5723564016008,1.38777878078145E-15));
#11697=CARTESIAN_POINT('Ctrl Pts',(-37.2761881456715,29.584838840566,1.42177441610613E-15));
#11698=CARTESIAN_POINT('Ctrl Pts',(-37.2757004320392,29.5973302169591,1.41595233551992E-15));
#11699=CARTESIAN_POINT('Ctrl Pts',(-37.2752993200193,29.6098201091207,1.41553435639707E-15));
#11700=CARTESIAN_POINT('Ctrl Pts',(-37.2723065021044,29.7030109664475,1.41241568793312E-15));
#11701=CARTESIAN_POINT('Ctrl Pts',(-37.2741232733776,29.7962662842263,3.40525005655215E-15));
#11702=CARTESIAN_POINT('Ctrl Pts',(-37.2806105303684,29.8892109312269,3.67761376907083E-15));
#11703=CARTESIAN_POINT('Ctrl Pts',(-37.2871107458397,29.9823412378062,3.95052153586022E-15));
#11704=CARTESIAN_POINT('Ctrl Pts',(-37.2983005079771,30.0751606128563,7.05637141741307E-16));
#11705=CARTESIAN_POINT('Ctrl Pts',(-37.3140909235774,30.1672796708414,1.22124532708767E-15));
#11706=CARTESIAN_POINT('Ctrl Pts',(-37.32965822843,30.2580971321851,1.72956822427593E-15));
#11707=CARTESIAN_POINT('Ctrl Pts',(-37.349697563177,30.3482347740108,1.91557599461872E-15));
#11708=CARTESIAN_POINT('Ctrl Pts',(-37.374166796696,30.4372943327761,1.84574577843932E-15));
#11709=CARTESIAN_POINT('Ctrl Pts',(-37.3836804577095,30.4719207730141,1.81859572469031E-15));
#11710=CARTESIAN_POINT('Ctrl Pts',(-37.3938641977425,30.506383904736,1.42353668742041E-15));
#11711=CARTESIAN_POINT('Ctrl Pts',(-37.4047171072924,30.5406588580658,1.06858966120171E-15));
#11712=CARTESIAN_POINT('Ctrl Pts',(-37.4105213261189,30.5589893645979,8.78761283608898E-16));
#11713=CARTESIAN_POINT('Ctrl Pts',(-37.4165169545494,30.5772660329217,4.70005909401713E-15));
#11714=CARTESIAN_POINT('Ctrl Pts',(-37.4227039491659,30.5954849444668,4.92661467177413E-15));
#11715=CARTESIAN_POINT('Ctrl Pts',(-37.4281525600734,30.6115295293288,5.12613208994136E-15));
#11716=CARTESIAN_POINT('Ctrl Pts',(-37.433750064935,30.6275303950272,2.76438724788175E-15));
#11717=CARTESIAN_POINT('Ctrl Pts',(-37.4394903125654,30.6434684551818,2.87270207621759E-15));
#11718=CARTESIAN_POINT('Ctrl Pts',(-37.4719158032,30.7334993133521,3.48455049773622E-15));
#11719=CARTESIAN_POINT('Ctrl Pts',(-37.5089323379402,30.821651437624,4.98050361397802E-15));
#11720=CARTESIAN_POINT('Ctrl Pts',(-37.5504668820251,30.9074802563227,5.40539835114373E-15));
#11721=CARTESIAN_POINT('Ctrl Pts',(-37.5816177900888,30.9718518703467,5.72406940401801E-15));
#11722=CARTESIAN_POINT('Ctrl Pts',(-37.6153112267555,31.0349160880258,2.99557423021898E-15));
#11723=CARTESIAN_POINT('Ctrl Pts',(-37.6515337488198,31.0964681987463,3.17801340798951E-15));
#11724=CARTESIAN_POINT('Ctrl Pts',(-37.6664655212945,31.1218414212673,3.2532191125533E-15));
#11725=CARTESIAN_POINT('Ctrl Pts',(-37.6818272197272,31.1469574944417,2.59709908762232E-15));
#11726=CARTESIAN_POINT('Ctrl Pts',(-37.6976185603144,31.1718011729578,2.26901830657766E-15));
#11727=CARTESIAN_POINT('Ctrl Pts',(-37.7070512127228,31.18664106465,2.07304558644154E-15));
#11728=CARTESIAN_POINT('Ctrl Pts',(-37.7166324846138,31.2013763450879,7.23090290612832E-15));
#11729=CARTESIAN_POINT('Ctrl Pts',(-37.7263603370399,31.2160016924469,6.80011602582908E-15));
#11730=CARTESIAN_POINT('Ctrl Pts',(-37.7738890060192,31.2874587070981,4.69536297885029E-15));
#11731=CARTESIAN_POINT('Ctrl Pts',(-37.8249264593017,31.3563137429908,3.52571416788317E-15));
#11732=CARTESIAN_POINT('Ctrl Pts',(-37.879438314505,31.4222140867493,2.82412981889024E-15));
#11733=CARTESIAN_POINT('Ctrl Pts',(-37.9310243832669,31.4845773956458,2.16020124162171E-15));
#11734=CARTESIAN_POINT('Ctrl Pts',(-37.9857223942837,31.544294891251,2.53051231403829E-15));
#11735=CARTESIAN_POINT('Ctrl Pts',(-38.0435270002979,31.6010317842403,2.43164863245049E-15));
#11736=CARTESIAN_POINT('Ctrl Pts',(-38.0564929750925,31.6137582635843,2.39949816171156E-15));
#11737=CARTESIAN_POINT('Ctrl Pts',(-38.0696153396013,31.6263346192956,-2.49073063447215E-17));
#11738=CARTESIAN_POINT('Ctrl Pts',(-38.0828908636835,31.6387595214235,-2.77555756156289E-17));
#11739=CARTESIAN_POINT('Ctrl Pts',(-42.5194677947045,29.9980220285566,8.38741669750802));
#11740=CARTESIAN_POINT('Ctrl Pts',(-42.5205892939538,29.8678903777981,8.3956620675864));
#11741=CARTESIAN_POINT('Ctrl Pts',(-42.5113777972944,29.7379179862643,8.40390743766478));
#11742=CARTESIAN_POINT('Ctrl Pts',(-42.4912802970509,29.6096514007085,8.41215280774316));
#11743=CARTESIAN_POINT('Ctrl Pts',(-42.3622714956278,28.7862893773384,8.46508104748506));
#11744=CARTESIAN_POINT('Ctrl Pts',(-41.7847000858182,28.0332158462492,8.51800928722695));
#11745=CARTESIAN_POINT('Ctrl Pts',(-41.0229436280752,27.6951313564435,8.57093752696884));
#11746=CARTESIAN_POINT('Ctrl Pts',(-40.2611871703322,27.3570468666378,8.62386576671074));
#11747=CARTESIAN_POINT('Ctrl Pts',(-39.3152456646558,27.4339514181157,8.67679400645263));
#11748=CARTESIAN_POINT('Ctrl Pts',(-38.6181179828953,27.890667827996,8.72972224619453));
#11749=CARTESIAN_POINT('Ctrl Pts',(-37.9209903011348,28.3473842378763,8.78265048593642));
#11750=CARTESIAN_POINT('Ctrl Pts',(-37.4726764432901,29.1839125061591,8.83557872567832));
#11751=CARTESIAN_POINT('Ctrl Pts',(-37.4783844595774,30.0172883248844,8.88850696542021));
#11752=CARTESIAN_POINT('Ctrl Pts',(-37.4840924758647,30.8506641436097,8.9414352051621));
#11753=CARTESIAN_POINT('Ctrl Pts',(-37.9438223662839,31.6808875127775,8.994363444904));
#11754=CARTESIAN_POINT('Ctrl Pts',(-38.6471443887468,32.1280311923952,9.0472916846459));
#11755=CARTESIAN_POINT('Ctrl Pts',(-39.3504664112097,32.575174872013,9.10021992438779));
#11756=CARTESIAN_POINT('Ctrl Pts',(-40.2973805657162,32.6392388620807,9.15314816412969));
#11757=CARTESIAN_POINT('Ctrl Pts',(-41.0544291129542,32.2906973974148,9.20607640387158));
#11758=CARTESIAN_POINT('Ctrl Pts',(-41.8114776601922,31.9421559327489,9.25900464361347));
#11759=CARTESIAN_POINT('Ctrl Pts',(-42.3786606001618,31.1810090133494,9.31193288335537));
#11760=CARTESIAN_POINT('Ctrl Pts',(-42.4963857173162,30.356066933708,9.36486112309726));
#11761=CARTESIAN_POINT('Ctrl Pts',(-42.5131087222309,30.2388828460158,9.37237964790084));
#11762=CARTESIAN_POINT('Ctrl Pts',(-42.5207623112886,30.1204114632572,9.37989817270443));
#11763=CARTESIAN_POINT('Ctrl Pts',(-42.5197815649842,30.0018165623494,9.38741669750802));
#11764=CARTESIAN_POINT('Ctrl Pts',(-40.7937992825329,27.0307770462543,10.));
#11765=CARTESIAN_POINT('Ctrl Pts',(-41.7812379463276,27.2947612990625,9.94707176025811));
#11766=CARTESIAN_POINT('Ctrl Pts',(-43.4548297940574,28.8815785121496,9.84121528077431));
#11767=CARTESIAN_POINT('Ctrl Pts',(-42.8129700816392,32.3023708276668,9.68243056154864));
#11768=CARTESIAN_POINT('Ctrl Pts',(-39.5908856649077,33.609025071703,9.52364584232295));
#11769=CARTESIAN_POINT('Ctrl Pts',(-36.7458102038522,31.6147488878258,9.36486112309727));
#11770=CARTESIAN_POINT('Ctrl Pts',(-36.8786563309339,28.140667484321,9.20607640387158));
#11771=CARTESIAN_POINT('Ctrl Pts',(-39.869659490377,26.3695393883571,9.0472916846459));
#11772=CARTESIAN_POINT('Ctrl Pts',(-42.9796775476457,27.9216549347271,8.88850696542022));
#11773=CARTESIAN_POINT('Ctrl Pts',(-43.3620051070722,31.3766528780855,8.72972224619453));
#11774=CARTESIAN_POINT('Ctrl Pts',(-40.6663948741839,33.5712517973455,8.57093752696885));
#11775=CARTESIAN_POINT('Ctrl Pts',(-37.3607500279849,32.4964767903705,8.41215280774316));
#11776=CARTESIAN_POINT('Ctrl Pts',(-36.4712754607486,29.1361944352982,8.25336808851748));
#11777=CARTESIAN_POINT('Ctrl Pts',(-38.812299668292,26.5667238666358,8.0945833692918));
#11778=CARTESIAN_POINT('Ctrl Pts',(-42.2406390269471,27.1403548434066,7.93579865006611));
#11779=CARTESIAN_POINT('Ctrl Pts',(-43.6177128150067,30.3319467464472,7.77701393084043));
#11780=CARTESIAN_POINT('Ctrl Pts',(-41.6828290582353,33.2196453721168,7.61822921161475));
#11781=CARTESIAN_POINT('Ctrl Pts',(-38.20734371072,33.1598126039199,7.45944449238906));
#11782=CARTESIAN_POINT('Ctrl Pts',(-36.3730052758037,30.2072232146022,7.30065977316339));
#11783=CARTESIAN_POINT('Ctrl Pts',(-37.859120749627,27.0649245856435,7.14187505393769));
#11784=CARTESIAN_POINT('Ctrl Pts',(-41.305175734599,26.6096389182437,6.98309033471202));
#11785=CARTESIAN_POINT('Ctrl Pts',(-43.5563639335371,29.258172862872,6.82430561548633));
#11786=CARTESIAN_POINT('Ctrl Pts',(-42.551759680255,32.5858372732818,6.66552089626064));
#11787=CARTESIAN_POINT('Ctrl Pts',(-39.211061602359,33.5462103878864,6.50673617703497));
#11788=CARTESIAN_POINT('Ctrl Pts',(-36.5926235900426,31.2600864669024,6.34795145780927));
#11789=CARTESIAN_POINT('Ctrl Pts',(-37.0935823963814,27.8203742040704,6.1891667385836));
#11790=CARTESIAN_POINT('Ctrl Pts',(-40.2553185059661,26.3760733502665,6.0303820193579));
#11791=CARTESIAN_POINT('Ctrl Pts',(-43.1833147416005,28.249417480727,5.87159730013223));
#11792=CARTESIAN_POINT('Ctrl Pts',(-43.1970389167639,31.7253909890071,5.71281258090654));
#11793=CARTESIAN_POINT('Ctrl Pts',(-40.2839267762627,33.6217975490946,5.55402786168086));
#11794=CARTESIAN_POINT('Ctrl Pts',(-37.1108843622561,32.2025082820388,5.39524314245517));
#11795=CARTESIAN_POINT('Ctrl Pts',(-36.5827795888035,28.7668590664683,5.2364584232295));
#11796=CARTESIAN_POINT('Ctrl Pts',(-39.1830836520825,26.460130005037,5.07767370400381));
#11797=CARTESIAN_POINT('Ctrl Pts',(-42.5312611370964,27.3940934482371,4.91888898477813));
#11798=CARTESIAN_POINT('Ctrl Pts',(-43.5621108654676,30.7137212921113,4.76010426555244));
#11799=CARTESIAN_POINT('Ctrl Pts',(-41.331906939677,33.379949083163,4.60131954632676));
#11800=CARTESIAN_POINT('Ctrl Pts',(-37.8823642126307,32.9518893225699,4.44253482710107));
#11801=CARTESIAN_POINT('Ctrl Pts',(-36.3714820672996,29.821423650004,4.2837501078754));
#11802=CARTESIAN_POINT('Ctrl Pts',(-38.1824481491975,26.8544416758625,4.1249653886497));
#11803=CARTESIAN_POINT('Ctrl Pts',(-41.6573529260186,26.767166385527,3.96618066942403));
#11804=CARTESIAN_POINT('Ctrl Pts',(-43.6149784772097,29.6394968652198,3.80739595019834));
#11805=CARTESIAN_POINT('Ctrl Pts',(-42.2631509489798,32.8418620100683,3.64861123097266));
#11806=CARTESIAN_POINT('Ctrl Pts',(-38.8394461124454,33.4425494289825,3.48982651174697));
#11807=CARTESIAN_POINT('Ctrl Pts',(-36.4782091884119,30.8916397157027,3.33104179252129));
#11808=CARTESIAN_POINT('Ctrl Pts',(-37.3411135755689,27.5244485680153,3.17225707329561));
#11809=CARTESIAN_POINT('Ctrl Pts',(-40.6381845610556,26.4235838698918,3.01347235406992));
#11810=CARTESIAN_POINT('Ctrl Pts',(-43.3510081243786,28.5968690440692,2.85468763484424));
#11811=CARTESIAN_POINT('Ctrl Pts',(-42.9960391033767,32.0546974604333,2.69590291561856));
#11812=CARTESIAN_POINT('Ctrl Pts',(-39.8982457801193,33.6314842325659,2.53711819639287));
#11813=CARTESIAN_POINT('Ctrl Pts',(-36.893606754763,31.8837073010328,2.37833347716719));
#11814=CARTESIAN_POINT('Ctrl Pts',(-36.7328194493102,28.4114272089134,2.21954875794151));
#11815=CARTESIAN_POINT('Ctrl Pts',(-39.5630819289538,26.3934597519746,2.06076403871582));
#11816=CARTESIAN_POINT('Ctrl Pts',(-42.7933357607888,27.6772193427188,1.90197931949014));
#11817=CARTESIAN_POINT('Ctrl Pts',(-43.4663366961235,31.0874481963816,1.74319460026445));
#11818=CARTESIAN_POINT('Ctrl Pts',(-40.9659639490253,33.5021323126134,1.58440988103877));
#11819=CARTESIAN_POINT('Ctrl Pts',(-37.5812665608262,32.7106798921575,1.42562516181309));
#11820=CARTESIAN_POINT('Ctrl Pts',(-36.4108808842817,29.4376293456934,1.2668404425874));
#11821=CARTESIAN_POINT('Ctrl Pts',(-38.5262720652766,26.679450722727,1.10805572336172));
#11822=CARTESIAN_POINT('Ctrl Pts',(-41.9908416256376,26.9611184445014,0.949271004136038));
#11823=CARTESIAN_POINT('Ctrl Pts',(-43.6328189794496,30.024955176587,0.790486284910354));
#11824=CARTESIAN_POINT('Ctrl Pts',(-41.9490297104332,33.065699934597,0.63170156568467));
#11825=CARTESIAN_POINT('Ctrl Pts',(-38.4808977151712,33.3003381572967,0.472916846458986));
#11826=CARTESIAN_POINT('Ctrl Pts',(-36.4035550591505,30.5125904676491,0.314132127233303));
#11827=CARTESIAN_POINT('Ctrl Pts',(-37.6185464810465,27.2575347505532,0.155347408007618));
#11828=CARTESIAN_POINT('Ctrl Pts',(-41.0140157220173,26.5092287064619,-0.00343731121806403));
#11829=CARTESIAN_POINT('Ctrl Pts',(-43.4806523136791,28.9647343328049,-0.162222030443749));
#11830=CARTESIAN_POINT('Ctrl Pts',(-43.0002811455948,31.2204253757916,-0.268078509927538));
#11831=CARTESIAN_POINT('Ctrl Pts',(-42.3360626576962,31.9973015569307,-0.321006749669432));
#11832=CARTESIAN_POINT('Ctrl Pts',(-40.7459328543469,27.2098224301578,10.1070022498898));
#11833=CARTESIAN_POINT('Ctrl Pts',(-41.673828554412,27.4578883222956,10.0540740101479));
#11834=CARTESIAN_POINT('Ctrl Pts',(-43.246502114919,28.9490197948615,9.94821753066413));
#11835=CARTESIAN_POINT('Ctrl Pts',(-42.6433468111667,32.1635369054084,9.78943281143844));
#11836=CARTESIAN_POINT('Ctrl Pts',(-39.6155554301386,33.3913993529387,9.63064809221277));
#11837=CARTESIAN_POINT('Ctrl Pts',(-36.9420392073399,31.5173788556549,9.47186337298707));
#11838=CARTESIAN_POINT('Ctrl Pts',(-37.0668746574889,28.2527860113768,9.3130786537614));
#11839=CARTESIAN_POINT('Ctrl Pts',(-39.8775190775307,26.5884576791301,9.1542939345357));
#11840=CARTESIAN_POINT('Ctrl Pts',(-42.8000017473647,28.0469800099716,8.99550921531003));
#11841=CARTESIAN_POINT('Ctrl Pts',(-43.1592747953177,31.2936401347184,8.83672449608433));
#11842=CARTESIAN_POINT('Ctrl Pts',(-40.6262109850188,33.3559038227971,8.67793977685867));
#11843=CARTESIAN_POINT('Ctrl Pts',(-37.5198979033106,32.3459381975126,8.51915505763297));
#11844=CARTESIAN_POINT('Ctrl Pts',(-36.6840590238768,29.1882822715299,8.36037033840731));
#11845=CARTESIAN_POINT('Ctrl Pts',(-38.8839184942158,26.7737518510347,8.20158561918159));
#11846=CARTESIAN_POINT('Ctrl Pts',(-42.1055275580482,27.312792640388,8.04280089995594));
#11847=CARTESIAN_POINT('Ctrl Pts',(-43.3995632216936,30.3119302190328,7.88401618073023));
#11848=CARTESIAN_POINT('Ctrl Pts',(-41.581353763362,33.0254994118221,7.72523146150456));
#11849=CARTESIAN_POINT('Ctrl Pts',(-38.3154416334834,32.9692745845306,7.56644674227887));
#11850=CARTESIAN_POINT('Ctrl Pts',(-36.5917145721166,30.1947275682361,7.4076620230532));
#11851=CARTESIAN_POINT('Ctrl Pts',(-37.988216662344,27.2419108586636,7.2488773038275));
#11852=CARTESIAN_POINT('Ctrl Pts',(-41.2264730928294,26.8140791071116,7.09009258460183));
#11853=CARTESIAN_POINT('Ctrl Pts',(-43.3419137033927,29.3029053489892,6.93130786537614));
#11854=CARTESIAN_POINT('Ctrl Pts',(-42.3978875060538,32.4299102059921,6.77252314615045));
#11855=CARTESIAN_POINT('Ctrl Pts',(-39.2586349171563,33.3323724207843,6.61373842692477));
#11856=CARTESIAN_POINT('Ctrl Pts',(-36.7980898103057,31.1841027268018,6.45495370769909));
#11857=CARTESIAN_POINT('Ctrl Pts',(-37.268840591448,27.951806549663,6.29616898847341));
#11858=CARTESIAN_POINT('Ctrl Pts',(-40.2399226934486,26.5945976404082,6.13738426924772));
#11859=CARTESIAN_POINT('Ctrl Pts',(-42.9913595334959,28.3549783375912,5.97859955002203));
#11860=CARTESIAN_POINT('Ctrl Pts',(-43.0042561351662,31.6213491919367,5.81981483079636));
#11861=CARTESIAN_POINT('Ctrl Pts',(-40.2668058731011,33.4034016446103,5.66103011157067));
#11862=CARTESIAN_POINT('Ctrl Pts',(-37.2850992415561,32.0696961129792,5.50224539234499));
#11863=CARTESIAN_POINT('Ctrl Pts',(-36.7888394064517,28.8412179796556,5.3434606731193));
#11864=CARTESIAN_POINT('Ctrl Pts',(-39.2323440489636,26.6735856437984,5.18467595389362));
#11865=CARTESIAN_POINT('Ctrl Pts',(-42.3786250336068,27.5512307013991,5.02589123466794));
#11866=CARTESIAN_POINT('Ctrl Pts',(-43.3473140929281,30.6706836001842,4.86710651544225));
#11867=CARTESIAN_POINT('Ctrl Pts',(-41.2515923950797,33.1761367421578,4.70832179621657));
#11868=CARTESIAN_POINT('Ctrl Pts',(-38.0100585348234,32.7738891638639,4.54953707699088));
#11869=CARTESIAN_POINT('Ctrl Pts',(-36.5902832137214,29.8321918784729,4.39075235776521));
#11870=CARTESIAN_POINT('Ctrl Pts',(-38.2920472847157,27.0441201562291,4.23196763853951));
#11871=CARTESIAN_POINT('Ctrl Pts',(-41.5574138525555,26.9621076023424,4.07318291931384));
#11872=CARTESIAN_POINT('Ctrl Pts',(-43.3969937656074,29.6612353547743,3.91439820008815));
#11873=CARTESIAN_POINT('Ctrl Pts',(-42.1266820017825,32.6704965442478,3.75561348086247));
#11874=CARTESIAN_POINT('Ctrl Pts',(-38.9094279964517,33.2349622609857,3.59682876163679));
#11875=CARTESIAN_POINT('Ctrl Pts',(-36.6905746448669,30.8378734685435,3.4380440424111));
#11876=CARTESIAN_POINT('Ctrl Pts',(-37.5014455371744,27.6737253530252,3.27925932318542));
#11877=CARTESIAN_POINT('Ctrl Pts',(-40.5997017655514,26.6392432558621,3.12047460395973));
#11878=CARTESIAN_POINT('Ctrl Pts',(-43.1489409352723,28.6814784265862,2.96168988473405));
#11879=CARTESIAN_POINT('Ctrl Pts',(-42.8153766944534,31.9307983456346,2.80290516550837));
#11880=CARTESIAN_POINT('Ctrl Pts',(-39.9043816020653,33.4125042170238,2.64412044628269));
#11881=CARTESIAN_POINT('Ctrl Pts',(-37.0809235645186,31.7701189642425,2.485335727057));
#11882=CARTESIAN_POINT('Ctrl Pts',(-36.929831800721,28.5072188115211,2.32655100783132));
#11883=CARTESIAN_POINT('Ctrl Pts',(-39.5894282710721,26.6109356348337,2.16776628860563));
#11884=CARTESIAN_POINT('Ctrl Pts',(-42.6248964480619,27.817283986225,2.00898156937995));
#11885=CARTESIAN_POINT('Ctrl Pts',(-43.2573151459858,31.0218746160781,1.85019685015426));
#11886=CARTESIAN_POINT('Ctrl Pts',(-40.9077159195629,33.290952271855,1.69141213092858));
#11887=CARTESIAN_POINT('Ctrl Pts',(-37.7271171971453,32.5472247628218,1.5326274117029));
#11888=CARTESIAN_POINT('Ctrl Pts',(-36.6273062655885,29.4715405309648,1.37384269247722));
#11889=CARTESIAN_POINT('Ctrl Pts',(-38.6151384750923,26.8796812306348,1.21505797325153));
#11890=CARTESIAN_POINT('Ctrl Pts',(-41.8707930443401,27.1443642711765,1.05627325402585));
#11891=CARTESIAN_POINT('Ctrl Pts',(-43.413758478113,30.0234503690188,0.897488534800164));
#11892=CARTESIAN_POINT('Ctrl Pts',(-41.831502405081,32.8808369484644,0.738703815574481));
#11893=CARTESIAN_POINT('Ctrl Pts',(-38.5725002172442,33.1013263883626,0.579919096348796));
#11894=CARTESIAN_POINT('Ctrl Pts',(-36.6204221907717,30.4816810484188,0.421134377123114));
#11895=CARTESIAN_POINT('Ctrl Pts',(-37.7621491226102,27.4229065502053,0.262349657897428));
#11896=CARTESIAN_POINT('Ctrl Pts',(-40.9528701505796,26.7197236730263,0.103564938671747));
#11897=CARTESIAN_POINT('Ctrl Pts',(-43.2707675258253,29.0271612848097,-0.0552197805539385));
#11898=CARTESIAN_POINT('Ctrl Pts',(-42.8193629397544,31.1468332160454,-0.161076260037727));
#11899=CARTESIAN_POINT('Ctrl Pts',(-42.1951971040191,31.8768634390788,-0.214004499779622));
#11900=CARTESIAN_POINT('Ctrl Pts',(-40.698066426161,27.3888678140614,10.2140044997796));
#11901=CARTESIAN_POINT('Ctrl Pts',(-41.5664191624963,27.6210153455288,10.1610762600377));
#11902=CARTESIAN_POINT('Ctrl Pts',(-43.0381744357806,29.0164610775733,10.0552197805539));
#11903=CARTESIAN_POINT('Ctrl Pts',(-42.4737235406942,32.0247029831501,9.89643506132824));
#11904=CARTESIAN_POINT('Ctrl Pts',(-39.6402251953695,33.1737736341743,9.73765034210259));
#11905=CARTESIAN_POINT('Ctrl Pts',(-37.1382682108276,31.4200088234841,9.57886562287687));
#11906=CARTESIAN_POINT('Ctrl Pts',(-37.2550929840439,28.3649045384325,9.42008090365121));
#11907=CARTESIAN_POINT('Ctrl Pts',(-39.8853786646844,26.8073759699033,9.26129618442551));
#11908=CARTESIAN_POINT('Ctrl Pts',(-42.6203259470837,28.172305085216,9.10251146519984));
#11909=CARTESIAN_POINT('Ctrl Pts',(-42.9565444835633,31.2106273913515,8.94372674597415));
#11910=CARTESIAN_POINT('Ctrl Pts',(-40.5860270958538,33.1405558482486,8.78494202674847));
#11911=CARTESIAN_POINT('Ctrl Pts',(-37.6790457786362,32.1953996046547,8.62615730752278));
#11912=CARTESIAN_POINT('Ctrl Pts',(-36.896842587005,29.2403701077616,8.46737258829711));
#11913=CARTESIAN_POINT('Ctrl Pts',(-38.9555373201395,26.9807798354337,8.30858786907141));
#11914=CARTESIAN_POINT('Ctrl Pts',(-41.9704160891492,27.4852304373692,8.14980314984574));
#11915=CARTESIAN_POINT('Ctrl Pts',(-43.1814136283805,30.2919136916184,7.99101843062005));
#11916=CARTESIAN_POINT('Ctrl Pts',(-41.4798784684888,32.8313534515275,7.83223371139437));
#11917=CARTESIAN_POINT('Ctrl Pts',(-38.4235395562468,32.7787365651412,7.67344899216869));
#11918=CARTESIAN_POINT('Ctrl Pts',(-36.8104238684295,30.18223192187,7.514664272943));
#11919=CARTESIAN_POINT('Ctrl Pts',(-38.117312575061,27.4188971316837,7.35587955371732));
#11920=CARTESIAN_POINT('Ctrl Pts',(-41.1477704510597,27.0185192959796,7.19709483449164));
#11921=CARTESIAN_POINT('Ctrl Pts',(-43.1274634732482,29.3476378351063,7.03831011526595));
#11922=CARTESIAN_POINT('Ctrl Pts',(-42.2440153318527,32.2739831387024,6.87952539604027));
#11923=CARTESIAN_POINT('Ctrl Pts',(-39.3062082319536,33.1185344536822,6.72074067681459));
#11924=CARTESIAN_POINT('Ctrl Pts',(-37.0035560305689,31.1081189867012,6.5619559575889));
#11925=CARTESIAN_POINT('Ctrl Pts',(-37.4440987865146,28.0832388952556,6.40317123836322));
#11926=CARTESIAN_POINT('Ctrl Pts',(-40.2245268809313,26.81312193055,6.24438651913753));
#11927=CARTESIAN_POINT('Ctrl Pts',(-42.7994043253911,28.4605391944553,6.08560179991184));
#11928=CARTESIAN_POINT('Ctrl Pts',(-42.8114733535686,31.5173073948663,5.92681708068617));
#11929=CARTESIAN_POINT('Ctrl Pts',(-40.2496849699394,33.1850057401262,5.76803236146048));
#11930=CARTESIAN_POINT('Ctrl Pts',(-37.4593141208561,31.9368839439196,5.6092476422348));
#11931=CARTESIAN_POINT('Ctrl Pts',(-36.9948992240999,28.9155768928429,5.45046292300912));
#11932=CARTESIAN_POINT('Ctrl Pts',(-39.2816044458447,26.8870412825597,5.29167820378343));
#11933=CARTESIAN_POINT('Ctrl Pts',(-42.2259889301172,27.7083679545611,5.13289348455775));
#11934=CARTESIAN_POINT('Ctrl Pts',(-43.1325173203886,30.6276459082571,4.97410876533206));
#11935=CARTESIAN_POINT('Ctrl Pts',(-41.1712778504822,32.9723244011526,4.81532404610638));
#11936=CARTESIAN_POINT('Ctrl Pts',(-38.137752857016,32.5958890051579,4.6565393268807));
#11937=CARTESIAN_POINT('Ctrl Pts',(-36.8090843601431,29.8429601069419,4.49775460765501));
#11938=CARTESIAN_POINT('Ctrl Pts',(-38.401646420234,27.2337986365958,4.33896988842933));
#11939=CARTESIAN_POINT('Ctrl Pts',(-41.4574747790924,27.1570488191579,4.18018516920364));
#11940=CARTESIAN_POINT('Ctrl Pts',(-43.1790090540052,29.6829738443289,4.02140044997797));
#11941=CARTESIAN_POINT('Ctrl Pts',(-41.9902130545851,32.4991310784273,3.86261573075228));
#11942=CARTESIAN_POINT('Ctrl Pts',(-38.9794098804581,33.027375092989,3.7038310115266));
#11943=CARTESIAN_POINT('Ctrl Pts',(-36.9029401013218,30.7841072213844,3.54504629230091));
#11944=CARTESIAN_POINT('Ctrl Pts',(-37.66177749878,27.823002138035,3.38626157307523));
#11945=CARTESIAN_POINT('Ctrl Pts',(-40.5612189700471,26.8549026418326,3.22747685384954));
#11946=CARTESIAN_POINT('Ctrl Pts',(-42.946873746166,28.7660878091031,3.06869213462386));
#11947=CARTESIAN_POINT('Ctrl Pts',(-42.6347142855301,31.806899230836,2.90990741539817));
#11948=CARTESIAN_POINT('Ctrl Pts',(-39.9105174240114,33.1935242014816,2.7511226961725));
#11949=CARTESIAN_POINT('Ctrl Pts',(-37.2682403742742,31.6565306274523,2.59233797694681));
#11950=CARTESIAN_POINT('Ctrl Pts',(-37.1268441521318,28.6030104141288,2.43355325772113));
#11951=CARTESIAN_POINT('Ctrl Pts',(-39.6157746131904,26.8284115176927,2.27476853849544));
#11952=CARTESIAN_POINT('Ctrl Pts',(-42.456457135335,27.9573486297311,2.11598381926976));
#11953=CARTESIAN_POINT('Ctrl Pts',(-43.0482935958481,30.9563010357746,1.95719910004407));
#11954=CARTESIAN_POINT('Ctrl Pts',(-40.8494678901005,33.0797722310966,1.79841438081839));
#11955=CARTESIAN_POINT('Ctrl Pts',(-37.8729678334645,32.3837696334862,1.63962966159271));
#11956=CARTESIAN_POINT('Ctrl Pts',(-36.8437316468953,29.5054517162361,1.48084494236703));
#11957=CARTESIAN_POINT('Ctrl Pts',(-38.7040048849081,27.0799117385426,1.32206022314134));
#11958=CARTESIAN_POINT('Ctrl Pts',(-41.7507444630425,27.3276100978515,1.16327550391566));
#11959=CARTESIAN_POINT('Ctrl Pts',(-43.1946979767764,30.0219455614506,1.00449078468998));
#11960=CARTESIAN_POINT('Ctrl Pts',(-41.7139750997287,32.6959739623317,0.84570606546429));
#11961=CARTESIAN_POINT('Ctrl Pts',(-38.6641027193173,32.9023146194285,0.686921346238608));
#11962=CARTESIAN_POINT('Ctrl Pts',(-36.8372893223927,30.4507716291885,0.528136627012924));
#11963=CARTESIAN_POINT('Ctrl Pts',(-37.9057517641739,27.5882783498574,0.369351907787239));
#11964=CARTESIAN_POINT('Ctrl Pts',(-40.8917245791419,26.9302186395907,0.210567188561557));
#11965=CARTESIAN_POINT('Ctrl Pts',(-43.0608827379715,29.0895882368145,0.0517824693358725));
#11966=CARTESIAN_POINT('Ctrl Pts',(-42.6384447339141,31.0732410562992,-0.0540740101479163));
#11967=CARTESIAN_POINT('Ctrl Pts',(-42.0543315503421,31.7564253212269,-0.107002249889811));
#11968=CARTESIAN_POINT('Ctrl Pts',(-40.6501999979751,27.5679131979649,10.3210067496694));
#11969=CARTESIAN_POINT('Ctrl Pts',(-41.4590097705807,27.7841423687619,10.2680785099275));
#11970=CARTESIAN_POINT('Ctrl Pts',(-42.8298467566421,29.0839023602852,10.1622220304438));
#11971=CARTESIAN_POINT('Ctrl Pts',(-42.3041002702218,31.8858690608918,10.0034373112181));
#11972=CARTESIAN_POINT('Ctrl Pts',(-39.6648949606003,32.95614791541,9.8446525919924));
#11973=CARTESIAN_POINT('Ctrl Pts',(-37.3344972143153,31.3226387913133,9.68586787276669));
#11974=CARTESIAN_POINT('Ctrl Pts',(-37.443311310599,28.4770230654882,9.52708315354102));
#11975=CARTESIAN_POINT('Ctrl Pts',(-39.893238251838,27.0262942606764,9.36829843431533));
#11976=CARTESIAN_POINT('Ctrl Pts',(-42.4406501468027,28.2976301604605,9.20951371508965));
#11977=CARTESIAN_POINT('Ctrl Pts',(-42.7538141718088,31.1276146479845,9.05072899586396));
#11978=CARTESIAN_POINT('Ctrl Pts',(-40.5458432066888,32.9252078737001,8.89194427663828));
#11979=CARTESIAN_POINT('Ctrl Pts',(-37.8381936539619,32.0448610117969,8.7331595574126));
#11980=CARTESIAN_POINT('Ctrl Pts',(-37.1096261501333,29.2924579439933,8.57437483818691));
#11981=CARTESIAN_POINT('Ctrl Pts',(-39.0271561460632,27.1878078198326,8.41559011896123));
#11982=CARTESIAN_POINT('Ctrl Pts',(-41.8353046202503,27.6576682343505,8.25680539973555));
#11983=CARTESIAN_POINT('Ctrl Pts',(-42.9632640350674,30.271897164204,8.09802068050986));
#11984=CARTESIAN_POINT('Ctrl Pts',(-41.3784031736155,32.6372074912328,7.93923596128418));
#11985=CARTESIAN_POINT('Ctrl Pts',(-38.5316374790102,32.5881985457519,7.78045124205849));
#11986=CARTESIAN_POINT('Ctrl Pts',(-37.0291331647424,30.1697362755039,7.62166652283281));
#11987=CARTESIAN_POINT('Ctrl Pts',(-38.246408487778,27.5958834047039,7.46288180360713));
#11988=CARTESIAN_POINT('Ctrl Pts',(-41.0690678092901,27.2229594848474,7.30409708438144));
#11989=CARTESIAN_POINT('Ctrl Pts',(-42.9130132431038,29.3923703212235,7.14531236515576));
#11990=CARTESIAN_POINT('Ctrl Pts',(-42.0901431576515,32.1180560714127,6.98652764593008));
#11991=CARTESIAN_POINT('Ctrl Pts',(-39.3537815467508,32.9046964865801,6.8277429267044));
#11992=CARTESIAN_POINT('Ctrl Pts',(-37.209022250832,31.0321352466005,6.66895820747871));
#11993=CARTESIAN_POINT('Ctrl Pts',(-37.6193569815813,28.2146712408483,6.51017348825303));
#11994=CARTESIAN_POINT('Ctrl Pts',(-40.2091310684138,27.0316462206917,6.35138876902734));
#11995=CARTESIAN_POINT('Ctrl Pts',(-42.6074491172863,28.5661000513194,6.19260404980166));
#11996=CARTESIAN_POINT('Ctrl Pts',(-42.618690571971,31.4132655977958,6.03381933057598));
#11997=CARTESIAN_POINT('Ctrl Pts',(-40.2325640667778,32.966609835642,5.8750346113503));
#11998=CARTESIAN_POINT('Ctrl Pts',(-37.6335290001561,31.8040717748601,5.7162498921246));
#11999=CARTESIAN_POINT('Ctrl Pts',(-37.2009590417481,28.9899358060303,5.55746517289893));
#12000=CARTESIAN_POINT('Ctrl Pts',(-39.3308648427259,27.1004969213211,5.39868045367324));
#12001=CARTESIAN_POINT('Ctrl Pts',(-42.0733528266276,27.8655052077231,5.23989573444756));
#12002=CARTESIAN_POINT('Ctrl Pts',(-42.9177205478493,30.58460821633,5.08111101522188));
#12003=CARTESIAN_POINT('Ctrl Pts',(-41.0909633058848,32.7685120601473,4.92232629599619));
#12004=CARTESIAN_POINT('Ctrl Pts',(-38.2654471792087,32.4178888464519,4.76354157677051));
#12005=CARTESIAN_POINT('Ctrl Pts',(-37.0278855065648,29.8537283354108,4.60475685754482));
#12006=CARTESIAN_POINT('Ctrl Pts',(-38.5112455557523,27.4234771169624,4.44597213831914));
#12007=CARTESIAN_POINT('Ctrl Pts',(-41.3575357056293,27.3519900359734,4.28718741909345));
#12008=CARTESIAN_POINT('Ctrl Pts',(-42.9610243424029,29.7047123338834,4.12840269986777));
#12009=CARTESIAN_POINT('Ctrl Pts',(-41.8537441073879,32.3277656126068,3.96961798064209));
#12010=CARTESIAN_POINT('Ctrl Pts',(-39.0493917644644,32.8197879249922,3.81083326141641));
#12011=CARTESIAN_POINT('Ctrl Pts',(-37.1153055577768,30.7303409742253,3.65204854219072));
#12012=CARTESIAN_POINT('Ctrl Pts',(-37.8221094603855,27.9722789230449,3.49326382296504));
#12013=CARTESIAN_POINT('Ctrl Pts',(-40.5227361745428,27.070562027803,3.33447910373935));
#12014=CARTESIAN_POINT('Ctrl Pts',(-42.7448065570598,28.85069719162,3.17569438451367));
#12015=CARTESIAN_POINT('Ctrl Pts',(-42.4540518766068,31.6830001160374,3.01690966528799));
#12016=CARTESIAN_POINT('Ctrl Pts',(-39.9166532459575,32.9745441859394,2.8581249460623));
#12017=CARTESIAN_POINT('Ctrl Pts',(-37.4555571840299,31.5429422906621,2.69934022683662));
#12018=CARTESIAN_POINT('Ctrl Pts',(-37.3238565035427,28.6988020167365,2.54055550761094));
#12019=CARTESIAN_POINT('Ctrl Pts',(-39.6421209553087,27.0458874005518,2.38177078838525));
#12020=CARTESIAN_POINT('Ctrl Pts',(-42.288017822608,28.0974132732372,2.22298606915957));
#12021=CARTESIAN_POINT('Ctrl Pts',(-42.8392720457105,30.8907274554712,2.06420134993389));
#12022=CARTESIAN_POINT('Ctrl Pts',(-40.7912198606381,32.8685921903381,1.9054166307082));
#12023=CARTESIAN_POINT('Ctrl Pts',(-38.0188184697836,32.2203145041505,1.74663191148252));
#12024=CARTESIAN_POINT('Ctrl Pts',(-37.0601570282021,29.5393629015074,1.58784719225684));
#12025=CARTESIAN_POINT('Ctrl Pts',(-38.7928712947239,27.2801422464504,1.42906247303115));
#12026=CARTESIAN_POINT('Ctrl Pts',(-41.6306958817449,27.5108559245266,1.27027775380547));
#12027=CARTESIAN_POINT('Ctrl Pts',(-42.9756374754398,30.0204407538824,1.11149303457979));
#12028=CARTESIAN_POINT('Ctrl Pts',(-41.5964477943764,32.5111109761991,0.952708315354102));
#12029=CARTESIAN_POINT('Ctrl Pts',(-38.7557052213904,32.7033028504944,0.793923596128418));
#12030=CARTESIAN_POINT('Ctrl Pts',(-37.0541564540138,30.4198622099582,0.635138876902736));
#12031=CARTESIAN_POINT('Ctrl Pts',(-38.0493544057376,27.7536501495095,0.47635415767705));
#12032=CARTESIAN_POINT('Ctrl Pts',(-40.8305790077041,27.1407136061552,0.317569438451368));
#12033=CARTESIAN_POINT('Ctrl Pts',(-42.8509979501178,29.1520151888193,0.158784719225683));
#12034=CARTESIAN_POINT('Ctrl Pts',(-42.4575265280738,30.9996488965529,0.0529282397418946));
#12035=CARTESIAN_POINT('Ctrl Pts',(-41.9134659966651,31.635987203375,0.));
#12036=CARTESIAN_POINT('Ctrl Pts',(-41.9134659966651,31.635987203375,0.));
#12037=CARTESIAN_POINT('Ctrl Pts',(-41.9750787519721,31.5780863425442,-1.96186115810562E-16));
#12038=CARTESIAN_POINT('Ctrl Pts',(-42.0333203309463,31.5170349684915,2.22103875014277E-15));
#12039=CARTESIAN_POINT('Ctrl Pts',(-42.0881938461448,31.4532178794343,1.66533453693773E-15));
#12040=CARTESIAN_POINT('Ctrl Pts',(-42.1445200426994,31.38771134338,1.09491901633508E-15));
#12041=CARTESIAN_POINT('Ctrl Pts',(-42.1972979235958,31.3192902871514,-1.47257027708725E-15));
#12042=CARTESIAN_POINT('Ctrl Pts',(-42.246505305796,31.2483223318251,-1.38777878078145E-15));
#12043=CARTESIAN_POINT('Ctrl Pts',(-42.297406955068,31.1749108677304,-1.30006781520595E-15));
#12044=CARTESIAN_POINT('Ctrl Pts',(-42.3444885826855,31.0987735779648,5.02613438679333E-16));
#12045=CARTESIAN_POINT('Ctrl Pts',(-42.3876907051178,31.0202733855454,1.22124532708767E-15));
#12046=CARTESIAN_POINT('Ctrl Pts',(-42.406591633682,30.9859295513619,1.53564677826632E-15));
#12047=CARTESIAN_POINT('Ctrl Pts',(-42.4247495066867,30.9511329365615,1.10529844948776E-15));
#12048=CARTESIAN_POINT('Ctrl Pts',(-42.4421568977288,30.915911843557,1.60982338570648E-15));
#12049=CARTESIAN_POINT('Ctrl Pts',(-42.4516651170732,30.8966734707859,1.88540366920346E-15));
#12050=CARTESIAN_POINT('Ctrl Pts',(-42.460949400319,30.8773084338143,1.31566465613105E-15));
#12051=CARTESIAN_POINT('Ctrl Pts',(-42.4700083335416,30.8578212163121,1.60982338570648E-15));
#12052=CARTESIAN_POINT('Ctrl Pts',(-42.4786583063457,30.8392137382265,1.89070248574673E-15));
#12053=CARTESIAN_POINT('Ctrl Pts',(-42.4871053067842,30.8204888630385,-2.805315957825E-15));
#12054=CARTESIAN_POINT('Ctrl Pts',(-42.4953340038778,30.8016832742127,-2.66453525910038E-15));
#12055=CARTESIAN_POINT('Ctrl Pts',(-42.5318948097226,30.718128432658,-2.0390345590246E-15));
#12056=CARTESIAN_POINT('Ctrl Pts',(-42.5641953969086,30.6328901298495,1.3017395342382E-15));
#12057=CARTESIAN_POINT('Ctrl Pts',(-42.59221149408,30.5463672129356,6.66133814775094E-16));
#12058=CARTESIAN_POINT('Ctrl Pts',(-42.6206898803926,30.4584165952001,2.00400669355727E-17));
#12059=CARTESIAN_POINT('Ctrl Pts',(-42.6447417066998,30.3691378634739,-3.20845694331531E-15));
#12060=CARTESIAN_POINT('Ctrl Pts',(-42.6643023724568,30.2789128079137,-3.3584246494911E-15));
#12061=CARTESIAN_POINT('Ctrl Pts',(-42.6835247634633,30.190248070317,-3.50579887091441E-15));
#12062=CARTESIAN_POINT('Ctrl Pts',(-42.6984102463557,30.1006685472939,-1.83791489597701E-16));
#12063=CARTESIAN_POINT('Ctrl Pts',(-42.7088548140498,30.0105137169402,6.66133814775094E-16));
#12064=CARTESIAN_POINT('Ctrl Pts',(-42.7129849619528,29.9748633392087,1.00222405004665E-15));
#12065=CARTESIAN_POINT('Ctrl Pts',(-42.7164201926426,29.9391228204044,-2.39044314140577E-15));
#12066=CARTESIAN_POINT('Ctrl Pts',(-42.7191520459164,29.9033126170804,-2.52575738102223E-15));
#12067=CARTESIAN_POINT('Ctrl Pts',(-42.720768952831,29.8821175675802,-2.60584606359175E-15));
#12068=CARTESIAN_POINT('Ctrl Pts',(-42.7221394354625,29.8608981026457,-3.21666721681218E-15));
#12069=CARTESIAN_POINT('Ctrl Pts',(-42.723261537278,29.8396584408921,-3.41393580072236E-15));
#12070=CARTESIAN_POINT('Ctrl Pts',(-42.7240084444107,29.8255206374949,-3.54524412795088E-15));
#12071=CARTESIAN_POINT('Ctrl Pts',(-42.724645223022,29.8113738891061,-3.12269885146989E-15));
#12072=CARTESIAN_POINT('Ctrl Pts',(-42.7251709450439,29.7972339960158,-3.08086889333481E-15));
#12073=CARTESIAN_POINT('Ctrl Pts',(-42.7287097000643,29.702055145649,-2.7993018899111E-15));
#12074=CARTESIAN_POINT('Ctrl Pts',(-42.7272297226826,29.6070253269581,6.43470337153603E-17));
#12075=CARTESIAN_POINT('Ctrl Pts',(-42.7206723647361,29.5125432621922,-2.77555756156289E-16));
#12076=CARTESIAN_POINT('Ctrl Pts',(-42.714137496433,29.4183852407328,-6.18285928655555E-16));
#12077=CARTESIAN_POINT('Ctrl Pts',(-42.7025603747006,29.3247702689567,-2.49368351834607E-15));
#12078=CARTESIAN_POINT('Ctrl Pts',(-42.6858349550881,29.2320750778189,-1.77635683940025E-15));
#12079=CARTESIAN_POINT('Ctrl Pts',(-42.6838980906665,29.221340637552,-1.69328780105545E-15));
#12080=CARTESIAN_POINT('Ctrl Pts',(-42.6818921284449,29.2106185215464,-4.13712221908638E-15));
#12081=CARTESIAN_POINT('Ctrl Pts',(-42.6798168585049,29.1999093083932,-4.21884749357559E-15));
#12082=CARTESIAN_POINT('Ctrl Pts',(-42.6622719337603,29.1093705619761,-4.96218911960519E-15));
#12083=CARTESIAN_POINT('Ctrl Pts',(-42.6397776265129,29.019753739261,6.15786555997277E-16));
#12084=CARTESIAN_POINT('Ctrl Pts',(-42.6126092292143,28.9312967674749,6.10622663543836E-16));
#12085=CARTESIAN_POINT('Ctrl Pts',(-42.6018609497875,28.8963016869939,6.08579739980496E-16));
#12086=CARTESIAN_POINT('Ctrl Pts',(-42.5903805354635,28.8614881887874,-1.38856776536099E-15));
#12087=CARTESIAN_POINT('Ctrl Pts',(-42.5781828380702,28.8268713474415,-1.41553435639707E-15));
#12088=CARTESIAN_POINT('Ctrl Pts',(-42.5722285540192,28.8099731985799,-1.42869804932521E-15));
#12089=CARTESIAN_POINT('Ctrl Pts',(-42.5661033314978,28.7931219150712,1.74111828938451E-15));
#12090=CARTESIAN_POINT('Ctrl Pts',(-42.5598087970384,28.776319278537,1.83186799063151E-15));
#12091=CARTESIAN_POINT('Ctrl Pts',(-42.554564129852,28.7623191587432,1.90748152224151E-15));
#12092=CARTESIAN_POINT('Ctrl Pts',(-42.5492048149782,28.7483606199135,-1.45408019805598E-15));
#12093=CARTESIAN_POINT('Ctrl Pts',(-42.5437340670539,28.7344492432458,-1.33226762955019E-15));
#12094=CARTESIAN_POINT('Ctrl Pts',(-42.5095094611057,28.6474206703273,-5.7021695305309E-16));
#12095=CARTESIAN_POINT('Ctrl Pts',(-42.4709064138711,28.5621802195229,1.68864321939785E-15));
#12096=CARTESIAN_POINT('Ctrl Pts',(-42.4282574113239,28.4789597631487,1.4432899320127E-15));
#12097=CARTESIAN_POINT('Ctrl Pts',(-42.3840281853581,28.3926558369106,1.18884585733067E-15));
#12098=CARTESIAN_POINT('Ctrl Pts',(-42.3354475000923,28.3085236412318,1.13314828784959E-16));
#12099=CARTESIAN_POINT('Ctrl Pts',(-42.2828302240828,28.2268253168789,-9.85322934354826E-16));
#12100=CARTESIAN_POINT('Ctrl Pts',(-42.2296353124201,28.1442301033568,-2.09602160961615E-15));
#12101=CARTESIAN_POINT('Ctrl Pts',(-42.1723142774313,28.0641216750719,-2.97253838087967E-16));
#12102=CARTESIAN_POINT('Ctrl Pts',(-42.1111408546837,27.9867862584352,-2.22044604925031E-16));
#12103=CARTESIAN_POINT('Ctrl Pts',(-42.0873237654165,27.9566767036837,-1.92762852498771E-16));
#12104=CARTESIAN_POINT('Ctrl Pts',(-42.062922203311,27.9269877214739,-2.27435711658574E-15));
#12105=CARTESIAN_POINT('Ctrl Pts',(-42.0379504574256,27.897737243879,-2.4980018054066E-15));
#12106=CARTESIAN_POINT('Ctrl Pts',(-42.0179637641745,27.8743259723636,-2.67700081545615E-15));
#12107=CARTESIAN_POINT('Ctrl Pts',(-41.9976117932189,27.8511956157283,-3.20009655856054E-15));
#12108=CARTESIAN_POINT('Ctrl Pts',(-41.9769014344167,27.8283557099806,-3.37230243729891E-15));
#12109=CARTESIAN_POINT('Ctrl Pts',(-41.9653531006681,27.8156199164157,-3.46832641158786E-15));
#12110=CARTESIAN_POINT('Ctrl Pts',(-41.9536984038099,27.8029800953511,7.67357186873025E-16));
#12111=CARTESIAN_POINT('Ctrl Pts',(-41.941943595762,27.7904426685355,6.38378239159465E-16));
#12112=CARTESIAN_POINT('Ctrl Pts',(-41.8728882149596,27.7167896765417,-1.19327910832526E-16));
#12113=CARTESIAN_POINT('Ctrl Pts',(-41.8003322451598,27.6466141188987,5.023733931277E-16));
#12114=CARTESIAN_POINT('Ctrl Pts',(-41.7245876255422,27.5802048475193,6.31439345255558E-16));
#12115=CARTESIAN_POINT('Ctrl Pts',(-41.6603367100057,27.5238727079194,7.40920462602983E-16));
#12116=CARTESIAN_POINT('Ctrl Pts',(-41.5937903710507,27.4702505403911,-6.6592528956053E-16));
#12117=CARTESIAN_POINT('Ctrl Pts',(-41.5251141439217,27.4195295723835,-9.0205620750794E-17));
#12118=CARTESIAN_POINT('Ctrl Pts',(-41.5024248047731,27.4027723145495,1.00001374685776E-16));
#12119=CARTESIAN_POINT('Ctrl Pts',(-41.4795028173951,27.3863318647826,3.04766671757009E-16));
#12120=CARTESIAN_POINT('Ctrl Pts',(-41.4563536803088,27.3702155597188,3.12250225675825E-16));
#12121=CARTESIAN_POINT('Ctrl Pts',(-41.4397590947421,27.3586624982632,3.17614852244211E-16));
#12122=CARTESIAN_POINT('Ctrl Pts',(-41.4230468122245,27.3472754851638,2.16855581531616E-16));
#12123=CARTESIAN_POINT('Ctrl Pts',(-41.4062334184353,27.3360667111883,1.87350135405495E-16));
#12124=CARTESIAN_POINT('Ctrl Pts',(-41.3198795578094,27.2784982679696,3.58096900660736E-17));
#12125=CARTESIAN_POINT('Ctrl Pts',(-41.2307763049236,27.2255680817869,1.44490008086718E-15));
#12126=CARTESIAN_POINT('Ctrl Pts',(-41.1392322045724,27.1775976168508,2.44942954807925E-15));
#12127=CARTESIAN_POINT('Ctrl Pts',(-41.0476881042212,27.1296271519147,3.45395901529133E-15));
#12128=CARTESIAN_POINT('Ctrl Pts',(-40.9537025110736,27.0866154975335,1.9880187375748E-15));
#12129=CARTESIAN_POINT('Ctrl Pts',(-40.8575459263663,27.0489248645033,3.05224595598119E-15));
#12130=CARTESIAN_POINT('Ctrl Pts',(-40.8369779594655,27.0408628093149,3.30417109938035E-15));
#12131=CARTESIAN_POINT('Ctrl Pts',(-40.8163105439644,27.0330443868027,6.92561079676203E-17));
#12132=CARTESIAN_POINT('Ctrl Pts',(-40.7955475841208,27.0254684201926,2.77555756156289E-17));
#12133=CARTESIAN_POINT('Ctrl Pts',(-42.5142224421888,30.0014129136195,9.11258330249199));
#12134=CARTESIAN_POINT('Ctrl Pts',(-42.5159017793566,30.3285506775319,9.09196520028265));
#12135=CARTESIAN_POINT('Ctrl Pts',(-42.4566447890085,30.6551053183166,9.07134709807331));
#12136=CARTESIAN_POINT('Ctrl Pts',(-42.3336250067878,30.9555494376831,9.05072899586397));
#12137=CARTESIAN_POINT('Ctrl Pts',(-42.0178238501021,31.7268123898897,8.99780075612207));
#12138=CARTESIAN_POINT('Ctrl Pts',(-41.2818335283954,32.3260101317949,8.94487251638018));
#12139=CARTESIAN_POINT('Ctrl Pts',(-40.4625634420876,32.4788845257636,8.89194427663829));
#12140=CARTESIAN_POINT('Ctrl Pts',(-39.6432933557798,32.6317589197323,8.83901603689639));
#12141=CARTESIAN_POINT('Ctrl Pts',(-38.7407435048708,32.3383099657646,8.7860877971545));
#12142=CARTESIAN_POINT('Ctrl Pts',(-38.1680406621116,31.7328516441468,8.7331595574126));
#12143=CARTESIAN_POINT('Ctrl Pts',(-37.5953378193524,31.127393322529,8.68023131767071));
#12144=CARTESIAN_POINT('Ctrl Pts',(-37.3524819847428,30.2099256332611,8.62730307792881));
#12145=CARTESIAN_POINT('Ctrl Pts',(-37.5506424000931,29.4004167679338,8.57437483818692));
#12146=CARTESIAN_POINT('Ctrl Pts',(-37.7488028154433,28.5909079026064,8.52144659844502));
#12147=CARTESIAN_POINT('Ctrl Pts',(-38.3879794807532,27.8893578612195,8.46851835870313));
#12148=CARTESIAN_POINT('Ctrl Pts',(-39.1755925591061,27.6168929096124,8.41559011896123));
#12149=CARTESIAN_POINT('Ctrl Pts',(-39.9632056374589,27.3444279580053,8.36266187921934));
#12150=CARTESIAN_POINT('Ctrl Pts',(-40.8992551288546,27.5010480961779,8.30973363947745));
#12151=CARTESIAN_POINT('Ctrl Pts',(-41.5552731103553,28.0150629869065,8.25680539973555));
#12152=CARTESIAN_POINT('Ctrl Pts',(-42.1511257187354,28.4819360331089,8.20873136732103));
#12153=CARTESIAN_POINT('Ctrl Pts',(-42.515956451978,29.2436544912819,8.16065733490651));
#12154=CARTESIAN_POINT('Ctrl Pts',(-42.5208028517601,30.0013273486611,8.11258330249199));
#12155=CARTESIAN_POINT('Origin',(40.,30.,12.2084234471775));
#12156=CARTESIAN_POINT('Ctrl Pts',(36.9237140680981,30.0022179367619,9.70842344717746));
#12157=CARTESIAN_POINT('Ctrl Pts',(36.922516753995,30.1470050693103,9.70090492237387));
#12158=CARTESIAN_POINT('Ctrl Pts',(36.9976393763497,31.3098392937669,9.64045815782839));
#12159=CARTESIAN_POINT('Ctrl Pts',(38.4808972548234,33.3003381457933,9.52708315354102));
#12160=CARTESIAN_POINT('Ctrl Pts',(41.9490301134684,33.0657006782122,9.36829843431533));
#12161=CARTESIAN_POINT('Ctrl Pts',(43.6328194606851,30.0249550147572,9.20951371508965));
#12162=CARTESIAN_POINT('Ctrl Pts',(41.990841947214,26.9611180881373,9.05072899586396));
#12163=CARTESIAN_POINT('Ctrl Pts',(38.5262718341427,26.6794501801396,8.89194427663828));
#12164=CARTESIAN_POINT('Ctrl Pts',(37.0061628405097,28.6614629298378,8.77784242707611));
#12165=CARTESIAN_POINT('Ctrl Pts',(36.9227278999928,29.8387134193989,8.71666881725584));
#12166=CARTESIAN_POINT('Ctrl Pts',(36.9240970871575,29.9975851957844,8.70842344717746));
#12167=CARTESIAN_POINT('Ctrl Pts',(36.9295987310864,29.9965353802945,9.79157655282255));
#12168=CARTESIAN_POINT('Ctrl Pts',(36.9349212372244,30.7003372070082,9.75519455573125));
#12169=CARTESIAN_POINT('Ctrl Pts',(37.5227892072477,32.4385323387372,9.66588431889804));
#12170=CARTESIAN_POINT('Ctrl Pts',(40.4091142878593,33.6090240981732,9.52364584232295));
#12171=CARTESIAN_POINT('Ctrl Pts',(43.2541895529164,31.6147492063695,9.36486112309727));
#12172=CARTESIAN_POINT('Ctrl Pts',(43.1213435063924,28.1406673653848,9.20607640387158));
#12173=CARTESIAN_POINT('Ctrl Pts',(40.1303404706603,26.3695397560852,9.0472916846459));
#12174=CARTESIAN_POINT('Ctrl Pts',(37.424156644603,27.7201137461279,8.90912506762955));
#12175=CARTESIAN_POINT('Ctrl Pts',(36.9337144820332,29.3758544021975,8.8238866903551));
#12176=CARTESIAN_POINT('Ctrl Pts',(36.9305016190507,30.0017249535699,8.79157655282255));
#12177=CARTESIAN_POINT('Ctrl Pts',(41.9134659966651,31.6359872033749,10.));
#12178=CARTESIAN_POINT('Ctrl Pts',(42.4575265280738,30.9996488965529,9.94707176025811));
#12179=CARTESIAN_POINT('Ctrl Pts',(42.8509942844496,29.1520113122851,9.84121528077432));
#12180=CARTESIAN_POINT('Ctrl Pts',(40.8305808300176,27.1407149884891,9.68243056154863));
#12181=CARTESIAN_POINT('Ctrl Pts',(38.0493533010215,27.7536486980057,9.52364584232295));
#12182=CARTESIAN_POINT('Ctrl Pts',(37.0541564147695,30.4198629586065,9.36486112309727));
#12183=CARTESIAN_POINT('Ctrl Pts',(38.7557048443201,32.703302841072,9.20607640387159));
#12184=CARTESIAN_POINT('Ctrl Pts',(41.596448124502,32.5111115852934,9.04729168464589));
#12185=CARTESIAN_POINT('Ctrl Pts',(42.9756378696192,30.0204406213279,8.88850696542022));
#12186=CARTESIAN_POINT('Ctrl Pts',(41.6306961451476,27.5108556326292,8.72972224619452));
#12187=CARTESIAN_POINT('Ctrl Pts',(38.7928711054024,27.2801418020177,8.57093752696886));
#12188=CARTESIAN_POINT('Ctrl Pts',(37.0601565987728,29.5393628566338,8.41215280774316));
#12189=CARTESIAN_POINT('Ctrl Pts',(38.0188181742894,32.220314819778,8.25336808851748));
#12190=CARTESIAN_POINT('Ctrl Pts',(40.7912199788668,32.8685926213582,8.0945833692918));
#12191=CARTESIAN_POINT('Ctrl Pts',(42.8392724649314,30.8907275834786,7.93579865006611));
#12192=CARTESIAN_POINT('Ctrl Pts',(42.2880181612085,28.0974129938986,7.77701393084043));
#12193=CARTESIAN_POINT('Ctrl Pts',(39.6421209022521,27.0458869626938,7.61822921161475));
#12194=CARTESIAN_POINT('Ctrl Pts',(37.3238561079106,28.698801824901,7.45944449238905));
#12195=CARTESIAN_POINT('Ctrl Pts',(37.4555568077712,31.5429425185067,7.30065977316339));
#12196=CARTESIAN_POINT('Ctrl Pts',(39.9166532336493,32.9745446259184,7.14187505393769));
#12197=CARTESIAN_POINT('Ctrl Pts',(42.45405223946,31.6830003648061,6.98309033471202));
#12198=CARTESIAN_POINT('Ctrl Pts',(42.7448069629157,28.8506970217256,6.82430561548633));
#12199=CARTESIAN_POINT('Ctrl Pts',(40.5227362518339,27.0705615946279,6.66552089626065));
#12200=CARTESIAN_POINT('Ctrl Pts',(37.8221091383592,27.9722786232342,6.50673617703496));
#12201=CARTESIAN_POINT('Ctrl Pts',(37.11530513124,30.7303410822086,6.34795145780927));
#12202=CARTESIAN_POINT('Ctrl Pts',(39.0493916239058,32.8197883419346,6.18916673858359));
#12203=CARTESIAN_POINT('Ctrl Pts',(41.8537443814859,32.3277659567929,6.03038201935791));
#12204=CARTESIAN_POINT('Ctrl Pts',(42.9610247802256,29.7047122902225,5.87159730013223));
#12205=CARTESIAN_POINT('Ctrl Pts',(41.3575359063571,27.3519896444331,5.71281258090654));
#12206=CARTESIAN_POINT('Ctrl Pts',(38.5112453356222,27.423476735993,5.55402786168086));
#12207=CARTESIAN_POINT('Ctrl Pts',(37.0278850671023,29.8537283137827,5.39524314245517));
#12208=CARTESIAN_POINT('Ctrl Pts',(38.2654469227344,32.4178892039655,5.2364584232295));
#12209=CARTESIAN_POINT('Ctrl Pts',(41.0909634671967,32.7685124695048,5.07767370400381));
#12210=CARTESIAN_POINT('Ctrl Pts',(42.9177209792689,30.5846083027713,4.91888898477813));
#12211=CARTESIAN_POINT('Ctrl Pts',(42.0733531331975,27.8655048921126,4.76010426555244));
#12212=CARTESIAN_POINT('Ctrl Pts',(39.3308647437863,27.1004964925952,4.60131954632676));
#12213=CARTESIAN_POINT('Ctrl Pts',(37.2009586278766,28.9899356566802,4.44253482710108));
#12214=CARTESIAN_POINT('Ctrl Pts',(37.6335286502452,31.8040720416137,4.28375010787539));
#12215=CARTESIAN_POINT('Ctrl Pts',(40.232564101165,32.9666102742903,4.12496538864971));
#12216=CARTESIAN_POINT('Ctrl Pts',(42.6186909591757,31.4132658067643,3.96618066942402));
#12217=CARTESIAN_POINT('Ctrl Pts',(42.6074495028282,28.5660998392996,3.80739595019834));
#12218=CARTESIAN_POINT('Ctrl Pts',(40.2091310993371,27.0316457817867,3.64861123097266));
#12219=CARTESIAN_POINT('Ctrl Pts',(37.6193566295732,28.2146709768635,3.48982651174698));
#12220=CARTESIAN_POINT('Ctrl Pts',(37.209021838156,31.0321353992193,3.33104179252129));
#12221=CARTESIAN_POINT('Ctrl Pts',(39.3537814511937,32.9046969160638,3.17225707329561));
#12222=CARTESIAN_POINT('Ctrl Pts',(42.0901434667156,32.1180563846122,3.01347235406992));
#12223=CARTESIAN_POINT('Ctrl Pts',(42.9130136738057,29.3923702313403,2.85468763484424));
#12224=CARTESIAN_POINT('Ctrl Pts',(41.0690679674053,27.2229590743015,2.69590291561856));
#12225=CARTESIAN_POINT('Ctrl Pts',(38.2464082284125,27.5958830490882,2.53711819639287));
#12226=CARTESIAN_POINT('Ctrl Pts',(37.0291327256062,30.1697363008652,2.37833347716719));
#12227=CARTESIAN_POINT('Ctrl Pts',(38.5316372616326,32.5881989279464,2.2195487579415));
#12228=CARTESIAN_POINT('Ctrl Pts',(41.3784033779123,32.6372078821259,2.06076403871582));
#12229=CARTESIAN_POINT('Ctrl Pts',(42.9632644723377,30.2718972026101,1.90197931949014));
#12230=CARTESIAN_POINT('Ctrl Pts',(41.8353048932223,27.6576678913952,1.74319460026445));
#12231=CARTESIAN_POINT('Ctrl Pts',(39.0271559993481,27.1878073976584,1.58440988103877));
#12232=CARTESIAN_POINT('Ctrl Pts',(37.1096257278314,29.2924578512643,1.42562516181309));
#12233=CARTESIAN_POINT('Ctrl Pts',(37.8381933254868,32.0448612920238,1.26684044258741));
#12234=CARTESIAN_POINT('Ctrl Pts',(40.5458433024136,32.9252083471976,1.10805572336172));
#12235=CARTESIAN_POINT('Ctrl Pts',(42.7538145542223,31.1276147393353,0.949271004136036));
#12236=CARTESIAN_POINT('Ctrl Pts',(42.4406505467311,28.2976300464195,0.790486284910354));
#12237=CARTESIAN_POINT('Ctrl Pts',(39.8932381788789,27.0262935717237,0.631701565684669));
#12238=CARTESIAN_POINT('Ctrl Pts',(37.4433110051919,28.4770232868416,0.472916846458986));
#12239=CARTESIAN_POINT('Ctrl Pts',(37.3344967579085,31.3226381965804,0.314132127233303));
#12240=CARTESIAN_POINT('Ctrl Pts',(39.6648948723936,32.9561497373541,0.155347408007618));
#12241=CARTESIAN_POINT('Ctrl Pts',(42.3041009889826,31.8858668894737,-0.00343731121806406));
#12242=CARTESIAN_POINT('Ctrl Pts',(42.8298459315877,29.0839076313313,-0.162222030443749));
#12243=CARTESIAN_POINT('Ctrl Pts',(41.4590097705807,27.7841423687619,-0.268078509927538));
#12244=CARTESIAN_POINT('Ctrl Pts',(40.6501999979751,27.5679131979649,-0.321006749669432));
#12245=CARTESIAN_POINT('Ctrl Pts',(42.0543315503421,31.7564253212268,10.1070022498898));
#12246=CARTESIAN_POINT('Ctrl Pts',(42.6384447339141,31.0732410562991,10.0540740101479));
#12247=CARTESIAN_POINT('Ctrl Pts',(43.0608788024441,29.0895840748975,9.94821753066413));
#12248=CARTESIAN_POINT('Ctrl Pts',(40.8917265356104,26.9302201236894,9.78943281143845));
#12249=CARTESIAN_POINT('Ctrl Pts',(37.9057505781308,27.5882767914968,9.63064809221276));
#12250=CARTESIAN_POINT('Ctrl Pts',(36.8372892802593,30.4507724329508,9.47186337298707));
#12251=CARTESIAN_POINT('Ctrl Pts',(38.6641023144879,32.9023146093124,9.3130786537614));
#12252=CARTESIAN_POINT('Ctrl Pts',(41.7139754541574,32.6959746162664,9.1542939345357));
#12253=CARTESIAN_POINT('Ctrl Pts',(43.1946983999746,30.0219454191376,8.99550921531004));
#12254=CARTESIAN_POINT('Ctrl Pts',(41.7507447458364,27.3276097844653,8.83672449608433));
#12255=CARTESIAN_POINT('Ctrl Pts',(38.7040046816492,27.0799112613917,8.67793977685867));
#12256=CARTESIAN_POINT('Ctrl Pts',(36.8437311858523,29.5054516680589,8.51915505763297));
#12257=CARTESIAN_POINT('Ctrl Pts',(37.8729675162166,32.3837699723495,8.3603703384073));
#12258=CARTESIAN_POINT('Ctrl Pts',(40.849468017033,33.0797726938475,8.2015856191816));
#12259=CARTESIAN_POINT('Ctrl Pts',(43.0482940459313,30.9563011732056,8.04280089995593));
#12260=CARTESIAN_POINT('Ctrl Pts',(42.4564574988625,27.9573483298281,7.88401618073024));
#12261=CARTESIAN_POINT('Ctrl Pts',(39.6157745562278,26.8284110476005,7.72523146150455));
#12262=CARTESIAN_POINT('Ctrl Pts',(37.1268437273741,28.6030102081707,7.56644674227888));
#12263=CARTESIAN_POINT('Ctrl Pts',(37.2682399703162,31.6565308720704,7.40766202305319));
#12264=CARTESIAN_POINT('Ctrl Pts',(39.9105174107972,33.193524673851,7.24887730382751));
#12265=CARTESIAN_POINT('Ctrl Pts',(42.6347146750959,31.8068994979186,7.09009258460182));
#12266=CARTESIAN_POINT('Ctrl Pts',(42.9468741819003,28.7660876267013,6.93130786537614));
#12267=CARTESIAN_POINT('Ctrl Pts',(40.5612190530281,26.854902176768,6.77252314615045));
#12268=CARTESIAN_POINT('Ctrl Pts',(37.6617771530468,27.8230018161528,6.61373842692477));
#12269=CARTESIAN_POINT('Ctrl Pts',(36.9029396433842,30.7841073373173,6.45495370769908));
#12270=CARTESIAN_POINT('Ctrl Pts',(38.9794097295519,33.0273755406259,6.29616898847341));
#12271=CARTESIAN_POINT('Ctrl Pts',(41.9902133488618,32.4991314479517,6.13738426924772));
#12272=CARTESIAN_POINT('Ctrl Pts',(43.1790095240595,29.6829737974538,5.97859955002203));
#12273=CARTESIAN_POINT('Ctrl Pts',(41.4574749945973,27.1570483987933,5.81981483079636));
#12274=CARTESIAN_POINT('Ctrl Pts',(38.4016461838984,27.2337982275802,5.66103011157067));
#12275=CARTESIAN_POINT('Ctrl Pts',(36.8090838883282,29.8429600837215,5.50224539234499));
#12276=CARTESIAN_POINT('Ctrl Pts',(38.1377525816606,32.595889388991,5.3434606731193));
#12277=CARTESIAN_POINT('Ctrl Pts',(41.1712780236696,32.972324840646,5.18467595389362));
#12278=CARTESIAN_POINT('Ctrl Pts',(43.1325177835687,30.6276460010621,5.02589123466794));
#12279=CARTESIAN_POINT('Ctrl Pts',(42.2259892592561,27.708367615716,4.86710651544225));
#12280=CARTESIAN_POINT('Ctrl Pts',(39.2816043396215,26.8870408222718,4.70832179621657));
#12281=CARTESIAN_POINT('Ctrl Pts',(36.9948987797599,28.915576732498,4.54953707699089));
#12282=CARTESIAN_POINT('Ctrl Pts',(37.4593137451855,31.9368842303111,4.3907523577652));
#12283=CARTESIAN_POINT('Ctrl Pts',(40.2496850068582,33.1850062110669,4.23196763853952));
#12284=CARTESIAN_POINT('Ctrl Pts',(42.8114737692787,31.5173076192186,4.07318291931383));
#12285=CARTESIAN_POINT('Ctrl Pts',(42.7994047393158,28.4605389668269,3.91439820008815));
#12286=CARTESIAN_POINT('Ctrl Pts',(40.2245269141311,26.8131214593336,3.75561348086246));
#12287=CARTESIAN_POINT('Ctrl Pts',(37.4440984085924,28.0832386118368,3.59682876163679));
#12288=CARTESIAN_POINT('Ctrl Pts',(37.0035555875124,31.1081191505555,3.4380440424111));
#12289=CARTESIAN_POINT('Ctrl Pts',(39.3062081293617,33.1185349147835,3.27925932318542));
#12290=CARTESIAN_POINT('Ctrl Pts',(42.2440156636693,32.2739834749591,3.12047460395973));
#12291=CARTESIAN_POINT('Ctrl Pts',(43.1274639356577,29.3476377386061,2.96168988473405));
#12292=CARTESIAN_POINT('Ctrl Pts',(41.147770620815,27.01851885521,2.80290516550837));
#12293=CARTESIAN_POINT('Ctrl Pts',(38.1173122966015,27.4188967498883,2.64412044628268));
#12294=CARTESIAN_POINT('Ctrl Pts',(36.810423396965,30.1822319490984,2.485335727057));
#12295=CARTESIAN_POINT('Ctrl Pts',(38.4235393228663,32.7787369754722,2.32655100783132));
#12296=CARTESIAN_POINT('Ctrl Pts',(41.4798786878256,32.8313538711974,2.16776628860563));
#12297=CARTESIAN_POINT('Ctrl Pts',(43.1814140978417,30.2919137328519,2.00898156937995));
#12298=CARTESIAN_POINT('Ctrl Pts',(41.970416382217,27.4852300691662,1.85019685015426));
#12299=CARTESIAN_POINT('Ctrl Pts',(38.9555371626234,26.9807793821798,1.69141213092858));
#12300=CARTESIAN_POINT('Ctrl Pts',(36.8968421336142,29.2403700082061,1.5326274117029));
#12301=CARTESIAN_POINT('Ctrl Pts',(37.6790454259794,32.1953999055115,1.37384269247722));
#12302=CARTESIAN_POINT('Ctrl Pts',(40.5860271986257,33.1405563566039,1.21505797325153));
#12303=CARTESIAN_POINT('Ctrl Pts',(42.9565448941293,31.2106274894275,1.05627325402585));
#12304=CARTESIAN_POINT('Ctrl Pts',(42.620326376454,28.1723049627795,0.897488534800165));
#12305=CARTESIAN_POINT('Ctrl Pts',(39.8853785863542,26.8073752302313,0.73870381557448));
#12306=CARTESIAN_POINT('Ctrl Pts',(37.2550926561533,28.3649047760814,0.579919096348797));
#12307=CARTESIAN_POINT('Ctrl Pts',(37.1382677208211,31.4200081849681,0.421134377123114));
#12308=CARTESIAN_POINT('Ctrl Pts',(39.6402251006691,33.1737755902464,0.262349657897428));
#12309=CARTESIAN_POINT('Ctrl Pts',(42.4737243123688,32.0247006518765,0.103564938671747));
#12310=CARTESIAN_POINT('Ctrl Pts',(43.0381735499873,29.0164667366633,-0.0552197805539385));
#12311=CARTESIAN_POINT('Ctrl Pts',(41.5664191624963,27.6210153455288,-0.161076260037727));
#12312=CARTESIAN_POINT('Ctrl Pts',(40.698066426161,27.3888678140614,-0.214004499779622));
#12313=CARTESIAN_POINT('Ctrl Pts',(42.1951971040191,31.8768634390787,10.2140044997796));
#12314=CARTESIAN_POINT('Ctrl Pts',(42.8193629397544,31.1468332160454,10.1610762600377));
#12315=CARTESIAN_POINT('Ctrl Pts',(43.2707633204387,29.02715683751,10.0552197805539));
#12316=CARTESIAN_POINT('Ctrl Pts',(40.9528722412032,26.7197252588896,9.89643506132826));
#12317=CARTESIAN_POINT('Ctrl Pts',(37.7621478552401,27.4229048849878,9.73765034210257));
#12318=CARTESIAN_POINT('Ctrl Pts',(36.6204221457491,30.4816819072951,9.57886562287689));
#12319=CARTESIAN_POINT('Ctrl Pts',(38.5724997846557,33.1013263775528,9.4200809036512));
#12320=CARTESIAN_POINT('Ctrl Pts',(41.8315027838129,32.8808376472393,9.26129618442552));
#12321=CARTESIAN_POINT('Ctrl Pts',(43.4137589303298,30.0234502169474,9.10251146519984));
#12322=CARTESIAN_POINT('Ctrl Pts',(41.8707933465252,27.1443639363013,8.94372674597414));
#12323=CARTESIAN_POINT('Ctrl Pts',(38.6151382578959,26.8796807207656,8.78494202674849));
#12324=CARTESIAN_POINT('Ctrl Pts',(36.6273057729317,29.4715404794841,8.62615730752277));
#12325=CARTESIAN_POINT('Ctrl Pts',(37.7271168581437,32.547225124921,8.46737258829711));
#12326=CARTESIAN_POINT('Ctrl Pts',(40.9077160551992,33.2909527663368,8.30858786907142));
#12327=CARTESIAN_POINT('Ctrl Pts',(43.2573156269313,31.0218747629328,8.14980314984574));
#12328=CARTESIAN_POINT('Ctrl Pts',(42.6248968365165,27.8172836657576,7.99101843062005));
#12329=CARTESIAN_POINT('Ctrl Pts',(39.5894282102036,26.6109351325072,7.83223371139437));
#12330=CARTESIAN_POINT('Ctrl Pts',(36.9298313468376,28.5072185914405,7.67344899216868));
#12331=CARTESIAN_POINT('Ctrl Pts',(37.0809231328611,31.7701192256341,7.514664272943));
#12332=CARTESIAN_POINT('Ctrl Pts',(39.904381587945,33.4125047217835,7.35587955371733));
#12333=CARTESIAN_POINT('Ctrl Pts',(42.8153771107317,31.9307986310311,7.19709483449163));
#12334=CARTESIAN_POINT('Ctrl Pts',(43.1489414008849,28.681478231677,7.03831011526596));
#12335=CARTESIAN_POINT('Ctrl Pts',(40.5997018542224,26.6392427589081,6.87952539604026));
#12336=CARTESIAN_POINT('Ctrl Pts',(37.5014451677344,27.6737250090714,6.72074067681458));
#12337=CARTESIAN_POINT('Ctrl Pts',(36.6905741555285,30.8378735924259,6.5619559575889));
#12338=CARTESIAN_POINT('Ctrl Pts',(38.9094278351979,33.2349627393171,6.40317123836321));
#12339=CARTESIAN_POINT('Ctrl Pts',(42.1266823162377,32.6704969391105,6.24438651913754));
#12340=CARTESIAN_POINT('Ctrl Pts',(43.3969942678934,29.6612353046849,6.08560179991184));
#12341=CARTESIAN_POINT('Ctrl Pts',(41.5574140828376,26.9621071531534,5.92681708068618));
#12342=CARTESIAN_POINT('Ctrl Pts',(38.2920470321746,27.0441197191674,5.76803236146047));
#12343=CARTESIAN_POINT('Ctrl Pts',(36.5902827095542,29.8321918536604,5.60924764223481));
#12344=CARTESIAN_POINT('Ctrl Pts',(38.0100582405868,32.7738895740165,5.45046292300911));
#12345=CARTESIAN_POINT('Ctrl Pts',(41.2515925801425,33.1761372117873,5.29167820378343));
#12346=CARTESIAN_POINT('Ctrl Pts',(43.3473145878683,30.6706836993528,5.13289348455775));
#12347=CARTESIAN_POINT('Ctrl Pts',(42.3786253853148,27.5512303393194,4.97410876533207));
#12348=CARTESIAN_POINT('Ctrl Pts',(39.2323439354566,26.6735851519484,4.81532404610638));
#12349=CARTESIAN_POINT('Ctrl Pts',(36.7888389316434,28.8412178083158,4.6565393268807));
#12350=CARTESIAN_POINT('Ctrl Pts',(37.2850988401258,32.0696964190085,4.49775460765501));
#12351=CARTESIAN_POINT('Ctrl Pts',(40.2668059125513,33.4034021478436,4.33896988842933));
#12352=CARTESIAN_POINT('Ctrl Pts',(43.0042565793815,31.6213494316729,4.18018516920364));
#12353=CARTESIAN_POINT('Ctrl Pts',(42.9913599758034,28.3549780943543,4.02140044997796));
#12354=CARTESIAN_POINT('Ctrl Pts',(40.2399227289251,26.5945971368806,3.86261573075228));
#12355=CARTESIAN_POINT('Ctrl Pts',(37.2688401876116,27.9518062468101,3.7038310115266));
#12356=CARTESIAN_POINT('Ctrl Pts',(36.7980893368689,31.1841029018916,3.54504629230091));
#12357=CARTESIAN_POINT('Ctrl Pts',(39.2586348075297,33.3323729135034,3.38626157307523));
#12358=CARTESIAN_POINT('Ctrl Pts',(42.3978878606232,32.4299105653059,3.22747685384954));
#12359=CARTESIAN_POINT('Ctrl Pts',(43.3419141975094,29.302905245872,3.06869213462386));
#12360=CARTESIAN_POINT('Ctrl Pts',(41.2264732742248,26.8140786361186,2.90990741539818));
#12361=CARTESIAN_POINT('Ctrl Pts',(37.9882163647905,27.2419104506884,2.75112269617249));
#12362=CARTESIAN_POINT('Ctrl Pts',(36.5917140683237,30.1947275973316,2.59233797694681));
#12363=CARTESIAN_POINT('Ctrl Pts',(38.3154413841,32.9692750229979,2.43355325772113));
#12364=CARTESIAN_POINT('Ctrl Pts',(41.5813539977387,33.0254998602688,2.27476853849544));
#12365=CARTESIAN_POINT('Ctrl Pts',(43.3995637233459,30.3119302630937,2.11598381926976));
#12366=CARTESIAN_POINT('Ctrl Pts',(42.1055278712115,27.3127922469373,1.95719910004408));
#12367=CARTESIAN_POINT('Ctrl Pts',(38.8839183258989,26.7737513667013,1.79841438081839));
#12368=CARTESIAN_POINT('Ctrl Pts',(36.6840585393969,29.1882821651479,1.63962966159271));
#12369=CARTESIAN_POINT('Ctrl Pts',(37.519897526472,32.3459385189991,1.48084494236703));
#12370=CARTESIAN_POINT('Ctrl Pts',(40.6262110948378,33.3559043660104,1.32206022314134));
#12371=CARTESIAN_POINT('Ctrl Pts',(43.1592752340363,31.2936402395195,1.16327550391566));
#12372=CARTESIAN_POINT('Ctrl Pts',(42.8000022061769,28.0469798791396,1.00449078468998));
#12373=CARTESIAN_POINT('Ctrl Pts',(39.8775189938294,26.5884568887389,0.84570606546429));
#12374=CARTESIAN_POINT('Ctrl Pts',(37.0668743071149,28.2527862653212,0.686921346238607));
#12375=CARTESIAN_POINT('Ctrl Pts',(36.9420386837336,31.5173781733559,0.528136627012925));
#12376=CARTESIAN_POINT('Ctrl Pts',(39.6155553289446,33.3914014431387,0.369351907787239));
#12377=CARTESIAN_POINT('Ctrl Pts',(42.643347635755,32.1635344142794,0.210567188561557));
#12378=CARTESIAN_POINT('Ctrl Pts',(43.2465011683868,28.9490258419954,0.0517824693358725));
#12379=CARTESIAN_POINT('Ctrl Pts',(41.6738285544119,27.4578883222956,-0.0540740101479163));
#12380=CARTESIAN_POINT('Ctrl Pts',(40.7459328543469,27.2098224301578,-0.107002249889811));
#12381=CARTESIAN_POINT('Ctrl Pts',(42.3360626576962,31.9973015569306,10.3210067496694));
#12382=CARTESIAN_POINT('Ctrl Pts',(43.0002811455947,31.2204253757916,10.2680785099275));
#12383=CARTESIAN_POINT('Ctrl Pts',(43.4806478384333,28.9647296001224,10.1622220304437));
#12384=CARTESIAN_POINT('Ctrl Pts',(41.0140179467961,26.5092303940899,10.0034373112181));
#12385=CARTESIAN_POINT('Ctrl Pts',(37.6185451323494,27.2575329784789,9.84465259199238));
#12386=CARTESIAN_POINT('Ctrl Pts',(36.4035550112389,30.5125913816394,9.6858678727667));
#12387=CARTESIAN_POINT('Ctrl Pts',(38.4808972548234,33.3003381457933,9.52708315354102));
#12388=CARTESIAN_POINT('Ctrl Pts',(41.9490301134684,33.0657006782122,9.36829843431533));
#12389=CARTESIAN_POINT('Ctrl Pts',(43.6328194606851,30.0249550147572,9.20951371508965));
#12390=CARTESIAN_POINT('Ctrl Pts',(41.990841947214,26.9611180881373,9.05072899586396));
#12391=CARTESIAN_POINT('Ctrl Pts',(38.5262718341427,26.6794501801396,8.89194427663828));
#12392=CARTESIAN_POINT('Ctrl Pts',(36.4108803600112,29.4376292909092,8.73315955741259));
#12393=CARTESIAN_POINT('Ctrl Pts',(37.5812662000709,32.7106802774926,8.57437483818692));
#12394=CARTESIAN_POINT('Ctrl Pts',(40.9659640933653,33.5021328388261,8.41559011896122));
#12395=CARTESIAN_POINT('Ctrl Pts',(43.4663372079312,31.0874483526599,8.25680539973555));
#12396=CARTESIAN_POINT('Ctrl Pts',(42.7933361741705,27.6772190016871,8.09802068050986));
#12397=CARTESIAN_POINT('Ctrl Pts',(39.5630818641794,26.3934592174139,7.93923596128418));
#12398=CARTESIAN_POINT('Ctrl Pts',(36.7328189663011,28.4114269747102,7.78045124205849));
#12399=CARTESIAN_POINT('Ctrl Pts',(36.8936062954061,31.8837075791978,7.62166652283282));
#12400=CARTESIAN_POINT('Ctrl Pts',(39.8982457650928,33.6314847697161,7.46288180360713));
#12401=CARTESIAN_POINT('Ctrl Pts',(42.9960395463676,32.0546977641436,7.30409708438144));
#12402=CARTESIAN_POINT('Ctrl Pts',(43.3510086198694,28.5968688366528,7.14531236515576));
#12403=CARTESIAN_POINT('Ctrl Pts',(40.6381846554167,26.4235833410482,6.98652764593007));
#12404=CARTESIAN_POINT('Ctrl Pts',(37.3411131824219,27.5244482019901,6.8277429267044));
#12405=CARTESIAN_POINT('Ctrl Pts',(36.4782086676728,30.8916398475345,6.66895820747871));
#12406=CARTESIAN_POINT('Ctrl Pts',(38.8394459408439,33.4425499380084,6.51017348825303));
#12407=CARTESIAN_POINT('Ctrl Pts',(42.2631512836135,32.8418624302693,6.35138876902734));
#12408=CARTESIAN_POINT('Ctrl Pts',(43.6149790117272,29.6394968119162,6.19260404980166));
#12409=CARTESIAN_POINT('Ctrl Pts',(41.657353171078,26.7671659075135,6.03381933057598));
#12410=CARTESIAN_POINT('Ctrl Pts',(38.1824478804507,26.8544412107546,5.87503461135029));
#12411=CARTESIAN_POINT('Ctrl Pts',(36.3714815307802,29.8214236235992,5.71624989212461));
#12412=CARTESIAN_POINT('Ctrl Pts',(37.882363899513,32.951889759042,5.55746517289893));
#12413=CARTESIAN_POINT('Ctrl Pts',(41.3319071366153,33.3799495829286,5.39868045367324));
#12414=CARTESIAN_POINT('Ctrl Pts',(43.562111392168,30.7137213976436,5.23989573444756));
#12415=CARTESIAN_POINT('Ctrl Pts',(42.5312615113734,27.3940930629228,5.08111101522188));
#12416=CARTESIAN_POINT('Ctrl Pts',(39.1830835312918,26.4601294816251,4.92232629599619));
#12417=CARTESIAN_POINT('Ctrl Pts',(36.5827790835267,28.7668588841336,4.7635415767705));
#12418=CARTESIAN_POINT('Ctrl Pts',(37.1108839350661,32.202508607706,4.60475685754482));
#12419=CARTESIAN_POINT('Ctrl Pts',(40.2839268182445,33.6217980846202,4.44597213831914));
#12420=CARTESIAN_POINT('Ctrl Pts',(43.1970393894843,31.7253912441272,4.28718741909346));
#12421=CARTESIAN_POINT('Ctrl Pts',(43.1833152122909,28.2494172218816,4.12840269986777));
#12422=CARTESIAN_POINT('Ctrl Pts',(40.255318543719,26.3760728144276,3.96961798064209));
#12423=CARTESIAN_POINT('Ctrl Pts',(37.0935819666309,27.8203738817834,3.8108332614164));
#12424=CARTESIAN_POINT('Ctrl Pts',(36.5926230862254,31.2600866532277,3.65204854219072));
#12425=CARTESIAN_POINT('Ctrl Pts',(39.2110614856976,33.5462109122232,3.49326382296504));
#12426=CARTESIAN_POINT('Ctrl Pts',(42.551760057577,32.5858376556528,3.33447910373935));
#12427=CARTESIAN_POINT('Ctrl Pts',(43.5563644593613,29.2581727531378,3.17569438451367));
#12428=CARTESIAN_POINT('Ctrl Pts',(41.3051759276346,26.6096384170271,3.01690966528799));
#12429=CARTESIAN_POINT('Ctrl Pts',(37.8591204329795,27.0649241514885,2.85812494606231));
#12430=CARTESIAN_POINT('Ctrl Pts',(36.3730047396825,30.2072232455647,2.69934022683662));
#12431=CARTESIAN_POINT('Ctrl Pts',(38.2073434453337,33.1598130705237,2.54055550761094));
#12432=CARTESIAN_POINT('Ctrl Pts',(41.6828293076519,33.2196458493402,2.38177078838525));
#12433=CARTESIAN_POINT('Ctrl Pts',(43.6177133488499,30.3319467933355,2.22298606915957));
#12434=CARTESIAN_POINT('Ctrl Pts',(42.2406393602062,27.1403544247083,2.06420134993389));
#12435=CARTESIAN_POINT('Ctrl Pts',(38.8122994891743,26.5667233512227,1.9054166307082));
#12436=CARTESIAN_POINT('Ctrl Pts',(36.4712749451797,29.1361943220897,1.74663191148252));
#12437=CARTESIAN_POINT('Ctrl Pts',(37.3607496269647,32.4964771324867,1.58784719225684));
#12438=CARTESIAN_POINT('Ctrl Pts',(40.6663949910499,33.5712523754168,1.42906247303115));
#12439=CARTESIAN_POINT('Ctrl Pts',(43.3620055739433,31.3766529896116,1.27027775380547));
#12440=CARTESIAN_POINT('Ctrl Pts',(42.9796780358998,27.9216547954996,1.11149303457979));
#12441=CARTESIAN_POINT('Ctrl Pts',(39.8696594013047,26.3695385472464,0.952708315354102));
#12442=CARTESIAN_POINT('Ctrl Pts',(36.8786559580763,28.1406677545611,0.793923596128418));
#12443=CARTESIAN_POINT('Ctrl Pts',(36.7458096466462,31.6147481617437,0.635138876902736));
#12444=CARTESIAN_POINT('Ctrl Pts',(39.5908855572201,33.609027296031,0.47635415767705));
#12445=CARTESIAN_POINT('Ctrl Pts',(42.8129709591412,32.3023681766822,0.317569438451369));
#12446=CARTESIAN_POINT('Ctrl Pts',(43.4548287867864,28.8815849473274,0.158784719225683));
#12447=CARTESIAN_POINT('Ctrl Pts',(41.7812379463276,27.2947612990625,0.0529282397418946));
#12448=CARTESIAN_POINT('Ctrl Pts',(40.7937992825328,27.0307770462543,0.));
#12449=CARTESIAN_POINT('Ctrl Pts',(40.7937992825328,27.0307770462543,0.));
#12450=CARTESIAN_POINT('Ctrl Pts',(40.8868532983231,27.0648166209,1.23206627813231E-16));
#12451=CARTESIAN_POINT('Ctrl Pts',(40.9778400910404,27.1036256541919,2.12059168736638E-15));
#12452=CARTESIAN_POINT('Ctrl Pts',(41.066551880518,27.1468754141207,1.88737914186277E-15));
#12453=CARTESIAN_POINT('Ctrl Pts',(41.1572334993246,27.1910855271895,1.64898815373364E-15));
#12454=CARTESIAN_POINT('Ctrl Pts',(41.2455386280921,27.239936384657,1.66196107955855E-15));
#12455=CARTESIAN_POINT('Ctrl Pts',(41.3312163993864,27.293122419604,1.66533453693773E-15));
#12456=CARTESIAN_POINT('Ctrl Pts',(41.4141658054003,27.3446147721763,1.6686005682734E-15));
#12457=CARTESIAN_POINT('Ctrl Pts',(41.4946528486676,27.4001714580703,-1.01232175488034E-15));
#12458=CARTESIAN_POINT('Ctrl Pts',(41.5724161625969,27.4595458715911,-7.21644966006352E-16));
#12459=CARTESIAN_POINT('Ctrl Pts',(41.640459062285,27.5114984834218,-4.67302775741614E-16));
#12460=CARTESIAN_POINT('Ctrl Pts',(41.7064163099332,27.5663747599262,-2.34369271321042E-15));
#12461=CARTESIAN_POINT('Ctrl Pts',(41.7700875460549,27.6240224703129,-3.10862446895044E-15));
#12462=CARTESIAN_POINT('Ctrl Pts',(41.7834301864647,27.6361028494133,-3.26891991751667E-15));
#12463=CARTESIAN_POINT('Ctrl Pts',(41.7966742105369,27.6483068338884,-2.63665242192149E-17));
#12464=CARTESIAN_POINT('Ctrl Pts',(41.8098005949636,27.6606167186647,-5.55111512312578E-17));
#12465=CARTESIAN_POINT('Ctrl Pts',(41.8822281775529,27.7285390929699,-2.1632275108547E-16));
#12466=CARTESIAN_POINT('Ctrl Pts',(41.9511900419254,27.799782684138,-1.11617369221794E-15));
#12467=CARTESIAN_POINT('Ctrl Pts',(42.016446845218,27.8740563163129,-1.02695629777827E-15));
#12468=CARTESIAN_POINT('Ctrl Pts',(42.0813423298977,27.9479187048411,-9.38232888694729E-16));
#12469=CARTESIAN_POINT('Ctrl Pts',(42.1425741539473,28.0247784714532,-1.19599204607943E-15));
#12470=CARTESIAN_POINT('Ctrl Pts',(42.1998633142192,28.1043759954772,-9.71445146547012E-16));
#12471=CARTESIAN_POINT('Ctrl Pts',(42.2557183977693,28.1819810141868,-7.52519161686897E-16));
#12472=CARTESIAN_POINT('Ctrl Pts',(42.3078260044473,28.2621891813364,1.94691714197589E-15));
#12473=CARTESIAN_POINT('Ctrl Pts',(42.3558807009596,28.3447740093935,2.58126853225349E-15));
#12474=CARTESIAN_POINT('Ctrl Pts',(42.3766082864569,28.3803955866496,2.85488534042471E-15));
#12475=CARTESIAN_POINT('Ctrl Pts',(42.3965812101076,28.4164594546924,1.497527271977E-15));
#12476=CARTESIAN_POINT('Ctrl Pts',(42.4157719782446,28.4529477707348,1.41553435639707E-15));
#12477=CARTESIAN_POINT('Ctrl Pts',(42.4294374159861,28.4789305145004,1.35714851821164E-15));
#12478=CARTESIAN_POINT('Ctrl Pts',(42.4427062131283,28.5051284836637,-1.16909168511305E-15));
#12479=CARTESIAN_POINT('Ctrl Pts',(42.4555678459356,28.5315352394017,-1.22124532708767E-15));
#12480=CARTESIAN_POINT('Ctrl Pts',(42.4611833798773,28.5430647267815,-1.24401619538084E-15));
#12481=CARTESIAN_POINT('Ctrl Pts',(42.4667203683547,28.5546322173608,-3.62400600888861E-15));
#12482=CARTESIAN_POINT('Ctrl Pts',(42.4721742413373,28.5662288988632,-3.58046925441613E-15));
#12483=CARTESIAN_POINT('Ctrl Pts',(42.5124020601376,28.6517661315138,-3.2593417408755E-15));
#12484=CARTESIAN_POINT('Ctrl Pts',(42.5481738402567,28.7390164875486,-2.58757764947659E-15));
#12485=CARTESIAN_POINT('Ctrl Pts',(42.579238603008,28.8277426426815,-2.27595720048157E-15));
#12486=CARTESIAN_POINT('Ctrl Pts',(42.6096166541956,28.914507434799,-1.9712253721258E-15));
#12487=CARTESIAN_POINT('Ctrl Pts',(42.6354937100697,29.0026841743411,-3.11366339761014E-15));
#12488=CARTESIAN_POINT('Ctrl Pts',(42.6565859526616,29.0920597462289,-2.4980018054066E-15));
#12489=CARTESIAN_POINT('Ctrl Pts',(42.6603145497727,29.1078591804377,-2.3891677625531E-15));
#12490=CARTESIAN_POINT('Ctrl Pts',(42.6638934918523,29.1236960859658,-2.40323005146812E-15));
#12491=CARTESIAN_POINT('Ctrl Pts',(42.6673210388351,29.1395692911278,-2.44249065417534E-15));
#12492=CARTESIAN_POINT('Ctrl Pts',(42.6874319440653,29.2327042725931,-2.69846234523205E-15));
#12493=CARTESIAN_POINT('Ctrl Pts',(42.7023348850078,29.3270899757285,5.17921855384608E-16));
#12494=CARTESIAN_POINT('Ctrl Pts',(42.7121083522879,29.4223175075911,1.0547118733939E-15));
#12495=CARTESIAN_POINT('Ctrl Pts',(42.7153862477415,29.4542555992424,1.23474435409905E-15));
#12496=CARTESIAN_POINT('Ctrl Pts',(42.7180867399261,29.4862882624031,5.37260594040857E-15));
#12497=CARTESIAN_POINT('Ctrl Pts',(42.720211565166,29.5183996018163,5.57887069874141E-15));
#12498=CARTESIAN_POINT('Ctrl Pts',(42.7214001886652,29.5363626285634,5.69425484149674E-15));
#12499=CARTESIAN_POINT('Ctrl Pts',(42.7224086601406,29.5543502699134,1.55024646972868E-15));
#12500=CARTESIAN_POINT('Ctrl Pts',(42.723237204183,29.5723596984032,1.47104550762833E-15));
#12501=CARTESIAN_POINT('Ctrl Pts',(42.7238114727046,29.5848421342712,1.41615087670374E-15));
#12502=CARTESIAN_POINT('Ctrl Pts',(42.7242991897067,29.5973335071231,2.07382757185176E-15));
#12503=CARTESIAN_POINT('Ctrl Pts',(42.7247003050432,29.6098233953396,1.9151347174784E-15));
#12504=CARTESIAN_POINT('Ctrl Pts',(42.7276931454214,29.7030141521449,7.31080309441068E-16));
#12505=CARTESIAN_POINT('Ctrl Pts',(42.7258764010177,29.7962693466217,3.12007103598847E-15));
#12506=CARTESIAN_POINT('Ctrl Pts',(42.7193891741356,29.8892138535835,2.55351295663786E-15));
#12507=CARTESIAN_POINT('Ctrl Pts',(42.7128889885514,29.98234402388,1.9858231367923E-15));
#12508=CARTESIAN_POINT('Ctrl Pts',(42.7016992591496,30.0751632458046,4.70096370999443E-15));
#12509=CARTESIAN_POINT('Ctrl Pts',(42.6859088780022,30.167282139709,4.42701431069281E-15));
#12510=CARTESIAN_POINT('Ctrl Pts',(42.6703416011653,30.2580994740049,4.15693557741601E-15));
#12511=CARTESIAN_POINT('Ctrl Pts',(42.6503022926889,30.3482369776061,1.17383405232967E-15));
#12512=CARTESIAN_POINT('Ctrl Pts',(42.6258330826424,30.4372963921836,1.0547118733939E-15));
#12513=CARTESIAN_POINT('Ctrl Pts',(42.6163194141826,30.4719228366785,1.00839697747183E-15));
#12514=CARTESIAN_POINT('Ctrl Pts',(42.6061356639453,30.5063859711879,9.2547699939467E-16));
#12515=CARTESIAN_POINT('Ctrl Pts',(42.5952827413713,30.5406609260158,7.49400541621981E-16));
#12516=CARTESIAN_POINT('Ctrl Pts',(42.58947852925,30.5589913901751,6.55233730470628E-16));
#12517=CARTESIAN_POINT('Ctrl Pts',(42.5834829076199,30.5772680160108,3.29288427622413E-15));
#12518=CARTESIAN_POINT('Ctrl Pts',(42.577295919888,30.5954868850076,3.24740234702858E-15));
#12519=CARTESIAN_POINT('Ctrl Pts',(42.571847351845,30.6115313240298,3.20734870595345E-15));
#12520=CARTESIAN_POINT('Ctrl Pts',(42.5662498919579,30.6275320443365,4.55710478188197E-15));
#12521=CARTESIAN_POINT('Ctrl Pts',(42.5605096912869,30.6434699599801,4.64905891561784E-15));
#12522=CARTESIAN_POINT('Ctrl Pts',(42.5280842400256,30.7335006290329,5.16849272161559E-15));
#12523=CARTESIAN_POINT('Ctrl Pts',(42.4910677443556,30.8216525646335,2.77315752414307E-15));
#12524=CARTESIAN_POINT('Ctrl Pts',(42.4495332377758,30.9074812017073,1.32532873564628E-15));
#12525=CARTESIAN_POINT('Ctrl Pts',(42.4183823578409,30.9718526795127,2.39457144273687E-16));
#12526=CARTESIAN_POINT('Ctrl Pts',(42.3846889484228,31.0349167649365,4.76029285454196E-15));
#12527=CARTESIAN_POINT('Ctrl Pts',(42.3484664521773,31.0964687502367,5.23192600354605E-15));
#12528=CARTESIAN_POINT('Ctrl Pts',(42.333534659064,31.1218419742131,5.42634464765648E-15));
#12529=CARTESIAN_POINT('Ctrl Pts',(42.3181729379481,31.1469580489284,6.86998275533235E-15));
#12530=CARTESIAN_POINT('Ctrl Pts',(42.3023815725951,31.1718017291815,6.78623823802127E-15));
#12531=CARTESIAN_POINT('Ctrl Pts',(42.2929489473471,31.1866415559078,6.73621528999162E-15));
#12532=CARTESIAN_POINT('Ctrl Pts',(42.2833677032904,31.2013767722444,5.84885791077277E-15));
#12533=CARTESIAN_POINT('Ctrl Pts',(42.2736398792402,31.2160020566235,5.75234304633909E-15));
#12534=CARTESIAN_POINT('Ctrl Pts',(42.2261111879894,31.2874590054872,5.28078587496221E-15));
#12535=CARTESIAN_POINT('Ctrl Pts',(42.175073702515,31.3563139832513,4.49466789804242E-15));
#12536=CARTESIAN_POINT('Ctrl Pts',(42.1205618043097,31.4222142805125,2.85188539450587E-15));
#12537=CARTESIAN_POINT('Ctrl Pts',(42.0689758173165,31.48457739736,1.29727879209382E-15));
#12538=CARTESIAN_POINT('Ctrl Pts',(42.0142778931532,31.5442947238755,-1.0060863342509E-15));
#12539=CARTESIAN_POINT('Ctrl Pts',(41.9564733781692,31.6010314766203,-2.0491421059976E-15));
#12540=CARTESIAN_POINT('Ctrl Pts',(41.9435074061502,31.6137579418236,-2.32930748699949E-15));
#12541=CARTESIAN_POINT('Ctrl Pts',(41.9303850442016,31.6263342844393,2.04314546332945E-17));
#12542=CARTESIAN_POINT('Ctrl Pts',(41.9171095224698,31.6387591744824,2.77555756156289E-17));
#12543=CARTESIAN_POINT('Ctrl Pts',(37.4805317771007,29.9980220368919,8.38741669750803));
#12544=CARTESIAN_POINT('Ctrl Pts',(37.4794102776092,29.8678903638642,8.39566206758641));
#12545=CARTESIAN_POINT('Ctrl Pts',(37.4886217757044,29.7379179497287,8.40390743766479));
#12546=CARTESIAN_POINT('Ctrl Pts',(37.5087192791305,29.6096513413884,8.41215280774317));
#12547=CARTESIAN_POINT('Ctrl Pts',(37.6377281009826,28.7862891717617,8.46508104748506));
#12548=CARTESIAN_POINT('Ctrl Pts',(38.2152996031925,28.0332154868897,8.51800928722696));
#12549=CARTESIAN_POINT('Ctrl Pts',(38.977056194255,27.6951309495556,8.57093752696885));
#12550=CARTESIAN_POINT('Ctrl Pts',(39.7388127853175,27.3570464122215,8.62386576671075));
#12551=CARTESIAN_POINT('Ctrl Pts',(40.6847544652325,27.4339510224254,8.67679400645264));
#12552=CARTESIAN_POINT('Ctrl Pts',(41.3818822592687,27.8906674923104,8.72972224619453));
#12553=CARTESIAN_POINT('Ctrl Pts',(42.0790100533048,28.3473839621954,8.78265048593643));
#12554=CARTESIAN_POINT('Ctrl Pts',(42.527323961462,29.1839122917617,8.83557872567833));
#12555=CARTESIAN_POINT('Ctrl Pts',(42.5216159580211,30.0172882838724,8.88850696542022));
#12556=CARTESIAN_POINT('Ctrl Pts',(42.5159079545802,30.8506642759831,8.94143520516211));
#12557=CARTESIAN_POINT('Ctrl Pts',(42.0561780395411,31.6808879306382,8.994363444904));
#12558=CARTESIAN_POINT('Ctrl Pts',(41.3528558686579,32.1280316339289,9.0472916846459));
#12559=CARTESIAN_POINT('Ctrl Pts',(40.6495336977747,32.5751753372196,9.10021992438779));
#12560=CARTESIAN_POINT('Ctrl Pts',(39.7026192710474,32.6392390891458,9.15314816412969));
#12561=CARTESIAN_POINT('Ctrl Pts',(38.9455706527587,32.2906976513646,9.20607640387159));
#12562=CARTESIAN_POINT('Ctrl Pts',(38.1885220344699,31.9421562135835,9.25900464361348));
#12563=CARTESIAN_POINT('Ctrl Pts',(37.6213392246197,31.181009586095,9.31193288335538));
#12564=CARTESIAN_POINT('Ctrl Pts',(37.5036139674033,30.3560672289173,9.36486112309727));
#12565=CARTESIAN_POINT('Ctrl Pts',(37.4868909425926,30.2388831018008,9.37237964790086));
#12566=CARTESIAN_POINT('Ctrl Pts',(37.4792373281869,30.1204116681271,9.37989817270444));
#12567=CARTESIAN_POINT('Ctrl Pts',(37.480218046669,30.0018167092234,9.38741669750803));
#12568=CARTESIAN_POINT('Ctrl Pts',(39.2062007174671,27.0307770462543,10.));
#12569=CARTESIAN_POINT('Ctrl Pts',(38.2187620536724,27.2947612990625,9.94707176025811));
#12570=CARTESIAN_POINT('Ctrl Pts',(36.5451697653868,28.8815756987713,9.84121528077432));
#12571=CARTESIAN_POINT('Ctrl Pts',(37.1870303021875,32.3023719893123,9.68243056154863));
#12572=CARTESIAN_POINT('Ctrl Pts',(40.4091142878593,33.6090240981732,9.52364584232295));
#12573=CARTESIAN_POINT('Ctrl Pts',(43.2541895529164,31.6147492063695,9.36486112309727));
#12574=CARTESIAN_POINT('Ctrl Pts',(43.1213435063924,28.1406673653848,9.20607640387158));
#12575=CARTESIAN_POINT('Ctrl Pts',(40.1303404706603,26.3695397560852,9.0472916846459));
#12576=CARTESIAN_POINT('Ctrl Pts',(37.0203226655434,27.9216549951598,8.88850696542021));
#12577=CARTESIAN_POINT('Ctrl Pts',(36.6379950966727,31.3766528296008,8.72972224619454));
#12578=CARTESIAN_POINT('Ctrl Pts',(39.3336051768584,33.5712515449036,8.57093752696884));
#12579=CARTESIAN_POINT('Ctrl Pts',(42.63924979695,32.4964766410994,8.41215280774317));
#12580=CARTESIAN_POINT('Ctrl Pts',(43.5287243142158,29.1361944846783,8.25336808851748));
#12581=CARTESIAN_POINT('Ctrl Pts',(41.1877002535156,26.5667240916348,8.0945833692918));
#12582=CARTESIAN_POINT('Ctrl Pts',(37.7593611185253,27.1403550261585,7.93579865006611));
#12583=CARTESIAN_POINT('Ctrl Pts',(36.3822874180148,30.3319467259865,7.77701393084044));
#12584=CARTESIAN_POINT('Ctrl Pts',(38.3171710506372,33.2196451638042,7.61822921161474));
#12585=CARTESIAN_POINT('Ctrl Pts',(41.7926561734374,33.159812400248,7.45944449238906));
#12586=CARTESIAN_POINT('Ctrl Pts',(43.6269944901785,30.207223201086,7.30065977316338));
#12587=CARTESIAN_POINT('Ctrl Pts',(42.1408791121553,27.0649247751536,7.14187505393769));
#12588=CARTESIAN_POINT('Ctrl Pts',(38.6948243496615,26.6096391370258,6.98309033471202));
#12589=CARTESIAN_POINT('Ctrl Pts',(36.4436362959865,29.2581729107715,6.82430561548632));
#12590=CARTESIAN_POINT('Ctrl Pts',(37.4482404844472,32.5858371063758,6.66552089626065));
#12591=CARTESIAN_POINT('Ctrl Pts',(40.7889383467181,33.5462101590121,6.50673617703496));
#12592=CARTESIAN_POINT('Ctrl Pts',(43.4073761900399,31.2600863855708,6.34795145780928));
#12593=CARTESIAN_POINT('Ctrl Pts',(42.9064174160314,27.8203743447495,6.1891667385836));
#12594=CARTESIAN_POINT('Ctrl Pts',(39.7446815105131,26.3760735841615,6.03038201935791));
#12595=CARTESIAN_POINT('Ctrl Pts',(36.816685463857,28.2494175937138,5.87159730013222));
#12596=CARTESIAN_POINT('Ctrl Pts',(36.8029612895799,31.7253908776466,5.71281258090655));
#12597=CARTESIAN_POINT('Ctrl Pts',(39.7160732420625,33.6217973153363,5.55402786168086));
#12598=CARTESIAN_POINT('Ctrl Pts',(42.8891154512744,32.2025081398842,5.39524314245518));
#12599=CARTESIAN_POINT('Ctrl Pts',(43.4172201906419,28.7668591460577,5.23645842322949));
#12600=CARTESIAN_POINT('Ctrl Pts',(40.8169162951919,26.4601302335076,5.07767370400381));
#12601=CARTESIAN_POINT('Ctrl Pts',(37.4687390262765,27.3940936164278,4.91888898477813));
#12602=CARTESIAN_POINT('Ctrl Pts',(36.4378893644385,30.7137212460463,4.76010426555244));
#12603=CARTESIAN_POINT('Ctrl Pts',(38.6680931462871,33.3799488650141,4.60131954632676));
#12604=CARTESIAN_POINT('Ctrl Pts',(42.1176356506926,32.9518891320487,4.44253482710108));
#12605=CARTESIAN_POINT('Ctrl Pts',(43.6285176985082,29.8214236615297,4.28375010787539));
#12606=CARTESIAN_POINT('Ctrl Pts',(41.8175517334939,26.8544418788833,4.1249653886497));
#12607=CARTESIAN_POINT('Ctrl Pts',(38.3426471809504,26.7671665941811,3.96618066942403));
#12608=CARTESIAN_POINT('Ctrl Pts',(36.3850217561086,29.639496888487,3.80739595019834));
#12609=CARTESIAN_POINT('Ctrl Pts',(37.7368491970887,32.8418618266495,3.64861123097266));
#12610=CARTESIAN_POINT('Ctrl Pts',(41.1605538126502,33.4425492067914,3.48982651174697));
#12611=CARTESIAN_POINT('Ctrl Pts',(43.5217905842841,30.8916396581577,3.33104179252129));
#12612=CARTESIAN_POINT('Ctrl Pts',(42.6588862528215,27.5244487277861,3.17225707329561));
#12613=CARTESIAN_POINT('Ctrl Pts',(39.3618154801332,26.4235841007334,3.01347235406992));
#12614=CARTESIAN_POINT('Ctrl Pts',(36.6489920919044,28.5968691346069,2.85468763484424));
#12615=CARTESIAN_POINT('Ctrl Pts',(37.0039610899898,32.0546973278633,2.69590291561856));
#12616=CARTESIAN_POINT('Ctrl Pts',(40.1017542133218,33.6314839980979,2.53711819639287));
#12617=CARTESIAN_POINT('Ctrl Pts',(43.1063930447263,31.883707179614,2.37833347716719));
#12618=CARTESIAN_POINT('Ctrl Pts',(43.2671803398556,28.4114273111418,2.21954875794151));
#12619=CARTESIAN_POINT('Ctrl Pts',(40.4369180427711,26.3934599853152,2.06076403871582));
#12620=CARTESIAN_POINT('Ctrl Pts',(37.2066644196549,27.6772194915737,1.90197931949014));
#12621=CARTESIAN_POINT('Ctrl Pts',(36.5336635272788,31.0874481281771,1.74319460026446));
#12622=CARTESIAN_POINT('Ctrl Pts',(39.0340361139851,33.5021320828999,1.58440988103877));
#12623=CARTESIAN_POINT('Ctrl Pts',(42.4187332816925,32.7106797239938,1.42562516181309));
#12624=CARTESIAN_POINT('Ctrl Pts',(43.5891188868934,29.4376293695436,1.2668404425874));
#12625=CARTESIAN_POINT('Ctrl Pts',(41.4737278337939,26.6794509596774,1.10805572336172));
#12626=CARTESIAN_POINT('Ctrl Pts',(38.0091585148051,26.9611185998674,0.949271004136034));
#12627=CARTESIAN_POINT('Ctrl Pts',(36.3671812304715,30.0249552475435,0.790486284910356));
#12628=CARTESIAN_POINT('Ctrl Pts',(38.0509704657541,33.0656996094815,0.631701565684668));
#12629=CARTESIAN_POINT('Ctrl Pts',(41.5191020833988,33.300338163167,0.472916846458987));
#12630=CARTESIAN_POINT('Ctrl Pts',(43.5964449208384,30.5125900673602,0.314132127233303));
#12631=CARTESIAN_POINT('Ctrl Pts',(42.3814529285809,27.2575355260863,0.155347408007619));
#12632=CARTESIAN_POINT('Ctrl Pts',(38.9859852522992,26.509227966563,-0.00343731121806271));
#12633=CARTESIAN_POINT('Ctrl Pts',(36.5193457296438,28.9647364017664,-0.162222030443748));
#12634=CARTESIAN_POINT('Ctrl Pts',(36.9997188544053,31.2204253757917,-0.268078509927537));
#12635=CARTESIAN_POINT('Ctrl Pts',(37.6639373423039,31.9973015569307,-0.321006749669432));
#12636=CARTESIAN_POINT('Ctrl Pts',(39.254067145653,27.2098224301579,10.1070022498898));
#12637=CARTESIAN_POINT('Ctrl Pts',(38.326171445588,27.4578883222957,10.0540740101479));
#12638=CARTESIAN_POINT('Ctrl Pts',(36.753497471091,28.9490171511311,9.94821753066412));
#12639=CARTESIAN_POINT('Ctrl Pts',(37.3566535495151,32.1635379970062,9.78943281143845));
#12640=CARTESIAN_POINT('Ctrl Pts',(40.3844445254766,33.391398438113,9.63064809221276));
#12641=CARTESIAN_POINT('Ctrl Pts',(43.0579605640956,31.5173791549904,9.47186337298707));
#12642=CARTESIAN_POINT('Ctrl Pts',(42.9331251896467,28.2527858996124,9.31307865376139));
#12643=CARTESIAN_POINT('Ctrl Pts',(40.1224808858561,26.5884580246842,9.15429393453571));
#12644=CARTESIAN_POINT('Ctrl Pts',(37.199998452969,28.0469800667601,8.99550921531002));
#12645=CARTESIAN_POINT('Ctrl Pts',(36.8407253961413,31.2936400891575,8.83672449608435));
#12646=CARTESIAN_POINT('Ctrl Pts',(39.3737890629457,33.3559035855774,8.67793977685866));
#12647=CARTESIAN_POINT('Ctrl Pts',(42.4801019321808,32.3459380572427,8.51915505763298));
#12648=CARTESIAN_POINT('Ctrl Pts',(43.3159407646573,29.1882823179323,8.36037033840729));
#12649=CARTESIAN_POINT('Ctrl Pts',(41.116081432307,26.7737520624662,8.20158561918161));
#12650=CARTESIAN_POINT('Ctrl Pts',(37.8944725786522,27.3127928121198,8.04280089995593));
#12651=CARTESIAN_POINT('Ctrl Pts',(36.6004369972767,30.3119301998059,7.88401618073024));
#12652=CARTESIAN_POINT('Ctrl Pts',(38.4186463389453,33.0254992160709,7.72523146150456));
#12653=CARTESIAN_POINT('Ctrl Pts',(41.6845582576594,32.9692743931401,7.56644674227887));
#12654=CARTESIAN_POINT('Ctrl Pts',(43.408285207977,30.194727555535,7.40766202305319));
#12655=CARTESIAN_POINT('Ctrl Pts',(42.0117832077729,27.2419110367462,7.24887730382751));
#12656=CARTESIAN_POINT('Ctrl Pts',(38.7735269863502,26.8140793127011,7.09009258460182));
#12657=CARTESIAN_POINT('Ctrl Pts',(36.6580865122905,29.3029053940003,6.93130786537614));
#12658=CARTESIAN_POINT('Ctrl Pts',(37.6021126487167,32.4299100491507,6.77252314615045));
#12659=CARTESIAN_POINT('Ctrl Pts',(40.7413650349914,33.3323722057112,6.61373842692478));
#12660=CARTESIAN_POINT('Ctrl Pts',(43.2019099830379,31.1841026503746,6.45495370769908));
#12661=CARTESIAN_POINT('Ctrl Pts',(42.7311592322764,27.9518066818591,6.29616898847341));
#12662=CARTESIAN_POINT('Ctrl Pts',(39.7600773220368,26.5945978601993,6.13738426924772));
#12663=CARTESIAN_POINT('Ctrl Pts',(37.0086406595725,28.3549784437647,5.97859955002205));
#12664=CARTESIAN_POINT('Ctrl Pts',(36.9957440587349,31.6213490872912,5.81981483079635));
#12665=CARTESIAN_POINT('Ctrl Pts',(39.7331941441191,33.4034014249478,5.66103011157068));
#12666=CARTESIAN_POINT('Ctrl Pts',(42.7149005832186,32.0696959793966,5.50224539234498));
#12667=CARTESIAN_POINT('Ctrl Pts',(43.2111603862932,28.8412180544458,5.34346067311931));
#12668=CARTESIAN_POINT('Ctrl Pts',(40.7676559014902,26.6735858584921,5.18467595389361));
#12669=CARTESIAN_POINT('Ctrl Pts',(37.6213751199146,27.5512308594478,5.02589123466794));
#12670=CARTESIAN_POINT('Ctrl Pts',(36.6526861231145,30.6706835568969,4.86710651544225));
#12671=CARTESIAN_POINT('Ctrl Pts',(38.7484076857008,33.1761365371633,4.70832179621658));
#12672=CARTESIAN_POINT('Ctrl Pts',(41.9899413367417,32.7738889848312,4.54953707699088));
#12673=CARTESIAN_POINT('Ctrl Pts',(43.4097165662084,29.8321918893037,4.39075235776521));
#12674=CARTESIAN_POINT('Ctrl Pts',(41.7079526050494,27.0441203470077,4.23196763853952));
#12675=CARTESIAN_POINT('Ctrl Pts',(38.4425862479632,26.9621077984146,4.07318291931383));
#12676=CARTESIAN_POINT('Ctrl Pts',(36.6030064536416,29.6612353766385,3.91439820008815));
#12677=CARTESIAN_POINT('Ctrl Pts',(37.873318135478,32.6704963718892,3.75561348086247));
#12678=CARTESIAN_POINT('Ctrl Pts',(41.0905719331606,33.2349620521929,3.59682876163679));
#12679=CARTESIAN_POINT('Ctrl Pts',(43.3094251415357,30.8378734144685,3.43804404241111));
#12680=CARTESIAN_POINT('Ctrl Pts',(42.498554301564,27.6737255031617,3.27925932318542));
#12681=CARTESIAN_POINT('Ctrl Pts',(39.4002982731538,26.6392434727839,3.12047460395974));
#12682=CARTESIAN_POINT('Ctrl Pts',(36.8510592679687,28.6814785116644,2.96168988473405));
#12683=CARTESIAN_POINT('Ctrl Pts',(37.1846234872531,31.9307982210587,2.80290516550837));
#12684=CARTESIAN_POINT('Ctrl Pts',(40.0956183917712,33.4125039966943,2.64412044628268));
#12685=CARTESIAN_POINT('Ctrl Pts',(42.9190762470616,31.7701188501454,2.485335727057));
#12686=CARTESIAN_POINT('Ctrl Pts',(43.0701680011581,28.5072189075851,2.32655100783132));
#12687=CARTESIAN_POINT('Ctrl Pts',(40.4105717023578,26.6109358541037,2.16776628860563));
#12688=CARTESIAN_POINT('Ctrl Pts',(37.3751037215009,27.8172841261039,2.00898156937995));
#12689=CARTESIAN_POINT('Ctrl Pts',(36.7426850639453,31.0218745519863,1.85019685015427));
#12690=CARTESIAN_POINT('Ctrl Pts',(39.092284139648,33.2909520559933,1.69141213092858));
#12691=CARTESIAN_POINT('Ctrl Pts',(42.2728826548695,32.5472246047984,1.5326274117029));
#12692=CARTESIAN_POINT('Ctrl Pts',(43.3726935193849,29.4715405533769,1.37384269247721));
#12693=CARTESIAN_POINT('Ctrl Pts',(41.3848614300641,26.879681453297,1.21505797325153));
#12694=CARTESIAN_POINT('Ctrl Pts',(38.129207087634,27.1443644171738,1.05627325402585));
#12695=CARTESIAN_POINT('Ctrl Pts',(36.5862417191497,30.0234504356966,0.897488534800165));
#12696=CARTESIAN_POINT('Ctrl Pts',(38.1684977604822,32.8808366429534,0.73870381557448));
#12697=CARTESIAN_POINT('Ctrl Pts',(41.4274995934721,33.1013263938789,0.579919096348797));
#12698=CARTESIAN_POINT('Ctrl Pts',(43.379577790424,30.4816806722675,0.421134377123115));
#12699=CARTESIAN_POINT('Ctrl Pts',(42.2378503226169,27.4229072789734,0.262349657897429));
#12700=CARTESIAN_POINT('Ctrl Pts',(39.0471307649853,26.7197229777436,0.103564938671748));
#12701=CARTESIAN_POINT('Ctrl Pts',(36.729230635486,29.027163229012,-0.0552197805539379));
#12702=CARTESIAN_POINT('Ctrl Pts',(37.1806370602456,31.1468332160454,-0.161076260037726));
#12703=CARTESIAN_POINT('Ctrl Pts',(37.8048028959809,31.8768634390788,-0.214004499779622));
#12704=CARTESIAN_POINT('Ctrl Pts',(39.301933573839,27.3888678140614,10.2140044997796));
#12705=CARTESIAN_POINT('Ctrl Pts',(38.4335808375037,27.6210153455288,10.1610762600377));
#12706=CARTESIAN_POINT('Ctrl Pts',(36.9618251767951,29.0164586034908,10.0552197805539));
#12707=CARTESIAN_POINT('Ctrl Pts',(37.5262767968427,32.0247040047002,9.89643506132825));
#12708=CARTESIAN_POINT('Ctrl Pts',(40.3597747630939,33.1737727780529,9.73765034210257));
#12709=CARTESIAN_POINT('Ctrl Pts',(42.8617315752749,31.4200091036112,9.57886562287689));
#12710=CARTESIAN_POINT('Ctrl Pts',(42.7449068729009,28.3649044338401,9.4200809036512));
#12711=CARTESIAN_POINT('Ctrl Pts',(40.1146213010519,26.8073762932831,9.26129618442552));
#12712=CARTESIAN_POINT('Ctrl Pts',(37.3796742403946,28.1723051383605,9.10251146519983));
#12713=CARTESIAN_POINT('Ctrl Pts',(37.0434556956098,31.2106273487141,8.94372674597416));
#12714=CARTESIAN_POINT('Ctrl Pts',(39.4139729490328,33.1405556262513,8.78494202674846));
#12715=CARTESIAN_POINT('Ctrl Pts',(42.3209540674116,32.1953994733859,8.62615730752279));
#12716=CARTESIAN_POINT('Ctrl Pts',(43.1031572150988,29.2403701511864,8.4673725882971));
#12717=CARTESIAN_POINT('Ctrl Pts',(41.0444626110982,26.9807800332976,8.30858786907142));
#12718=CARTESIAN_POINT('Ctrl Pts',(38.0295840387791,27.4852305980811,8.14980314984573));
#12719=CARTESIAN_POINT('Ctrl Pts',(36.8185865765384,30.2919136736252,7.99101843062005));
#12720=CARTESIAN_POINT('Ctrl Pts',(38.5201216272536,32.8313532683376,7.83223371139437));
#12721=CARTESIAN_POINT('Ctrl Pts',(41.5764603418814,32.7787363860323,7.67344899216869));
#12722=CARTESIAN_POINT('Ctrl Pts',(43.1895759257755,30.1822319099838,7.514664272943));
#12723=CARTESIAN_POINT('Ctrl Pts',(41.8826873033904,27.4188972983388,7.35587955371731));
#12724=CARTESIAN_POINT('Ctrl Pts',(38.8522296230389,27.0185194883763,7.19709483449164));
#12725=CARTESIAN_POINT('Ctrl Pts',(36.8725367285946,29.3476378772291,7.03831011526595));
#12726=CARTESIAN_POINT('Ctrl Pts',(37.7559848129862,32.2739829919254,6.87952539604026));
#12727=CARTESIAN_POINT('Ctrl Pts',(40.6937917232649,33.1185342524103,6.7207406768146));
#12728=CARTESIAN_POINT('Ctrl Pts',(42.9964437760359,31.1081189151782,6.56195595758889));
#12729=CARTESIAN_POINT('Ctrl Pts',(42.5559010485213,28.0832390189687,6.40317123836322));
#12730=CARTESIAN_POINT('Ctrl Pts',(39.7754731335606,26.813122136237,6.24438651913753));
#12731=CARTESIAN_POINT('Ctrl Pts',(37.2005958552881,28.4605392938157,6.08560179991186));
#12732=CARTESIAN_POINT('Ctrl Pts',(37.1885268278899,31.5173072969359,5.92681708068615));
#12733=CARTESIAN_POINT('Ctrl Pts',(39.7503150461758,33.1850055345593,5.7680323614605));
#12734=CARTESIAN_POINT('Ctrl Pts',(42.5406857151627,31.9368838189091,5.60924764223479));
#12735=CARTESIAN_POINT('Ctrl Pts',(43.0051005819446,28.9155769628338,5.45046292300913));
#12736=CARTESIAN_POINT('Ctrl Pts',(40.7183955077885,26.8870414834766,5.29167820378342));
#12737=CARTESIAN_POINT('Ctrl Pts',(37.7740112135527,27.7083681024678,5.13289348455775));
#12738=CARTESIAN_POINT('Ctrl Pts',(36.8674828817906,30.6276458677476,4.97410876533206));
#12739=CARTESIAN_POINT('Ctrl Pts',(38.8287222251146,32.9723242093125,4.81532404610638));
#12740=CARTESIAN_POINT('Ctrl Pts',(41.8622470227907,32.5958888376137,4.65653932688069));
#12741=CARTESIAN_POINT('Ctrl Pts',(43.1909154339085,29.8429601170776,4.49775460765501));
#12742=CARTESIAN_POINT('Ctrl Pts',(41.5983534766049,27.2337988151321,4.33896988842933));
#12743=CARTESIAN_POINT('Ctrl Pts',(38.542525314976,27.1570490026481,4.18018516920365));
#12744=CARTESIAN_POINT('Ctrl Pts',(36.8209911511747,29.6829738647901,4.02140044997796));
#12745=CARTESIAN_POINT('Ctrl Pts',(38.0097870738674,32.4991309171289,3.86261573075228));
#12746=CARTESIAN_POINT('Ctrl Pts',(41.020590053671,33.0273748975943,3.70383101152659));
#12747=CARTESIAN_POINT('Ctrl Pts',(43.0970596987873,30.7841071707794,3.54504629230091));
#12748=CARTESIAN_POINT('Ctrl Pts',(42.3382223503066,27.8230022785374,3.38626157307523));
#12749=CARTESIAN_POINT('Ctrl Pts',(39.4387810661743,26.8549028448345,3.22747685384954));
#12750=CARTESIAN_POINT('Ctrl Pts',(37.053126444033,28.7660878887219,3.06869213462386));
#12751=CARTESIAN_POINT('Ctrl Pts',(37.3652858845164,31.8068991142541,2.90990741539818));
#12752=CARTESIAN_POINT('Ctrl Pts',(40.0894825702206,33.1935239952906,2.75112269617249));
#12753=CARTESIAN_POINT('Ctrl Pts',(42.7317594493968,31.6565305206768,2.59233797694681));
#12754=CARTESIAN_POINT('Ctrl Pts',(42.8731556624607,28.6030105040283,2.43355325772113));
#12755=CARTESIAN_POINT('Ctrl Pts',(40.3842253619445,26.8284117228923,2.27476853849544));
#12756=CARTESIAN_POINT('Ctrl Pts',(37.543543023347,27.957348760634,2.11598381926976));
#12757=CARTESIAN_POINT('Ctrl Pts',(36.9517066006117,30.9563009757956,1.95719910004408));
#12758=CARTESIAN_POINT('Ctrl Pts',(39.1505321653109,33.0797720290867,1.79841438081839));
#12759=CARTESIAN_POINT('Ctrl Pts',(42.1270320280466,32.3837694856031,1.63962966159271));
#12760=CARTESIAN_POINT('Ctrl Pts',(43.1562681518763,29.50545173721,1.48084494236703));
#12761=CARTESIAN_POINT('Ctrl Pts',(41.2959950263345,27.0799119469166,1.32206022314134));
#12762=CARTESIAN_POINT('Ctrl Pts',(38.2492556604628,27.3276102344802,1.16327550391566));
#12763=CARTESIAN_POINT('Ctrl Pts',(36.805302207828,30.0219456238497,1.00449078468998));
#12764=CARTESIAN_POINT('Ctrl Pts',(38.2860250552103,32.6959736764254,0.845706065464291));
#12765=CARTESIAN_POINT('Ctrl Pts',(41.3358971035453,32.9023146245908,0.686921346238608));
#12766=CARTESIAN_POINT('Ctrl Pts',(43.1627106600096,30.4507712771748,0.528136627012925));
#12767=CARTESIAN_POINT('Ctrl Pts',(42.0942477166529,27.5882790318606,0.36935190778724));
#12768=CARTESIAN_POINT('Ctrl Pts',(39.1082762776713,26.9302179889242,0.210567188561559));
#12769=CARTESIAN_POINT('Ctrl Pts',(36.9391155413282,29.0895900562576,0.051782469335873));
#12770=CARTESIAN_POINT('Ctrl Pts',(37.3615552660859,31.0732410562992,-0.0540740101479155));
#12771=CARTESIAN_POINT('Ctrl Pts',(37.9456684496579,31.7564253212269,-0.107002249889811));
#12772=CARTESIAN_POINT('Ctrl Pts',(39.3498000020249,27.5679131979649,10.3210067496694));
#12773=CARTESIAN_POINT('Ctrl Pts',(38.5409902294193,27.784142368762,10.2680785099275));
#12774=CARTESIAN_POINT('Ctrl Pts',(37.1701528824992,29.0839000558506,10.1622220304438));
#12775=CARTESIAN_POINT('Ctrl Pts',(37.6959000441702,31.8858700123942,10.0034373112181));
#12776=CARTESIAN_POINT('Ctrl Pts',(40.3351050007111,32.9561471179928,9.84465259199238));
#12777=CARTESIAN_POINT('Ctrl Pts',(42.6655025864542,31.3226390522321,9.6858678727667));
#12778=CARTESIAN_POINT('Ctrl Pts',(42.5566885561551,28.4770229680677,9.52708315354102));
#12779=CARTESIAN_POINT('Ctrl Pts',(40.1067617162477,27.0262945618821,9.36829843431533));
#12780=CARTESIAN_POINT('Ctrl Pts',(37.5593500278202,28.2976302099609,9.20951371508965));
#12781=CARTESIAN_POINT('Ctrl Pts',(37.2461859950784,31.1276146082707,9.05072899586396));
#12782=CARTESIAN_POINT('Ctrl Pts',(39.45415683512,32.9252076669253,8.89194427663829));
#12783=CARTESIAN_POINT('Ctrl Pts',(42.1618062026424,32.0448608895291,8.73315955741259));
#12784=CARTESIAN_POINT('Ctrl Pts',(42.8903736655403,29.2924579844404,8.57437483818692));
#12785=CARTESIAN_POINT('Ctrl Pts',(40.9728437898896,27.187808004129,8.41559011896122));
#12786=CARTESIAN_POINT('Ctrl Pts',(38.164695498906,27.6576683840423,8.25680539973555));
#12787=CARTESIAN_POINT('Ctrl Pts',(37.0367361558003,30.2718971474446,8.09802068050986));
#12788=CARTESIAN_POINT('Ctrl Pts',(38.6215969155617,32.6372073206043,7.93923596128419));
#12789=CARTESIAN_POINT('Ctrl Pts',(41.4683624261034,32.5881983789245,7.78045124205849));
#12790=CARTESIAN_POINT('Ctrl Pts',(42.9708666435739,30.1697362644327,7.62166652283282));
#12791=CARTESIAN_POINT('Ctrl Pts',(41.753591399008,27.5958835599314,7.46288180360712));
#12792=CARTESIAN_POINT('Ctrl Pts',(38.9309322597276,27.2229596640516,7.30409708438145));
#12793=CARTESIAN_POINT('Ctrl Pts',(37.0869869448986,29.3923703604579,7.14531236515576));
#12794=CARTESIAN_POINT('Ctrl Pts',(37.9098569772558,32.1180559347003,6.98652764593008));
#12795=CARTESIAN_POINT('Ctrl Pts',(40.6462184115382,32.9046962991094,6.8277429267044));
#12796=CARTESIAN_POINT('Ctrl Pts',(42.7909775690338,31.032135179982,6.66895820747871));
#12797=CARTESIAN_POINT('Ctrl Pts',(42.3806428647663,28.2146713560783,6.51017348825303));
#12798=CARTESIAN_POINT('Ctrl Pts',(39.7908689450844,27.0316464122748,6.35138876902734));
#12799=CARTESIAN_POINT('Ctrl Pts',(37.3925510510037,28.5661001438667,6.19260404980166));
#12800=CARTESIAN_POINT('Ctrl Pts',(37.3813095970449,31.4132655065806,6.03381933057598));
#12801=CARTESIAN_POINT('Ctrl Pts',(39.7674359482324,32.9666096441708,5.87503461135029));
#12802=CARTESIAN_POINT('Ctrl Pts',(42.3664708471069,31.8040716584215,5.71624989212461));
#12803=CARTESIAN_POINT('Ctrl Pts',(42.7990407775959,28.9899358712219,5.55746517289892));
#12804=CARTESIAN_POINT('Ctrl Pts',(40.6691351140867,27.1004971084611,5.39868045367324));
#12805=CARTESIAN_POINT('Ctrl Pts',(37.9266473071909,27.8655053454879,5.23989573444756));
#12806=CARTESIAN_POINT('Ctrl Pts',(37.0822796404666,30.5846081785982,5.08111101522187));
#12807=CARTESIAN_POINT('Ctrl Pts',(38.9090367645283,32.7685118814618,4.9223262959962));
#12808=CARTESIAN_POINT('Ctrl Pts',(41.7345527088397,32.4178886903962,4.76354157677051));
#12809=CARTESIAN_POINT('Ctrl Pts',(42.9721143016087,29.8537283448515,4.60475685754483));
#12810=CARTESIAN_POINT('Ctrl Pts',(41.4887543481603,27.4234772832564,4.44597213831914));
#12811=CARTESIAN_POINT('Ctrl Pts',(38.6424643819888,27.3519902068817,4.28718741909346));
#12812=CARTESIAN_POINT('Ctrl Pts',(37.0389758487078,29.7047123529416,4.12840269986777));
#12813=CARTESIAN_POINT('Ctrl Pts',(38.1462560122567,32.3277654623687,3.9696179806421));
#12814=CARTESIAN_POINT('Ctrl Pts',(40.9506081741815,32.8197877429958,3.8108332614164));
#12815=CARTESIAN_POINT('Ctrl Pts',(42.8846942560388,30.7303409270902,3.65204854219072));
#12816=CARTESIAN_POINT('Ctrl Pts',(42.1778903990493,27.972279053913,3.49326382296504));
#12817=CARTESIAN_POINT('Ctrl Pts',(39.4772638591948,27.0705622168851,3.33447910373936));
#12818=CARTESIAN_POINT('Ctrl Pts',(37.2551936200974,28.8506972657794,3.17569438451367));
#12819=CARTESIAN_POINT('Ctrl Pts',(37.5459482817796,31.6830000074495,3.01690966528799));
#12820=CARTESIAN_POINT('Ctrl Pts',(40.0833467486701,32.974543993887,2.8581249460623));
#12821=CARTESIAN_POINT('Ctrl Pts',(42.5444426517321,31.5429421912082,2.69934022683662));
#12822=CARTESIAN_POINT('Ctrl Pts',(42.6761433237633,28.6988021004716,2.54055550761094));
#12823=CARTESIAN_POINT('Ctrl Pts',(40.3578790215312,27.0458875916808,2.38177078838525));
#12824=CARTESIAN_POINT('Ctrl Pts',(37.7119823251932,28.0974133951641,2.22298606915957));
#12825=CARTESIAN_POINT('Ctrl Pts',(37.1607281372782,30.8907273996049,2.06420134993389));
#12826=CARTESIAN_POINT('Ctrl Pts',(39.2087801909737,32.8685920021801,1.9054166307082));
#12827=CARTESIAN_POINT('Ctrl Pts',(41.9811814012236,32.2203143664078,1.74663191148252));
#12828=CARTESIAN_POINT('Ctrl Pts',(42.9398427843677,29.5393629210432,1.58784719225684));
#12829=CARTESIAN_POINT('Ctrl Pts',(41.2071286226048,27.2801424405362,1.42906247303115));
#12830=CARTESIAN_POINT('Ctrl Pts',(38.3693042332916,27.5108560517866,1.27027775380547));
#12831=CARTESIAN_POINT('Ctrl Pts',(37.0243626965063,30.0204408120029,1.11149303457979));
#12832=CARTESIAN_POINT('Ctrl Pts',(38.4035523499385,32.5111107098974,0.952708315354102));
#12833=CARTESIAN_POINT('Ctrl Pts',(41.2442946136185,32.7033028553028,0.793923596128417));
#12834=CARTESIAN_POINT('Ctrl Pts',(42.9458435295952,30.419861882082,0.635138876902737));
#12835=CARTESIAN_POINT('Ctrl Pts',(41.9506451106889,27.7536507847478,0.47635415767705));
#12836=CARTESIAN_POINT('Ctrl Pts',(39.1694217903574,27.1407130001049,0.31756943845137));
#12837=CARTESIAN_POINT('Ctrl Pts',(37.1490004471704,29.1520168835031,0.158784719225683));
#12838=CARTESIAN_POINT('Ctrl Pts',(37.5424734719262,30.999648896553,0.0529282397418953));
#12839=CARTESIAN_POINT('Ctrl Pts',(38.086534003335,31.635987203375,0.));
#12840=CARTESIAN_POINT('Ctrl Pts',(38.086534003335,31.635987203375,0.));
#12841=CARTESIAN_POINT('Ctrl Pts',(38.0249211977032,31.5780862952513,1.31416644246444E-16));
#12842=CARTESIAN_POINT('Ctrl Pts',(37.9666795658435,31.5170348772935,-1.65265760471522E-15));
#12843=CARTESIAN_POINT('Ctrl Pts',(37.9118059968576,31.4532177469288,-1.0547118733939E-15));
#12844=CARTESIAN_POINT('Ctrl Pts',(37.8554797506553,31.3877111749439,-4.40936624208665E-16));
#12845=CARTESIAN_POINT('Ctrl Pts',(37.8027018184566,31.3192900860968,7.34498374270318E-16));
#12846=CARTESIAN_POINT('Ctrl Pts',(37.7534943850504,31.248322100481,1.38777878078145E-15));
#12847=CARTESIAN_POINT('Ctrl Pts',(37.7025927286682,31.1749106711927,2.063551778308E-15));
#12848=CARTESIAN_POINT('Ctrl Pts',(37.6555110871616,31.0987734236319,-2.49260826547319E-16));
#12849=CARTESIAN_POINT('Ctrl Pts',(37.6123089458347,31.0202732787551,-1.66533453693773E-16));
#12850=CARTESIAN_POINT('Ctrl Pts',(37.5934080090042,30.9859294653715,-1.30340228070347E-16));
#12851=CARTESIAN_POINT('Ctrl Pts',(37.5752501267739,30.9511328723943,9.4717807460593E-16));
#12852=CARTESIAN_POINT('Ctrl Pts',(37.5578427256908,30.9159118020698,9.43689570931383E-16));
#12853=CARTESIAN_POINT('Ctrl Pts',(37.5483345257469,30.8966734920379,9.4178409461791E-16));
#12854=CARTESIAN_POINT('Ctrl Pts',(37.5390502604861,30.877308518724,3.47271198083739E-15));
#12855=CARTESIAN_POINT('Ctrl Pts',(37.529991343845,30.8578213657365,3.66373598126302E-15));
#12856=CARTESIAN_POINT('Ctrl Pts',(37.521341388929,30.8392139536738,3.84613626785524E-15));
#12857=CARTESIAN_POINT('Ctrl Pts',(37.5128944050193,30.8204891453965,3.43625081085264E-15));
#12858=CARTESIAN_POINT('Ctrl Pts',(37.5046657230374,30.8016836240999,3.49720252756924E-15));
#12859=CARTESIAN_POINT('Ctrl Pts',(37.4681048541193,30.7181287849921,3.76801718903391E-15));
#12860=CARTESIAN_POINT('Ctrl Pts',(37.4358042063432,30.6328904850717,1.83819694350877E-15));
#12861=CARTESIAN_POINT('Ctrl Pts',(37.4077880529032,30.5463675702544,1.60982338570648E-15));
#12862=CARTESIAN_POINT('Ctrl Pts',(37.3793096171943,30.4584169787416,1.37768153591975E-15));
#12863=CARTESIAN_POINT('Ctrl Pts',(37.3552577435286,30.3691382731478,2.54125228512118E-15));
#12864=CARTESIAN_POINT('Ctrl Pts',(37.3356970343403,30.2789132420247,2.63677968348475E-15));
#12865=CARTESIAN_POINT('Ctrl Pts',(37.316474608434,30.1902485643299,2.73065502917864E-15));
#12866=CARTESIAN_POINT('Ctrl Pts',(37.3015890909228,30.1006691003133,-1.19299483480687E-15));
#12867=CARTESIAN_POINT('Ctrl Pts',(37.2911444905801,30.01051432614,-1.11022302462516E-15));
#12868=CARTESIAN_POINT('Ctrl Pts',(37.2870143326577,29.9748639955796,-1.07749217458295E-15));
#12869=CARTESIAN_POINT('Ctrl Pts',(37.2835790912838,29.9391235236307,1.64690140981544E-15));
#12870=CARTESIAN_POINT('Ctrl Pts',(37.2808472267473,29.9033133666839,1.9151347174784E-15));
#12871=CARTESIAN_POINT('Ctrl Pts',(37.279230311654,29.8821183248032,2.07389459664214E-15));
#12872=CARTESIAN_POINT('Ctrl Pts',(37.2778598211019,29.8608988672751,1.32362561983342E-15));
#12873=CARTESIAN_POINT('Ctrl Pts',(37.2767377116473,29.8396592126925,1.47104550762833E-15));
#12874=CARTESIAN_POINT('Ctrl Pts',(37.2759907997416,29.8255214199689,1.56917289519332E-15));
#12875=CARTESIAN_POINT('Ctrl Pts',(37.2753540163908,29.8113746821749,-3.79292133871148E-15));
#12876=CARTESIAN_POINT('Ctrl Pts',(37.2748282896725,29.7972347995588,-3.58046925441613E-15));
#12877=CARTESIAN_POINT('Ctrl Pts',(37.271289501429,29.7020559763699,-2.15040509360744E-15));
#12878=CARTESIAN_POINT('Ctrl Pts',(37.2727694520664,29.6070261797158,5.94361540829616E-15));
#12879=CARTESIAN_POINT('Ctrl Pts',(37.2793267916415,29.5125441300592,5.02375918642883E-15));
#12880=CARTESIAN_POINT('Ctrl Pts',(37.2858616393742,29.4183861562479,4.10705809491485E-15));
#12881=CARTESIAN_POINT('Ctrl Pts',(37.2974387453601,29.3247712248665,1.93403274150591E-15));
#12882=CARTESIAN_POINT('Ctrl Pts',(37.3141641558389,29.2320760646995,2.44249065417534E-15));
#12883=CARTESIAN_POINT('Ctrl Pts',(37.3161010199708,29.2213416237625,2.50137195307623E-15));
#12884=CARTESIAN_POINT('Ctrl Pts',(37.3181069820462,29.2106195069702,5.84958917054875E-15));
#12885=CARTESIAN_POINT('Ctrl Pts',(37.3201822519865,29.199910292911,5.99520433297585E-15));
#12886=CARTESIAN_POINT('Ctrl Pts',(37.3377271674815,29.109371586578,7.22834140910308E-15));
#12887=CARTESIAN_POINT('Ctrl Pts',(37.3602214707246,29.0197547944519,4.68527759423326E-15));
#12888=CARTESIAN_POINT('Ctrl Pts',(37.3873898680817,28.9312978449583,4.08006961549745E-15));
#12889=CARTESIAN_POINT('Ctrl Pts',(37.3981381405763,28.8963027959425,3.84063921458696E-15));
#12890=CARTESIAN_POINT('Ctrl Pts',(37.4096185476567,28.8614893276667,2.28153659614193E-15));
#12891=CARTESIAN_POINT('Ctrl Pts',(37.4218162374507,28.8268725147577,2.41473507855972E-15));
#12892=CARTESIAN_POINT('Ctrl Pts',(37.427770307641,28.8099749761822,2.4797533834154E-15));
#12893=CARTESIAN_POINT('Ctrl Pts',(37.4338953041512,28.7931242992959,-2.54918434296526E-16));
#12894=CARTESIAN_POINT('Ctrl Pts',(37.4401896006146,28.7763222655356,-3.60822483003176E-16));
#12895=CARTESIAN_POINT('Ctrl Pts',(37.4454344715524,28.7623215747388,-4.49069528641816E-16));
#12896=CARTESIAN_POINT('Ctrl Pts',(37.4507940003222,28.7483624662939,-9.55594185352511E-17));
#12897=CARTESIAN_POINT('Ctrl Pts',(37.4562649710241,28.7344505244132,0.));
#12898=CARTESIAN_POINT('Ctrl Pts',(37.4904895705801,28.6474219757606,5.97788401973891E-16));
#12899=CARTESIAN_POINT('Ctrl Pts',(37.5290926132927,28.5621815406575,-1.01907588556041E-15));
#12900=CARTESIAN_POINT('Ctrl Pts',(37.5717416121145,28.4789610925679,-8.04911692853238E-16));
#12901=CARTESIAN_POINT('Ctrl Pts',(37.6159708476505,28.392657148709,-5.82812258299535E-16));
#12902=CARTESIAN_POINT('Ctrl Pts',(37.6645515459853,28.3085249287516,3.03185407248741E-15));
#12903=CARTESIAN_POINT('Ctrl Pts',(37.7171688370768,28.2268265748556,2.91433543964104E-15));
#12904=CARTESIAN_POINT('Ctrl Pts',(37.7703637738187,28.1442313162008,2.79552665814381E-15));
#12905=CARTESIAN_POINT('Ctrl Pts',(37.82768483747,28.0641228383192,1.3259987157817E-15));
#12906=CARTESIAN_POINT('Ctrl Pts',(37.8888582908095,27.9867873691188,1.52655665885959E-15));
#12907=CARTESIAN_POINT('Ctrl Pts',(37.9126752729538,27.9566779443845,1.60464093706217E-15));
#12908=CARTESIAN_POINT('Ctrl Pts',(37.9370767223879,27.9269890875379,2.09229451977724E-15));
#12909=CARTESIAN_POINT('Ctrl Pts',(37.9620483501692,27.8977387304677,2.35922392732846E-15));
#12910=CARTESIAN_POINT('Ctrl Pts',(37.9820324481196,27.8743304846818,2.57284009496863E-15));
#12911=CARTESIAN_POINT('Ctrl Pts',(38.0023817288993,27.8512030803908,8.27742804330915E-16));
#12912=CARTESIAN_POINT('Ctrl Pts',(38.0230893052639,27.8283660499001,9.85322934354826E-16));
#12913=CARTESIAN_POINT('Ctrl Pts',(38.0346401981847,27.8156273261991,1.07322270477195E-15));
#12914=CARTESIAN_POINT('Ctrl Pts',(38.0462975091725,27.8029846107706,4.1054544629886E-15));
#12915=CARTESIAN_POINT('Ctrl Pts',(38.0580549739782,27.7904443387168,4.08006961549745E-15));
#12916=CARTESIAN_POINT('Ctrl Pts',(38.1271103604421,27.7167912725716,3.93097621119732E-15));
#12917=CARTESIAN_POINT('Ctrl Pts',(38.1996663368624,27.6466156377666,4.44679118004536E-17));
#12918=CARTESIAN_POINT('Ctrl Pts',(38.2754109622693,27.5802062876346,1.93595139919012E-15));
#12919=CARTESIAN_POINT('Ctrl Pts',(38.3396619945932,27.5238739831441,3.54041859452371E-15));
#12920=CARTESIAN_POINT('Ctrl Pts',(38.4062084577275,27.4702516590102,4.21609339266478E-15));
#12921=CARTESIAN_POINT('Ctrl Pts',(38.474884814511,27.4195305445025,4.49640324973188E-15));
#12922=CARTESIAN_POINT('Ctrl Pts',(38.4975730150005,27.4027741108636,4.58900755395234E-15));
#12923=CARTESIAN_POINT('Ctrl Pts',(38.5204938400916,27.3863344534043,7.30713928788027E-15));
#12924=CARTESIAN_POINT('Ctrl Pts',(38.5436417920506,27.370218907676,7.78543896018391E-15));
#12925=CARTESIAN_POINT('Ctrl Pts',(38.5602378257786,27.358664790883,8.12835817427495E-15));
#12926=CARTESIAN_POINT('Ctrl Pts',(38.5769515782062,27.3472767508646,7.01631171217938E-15));
#12927=CARTESIAN_POINT('Ctrl Pts',(38.5937664597273,27.3360669813717,6.82093270754081E-15));
#12928=CARTESIAN_POINT('Ctrl Pts',(38.6801203856795,27.27849847555,5.81755102578388E-15));
#12929=CARTESIAN_POINT('Ctrl Pts',(38.7692237014379,27.2255682326337,2.2208055584883E-15));
#12930=CARTESIAN_POINT('Ctrl Pts',(38.8607678601949,27.1775977188098,1.64104840827406E-15));
#12931=CARTESIAN_POINT('Ctrl Pts',(38.9523120189519,27.1296272049858,1.06129125805982E-15));
#12932=CARTESIAN_POINT('Ctrl Pts',(39.0462976660425,27.0866155095581,-3.08948526585221E-15));
#12933=CARTESIAN_POINT('Ctrl Pts',(39.1424542982338,27.0489248453569,-3.74960479332387E-15));
#12934=CARTESIAN_POINT('Ctrl Pts',(39.1630222702032,27.0408627854955,-3.85678960606204E-15));
#12935=CARTESIAN_POINT('Ctrl Pts',(39.1836896904282,27.033044358642,-2.30566390043011E-15));
#12936=CARTESIAN_POINT('Ctrl Pts',(39.2044526546617,27.0254683880106,-2.24820162486594E-15));
#12937=CARTESIAN_POINT('Ctrl Pts',(37.4857777211518,30.0014129073083,9.11258330249198));
#12938=CARTESIAN_POINT('Ctrl Pts',(37.4840983822515,30.328550656152,9.09196520028264));
#12939=CARTESIAN_POINT('Ctrl Pts',(37.5433553669445,30.6551052822669,9.0713470980733));
#12940=CARTESIAN_POINT('Ctrl Pts',(37.6663751405423,30.9555493849948,9.05072899586396));
#12941=CARTESIAN_POINT('Ctrl Pts',(37.9821762750923,31.7268122944889,8.99780075612207));
#12942=CARTESIAN_POINT('Ctrl Pts',(38.7181665551061,32.3260099807071,8.94487251638018));
#12943=CARTESIAN_POINT('Ctrl Pts',(39.5374365897001,32.4788843609168,8.89194427663828));
#12944=CARTESIAN_POINT('Ctrl Pts',(40.3567066242941,32.6317587411266,8.83901603689639));
#12945=CARTESIAN_POINT('Ctrl Pts',(41.2592564134683,32.3383098153278,8.78608779715449));
#12946=CARTESIAN_POINT('Ctrl Pts',(41.8319592185383,31.7328515349137,8.73315955741259));
#12947=CARTESIAN_POINT('Ctrl Pts',(42.4046620236084,31.1273932544996,8.6802313176707));
#12948=CARTESIAN_POINT('Ctrl Pts',(42.6475178445743,30.20992561947,8.62730307792881));
#12949=CARTESIAN_POINT('Ctrl Pts',(42.4493574424489,29.4004168052366,8.57437483818691));
#12950=CARTESIAN_POINT('Ctrl Pts',(42.2511970403234,28.5909079910033,8.52144659844502));
#12951=CARTESIAN_POINT('Ctrl Pts',(41.6120204151065,27.8893579975662,8.46851835870312));
#12952=CARTESIAN_POINT('Ctrl Pts',(40.8244073873341,27.6168930641665,8.41559011896123));
#12953=CARTESIAN_POINT('Ctrl Pts',(40.0367943595617,27.3444281307668,8.36266187921933));
#12954=CARTESIAN_POINT('Ctrl Pts',(39.1007449292338,27.5010482574046,8.30973363947744));
#12955=CARTESIAN_POINT('Ctrl Pts',(38.444726990219,28.0150631146238,8.25680539973555));
#12956=CARTESIAN_POINT('Ctrl Pts',(37.8488744204282,28.4819361303902,8.20873136732103));
#12957=CARTESIAN_POINT('Ctrl Pts',(37.484043710445,29.2436545399986,8.1606573349065));
#12958=CARTESIAN_POINT('Ctrl Pts',(37.4791973108607,30.0013273487219,8.11258330249198));
#12959=CARTESIAN_POINT('Origin',(40.,-30.,5.));
#12960=CARTESIAN_POINT('Origin',(-40.,-30.,5.));
#12961=CARTESIAN_POINT('Origin',(-40.,30.,5.));
#12962=CARTESIAN_POINT('Origin',(40.,30.,5.));
#12963=CARTESIAN_POINT('Origin',(60.,50.,0.));
#12964=CARTESIAN_POINT('',(60.,50.,0.));
#12965=CARTESIAN_POINT('',(-60.,50.,0.));
#12966=CARTESIAN_POINT('',(60.,50.,0.));
#12967=CARTESIAN_POINT('',(-60.,50.,0.));
#12968=CARTESIAN_POINT('',(60.,50.,0.));
#12969=CARTESIAN_POINT('Origin',(60.,-50.,0.));
#12970=CARTESIAN_POINT('',(60.,-50.,0.));
#12971=CARTESIAN_POINT('',(60.,-50.,0.));
#12972=CARTESIAN_POINT('',(60.,-50.,0.));
#12973=CARTESIAN_POINT('Origin',(-60.,-50.,0.));
#12974=CARTESIAN_POINT('',(-60.,-50.,0.));
#12975=CARTESIAN_POINT('',(-60.,-50.,0.));
#12976=CARTESIAN_POINT('',(-60.,-50.,0.));
#12977=CARTESIAN_POINT('Origin',(-60.,50.,0.));
#12978=CARTESIAN_POINT('',(-60.,50.,0.));
#12979=CARTESIAN_POINT('Origin',(0.,0.,0.));
#13204=UNCERTAINTY_MEASURE_WITH_UNIT(LENGTH_MEASURE(0.01),#13232,
'DISTANCE_ACCURACY_VALUE',
'Maximum model space distance between geometric entities at asserted c
onnectivities');
#13213=UNCERTAINTY_MEASURE_WITH_UNIT(LENGTH_MEASURE(0.01),#13232,
'DISTANCE_ACCURACY_VALUE',
'Maximum model space distance between geometric entities at asserted c
onnectivities');
#13222=(
GEOMETRIC_REPRESENTATION_CONTEXT(3)
GLOBAL_UNCERTAINTY_ASSIGNED_CONTEXT((#13204))
GLOBAL_UNIT_ASSIGNED_CONTEXT((#13232,#13234,#13235))
REPRESENTATION_CONTEXT('','3D')
);
#13231=(
GEOMETRIC_REPRESENTATION_CONTEXT(3)
GLOBAL_UNCERTAINTY_ASSIGNED_CONTEXT((#13213))
GLOBAL_UNIT_ASSIGNED_CONTEXT((#13232,#13234,#13235))
REPRESENTATION_CONTEXT('','3D')
);
#13232=(
LENGTH_UNIT()
NAMED_UNIT(*)
SI_UNIT(.MILLI.,.METRE.)
);
#13234=(
NAMED_UNIT(*)
PLANE_ANGLE_UNIT()
SI_UNIT($,.RADIAN.)
);
#13235=(
NAMED_UNIT(*)
SI_UNIT($,.STERADIAN.)
SOLID_ANGLE_UNIT()
);
#13244=SHAPE_DEFINITION_REPRESENTATION(#13261,#13335);
#13261=PRODUCT_DEFINITION_SHAPE('',$,#13353);
#13335=SHAPE_REPRESENTATION('',(#4486),#13222);
#13344=PRODUCT_DEFINITION_CONTEXT('part definition',#13397,'design');
#13353=PRODUCT_DEFINITION('Carriage bridge plate',
'Carriage bridge plate',#13370,#13344);
#13370=PRODUCT_DEFINITION_FORMATION('',$,#13407);
#13397=APPLICATION_CONTEXT(
'Core Data for Automotive Mechanical Design Process');
#13398=PRODUCT_CONTEXT('part definition',#13397,'mechanical');
#13407=PRODUCT('Carriage bridge plate','Carriage bridge plate',$,(#13398));
#13417=PRESENTATION_STYLE_ASSIGNMENT((#13431));
#13431=SURFACE_STYLE_USAGE(.BOTH.,#13445);
#13445=SURFACE_SIDE_STYLE('',(#13459));
#13459=SURFACE_STYLE_FILL_AREA(#13473);
#13473=FILL_AREA_STYLE('Dark blue',(#13487));
#13487=FILL_AREA_STYLE_COLOUR('Dark blue',#13501);
#13501=COLOUR_RGB('Dark blue',0.0901960784313725,0.270588235294118,0.513725490196078);
ENDSEC;
END-ISO-10303-21;
